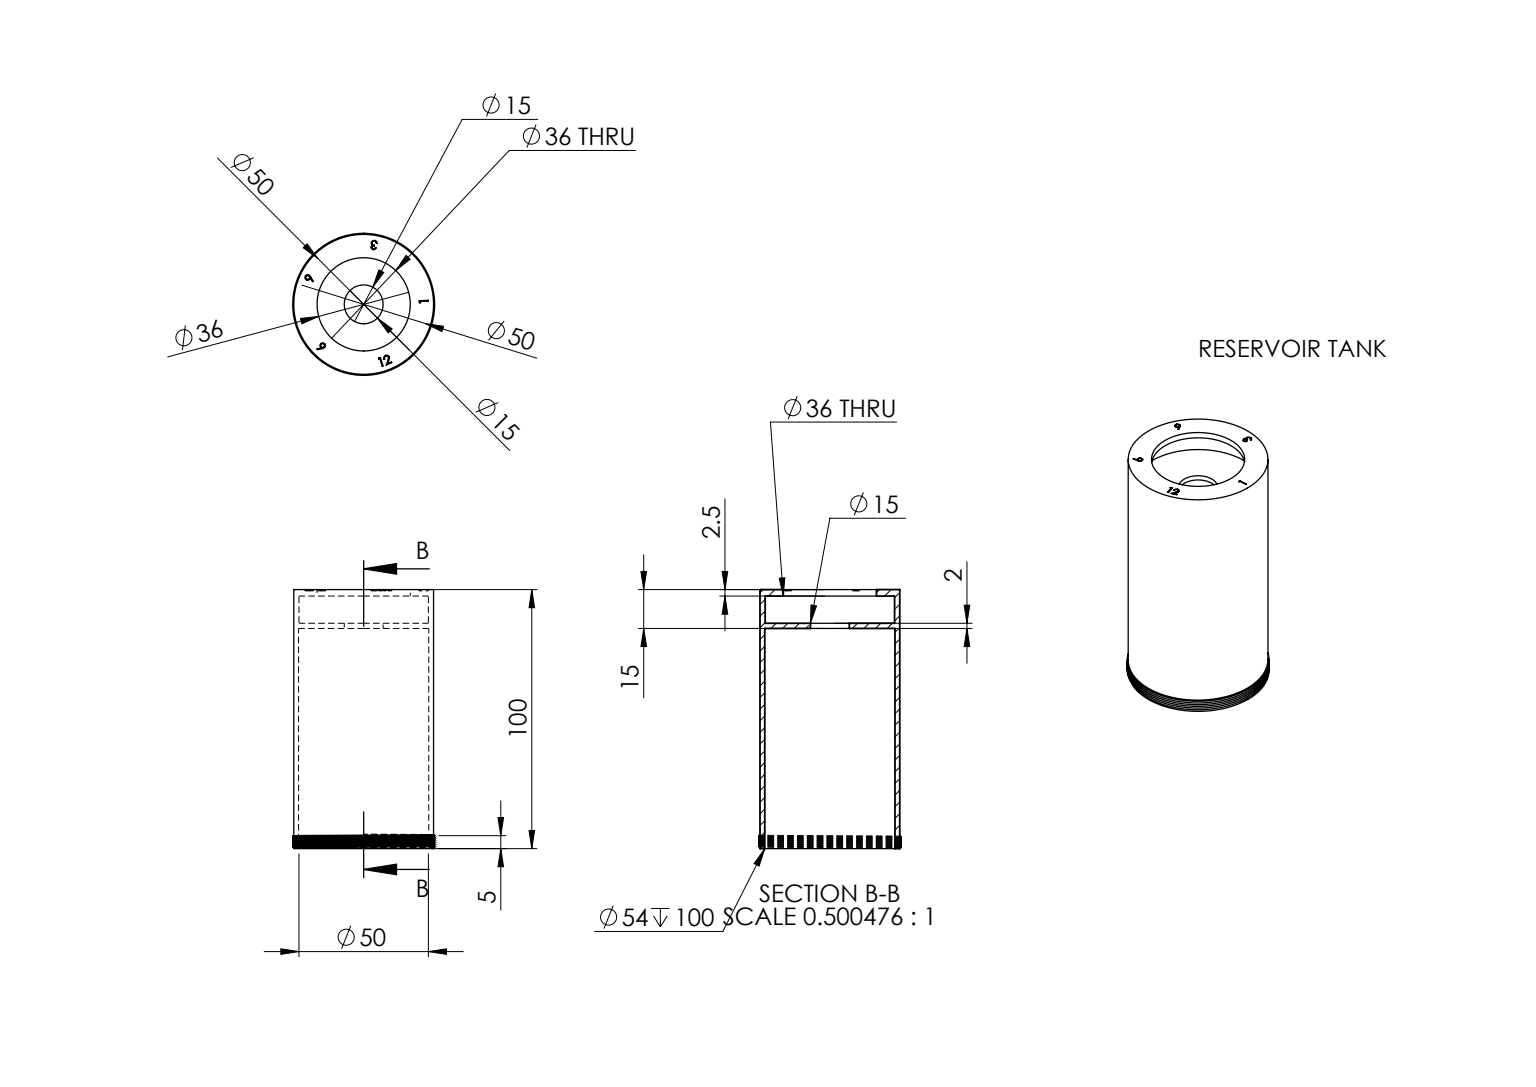
ISO-10303-21;
HEADER;
FILE_DESCRIPTION (('STEP AP214'),
    '1' );
FILE_NAME ('Reservoir Tank.step',
    '2026-10-24T15:06:47',
    ( '' ),
    ( '' ),
    'SwSTEP 2.0',
    'SolidWorks 2026',
    '' );
FILE_SCHEMA (( 'AUTOMOTIVE_DESIGN' ));
ENDSEC;

DATA;
#4=CARTESIAN_POINT ( 'NONE',  ( -22.08823018108446234, 99.50000000000000000, -9.406177930363766038 ) ) ;
#6=EDGE_LOOP ( 'NONE', ( #8139, #8496, #8983, #2392 ) ) ;
#8=CARTESIAN_POINT ( 'NONE',  ( 11.36312591709336850, 1.799999998907525267, 27.43301269999999903 ) ) ;
#9=EDGE_CURVE ( 'NONE', #2280, #2682, #6327, .T. ) ;
#12=ADVANCED_FACE ( 'NONE', ( #17 ), #758, .T. ) ;
#13=CARTESIAN_POINT ( 'NONE',  ( -27.00000000000001421, 4.450000000000000178, 11.18376618407356382 ) ) ;
#14=DIRECTION ( 'NONE',  ( 0.3918949146621865109, 0.000000000000000000, 0.9200099868272720860 ) ) ;
#15=CARTESIAN_POINT ( 'NONE',  ( -21.07742585509981126, 99.49999999999998579, -10.85999754779651383 ) ) ;
#17=FACE_OUTER_BOUND ( 'NONE', #3726, .T. ) ;
#18=CARTESIAN_POINT ( 'NONE',  ( -11.36312591709335962, 2.899999998907525356, -27.43301270000000258 ) ) ;
#19=CARTESIAN_POINT ( 'NONE',  ( 4.295198626299898237, 99.50000000000001421, -24.68029520312135361 ) ) ;
#23=CARTESIAN_POINT ( 'NONE',  ( -22.51767453479306980, 100.0000000000000000, -9.764155749770198511 ) ) ;
#29=CARTESIAN_POINT ( 'NONE',  ( -14.97509118869195888, 99.99999999999998579, 15.26515554624281101 ) ) ;
#35=CARTESIAN_POINT ( 'NONE',  ( -22.31230063665282515, 99.99999999999997158, -10.62159318200525249 ) ) ;
#36=DIRECTION ( 'NONE',  ( 0.000000000000000000, 1.000000000000000000, 0.000000000000000000 ) ) ;
#38=CARTESIAN_POINT ( 'NONE',  ( 27.00000000000000355, 2.999999997815050889, 0.000000000000000000 ) ) ;
#39=CARTESIAN_POINT ( 'NONE',  ( 19.39806930854667399, 3.449999998907525622, 19.39806930854668465 ) ) ;
#41=EDGE_LOOP ( 'NONE', ( #10357, #6514, #2134, #4776 ) ) ;
#43=CARTESIAN_POINT ( 'NONE',  ( 3.739209042966563867, 99.50000000000000000, -21.42288334414699236 ) ) ;
#45=CARTESIAN_POINT ( 'NONE',  ( 3.873456569393397331, 100.0000000000000284, -22.53291374702356364 ) ) ;
#47=CARTESIAN_POINT ( 'NONE',  ( -21.28703419482447146, 99.49999999999997158, -11.01737971290317297 ) ) ;
#48=CARTESIAN_POINT ( 'NONE',  ( 11.36312591709336139, 5.299999998907526155, -27.43301270000000258 ) ) ;
#51=CARTESIAN_POINT ( 'NONE',  ( -15.10382517959271098, 99.49999999999998579, 15.91526905993627317 ) ) ;
#52=DIRECTION ( 'NONE',  ( 0.4750403377899758972, 0.000000000000000000, -0.8799640205556052974 ) ) ;
#56=CARTESIAN_POINT ( 'NONE',  ( 9.910564025336874749, 100.0000000000000142, 20.75459158945058036 ) ) ;
#58=ADVANCED_FACE ( 'NONE', ( #3173 ), #2520, .T. ) ;
#61=CARTESIAN_POINT ( 'NONE',  ( 27.43301270000000258, 1.999999998907524779, -11.36312591709336139 ) ) ;
#63=CARTESIAN_POINT ( 'NONE',  ( 1.679787559701184688E-15, 5.249999998907525445, -27.43301270000000258 ) ) ;
#65=CARTESIAN_POINT ( 'NONE',  ( 11.18376618407356915, 4.950000000000000178, -27.00000000000000355 ) ) ;
#66=FACE_OUTER_BOUND ( 'NONE', #7305, .T. ) ;
#67=CARTESIAN_POINT ( 'NONE',  ( -16.33590634957226229, 99.50000000000000000, 16.80570853669505382 ) ) ;
#68=CARTESIAN_POINT ( 'NONE',  ( -20.91264567078791714, 99.99999999999994316, -10.54226115003387676 ) ) ;
#69=EDGE_CURVE ( 'NONE', #5685, #7937, #6333, .T. ) ;
#70=ORIENTED_EDGE ( 'NONE', *, *, #9652, .T. ) ;
#71=ORIENTED_EDGE ( 'NONE', *, *, #3469, .T. ) ;
#72=CARTESIAN_POINT ( 'NONE',  ( 3.551917533706515417, 100.0000000000000142, -21.11785906961830150 ) ) ;
#73=ORIENTED_EDGE ( 'NONE', *, *, #5083, .F. ) ;
#74=ADVANCED_FACE ( 'NONE', ( #2725 ), #8325, .T. ) ;
#75=CARTESIAN_POINT ( 'NONE',  ( 27.43301269999999548, 4.199999998907525622, 11.36312591709337916 ) ) ;
#76=FACE_OUTER_BOUND ( 'NONE', #1497, .T. ) ;
#81=CARTESIAN_POINT ( 'NONE',  ( -22.63784607493503387, 99.50000000000001421, -10.71517552924587058 ) ) ;
#85=EDGE_CURVE ( 'NONE', #5894, #5272, #1155, .T. ) ;
#86=CARTESIAN_POINT ( 'NONE',  ( 1.653273178848927064E-15, 2.399999997815050357, -27.00000000000000355 ) ) ;
#87=CARTESIAN_POINT ( 'NONE',  ( -20.71654887124055122, 99.50000000000001421, -9.874326132881018125 ) ) ;
#90=B_SPLINE_SURFACE_WITH_KNOTS ( 'NONE', 3, 1, ( 
 ( #3080, #5199 ),
 ( #8397, #1229 ),
 ( #4422, #5539 ),
 ( #1701, #10302 ),
 ( #3282, #3232 ),
 ( #4117, #7200 ),
 ( #3911, #924 ),
 ( #4848, #7097 ),
 ( #4064, #3134 ),
 ( #2291, #2443 ),
 ( #6321, #139 ) ),
 .UNSPECIFIED., .F., .F., .F.,
 ( 4, 1, 1, 1, 1, 1, 1, 1, 4 ),
 ( 2, 2 ),
 ( 0.000000000000000000, 0.09809051273808343241, 0.1997563395654988194, 0.3058527769869914259, 0.4162847437678430240, 0.5377099880548563693, 0.6743560419832976827, 0.8289895874771281425, 1.000000000000000000 ),
 ( 0.000000000000000000, 1.000000000000000000 ),
 .UNSPECIFIED. ) ;
#91=CARTESIAN_POINT ( 'NONE',  ( 3.058419780146050648, 99.50000000000000000, -23.12871267107006545 ) ) ;
#93=AXIS2_PLACEMENT_3D ( 'NONE', #4532, #670, #7729 ) ;
#94=CARTESIAN_POINT ( 'NONE',  ( -15.22320097062094568, 99.50000000000001421, 16.32303119091969634 ) ) ;
#96=CARTESIAN_POINT ( 'NONE',  ( 0.000000000000000000, 100.0000000000000000, 0.000000000000000000 ) ) ;
#97=CARTESIAN_POINT ( 'NONE',  ( 9.245739950628269810, 100.0000000000000284, 20.03726560014620617 ) ) ;
#100=VECTOR ( 'NONE', #6339, 1000.000000000000000 ) ;
#101=CARTESIAN_POINT ( 'NONE',  ( -20.89169796687544789, 100.0000000000000142, -10.40078880447404330 ) ) ;
#105=CARTESIAN_POINT ( 'NONE',  ( 27.43301269999999548, 5.099999998907525978, 11.36312591709337738 ) ) ;
#106=CARTESIAN_POINT ( 'NONE',  ( -15.19031985176477662, 99.49999999999998579, 15.56880617076518547 ) ) ;
#108=CARTESIAN_POINT ( 'NONE',  ( -15.37123125604856710, 99.50000000000001421, 16.48683530611566539 ) ) ;
#111=CARTESIAN_POINT ( 'NONE',  ( 3.970307086022987431, 99.50000000000001421, -24.36314111580913178 ) ) ;
#113=ORIENTED_EDGE ( 'NONE', *, *, #6148, .T. ) ;
#115=CARTESIAN_POINT ( 'NONE',  ( 27.43301270000000258, 1.149999998907525356, 0.000000000000000000 ) ) ;
#118=CARTESIAN_POINT ( 'NONE',  ( -27.43301270000000258, 0.6499999989075253559, -3.359575119402369376E-15 ) ) ;
#120=ORIENTED_EDGE ( 'NONE', *, *, #3091, .T. ) ;
#122=VECTOR ( 'NONE', #1890, 999.9999999999998863 ) ;
#123=CARTESIAN_POINT ( 'NONE',  ( 0.000000000000000000, 99.50000000000000000, 0.000000000000000000 ) ) ;
#124=FACE_OUTER_BOUND ( 'NONE', #10204, .T. ) ;
#128=CARTESIAN_POINT ( 'NONE',  ( 19.39806930854667399, 4.949999998907525622, 19.39806930854668465 ) ) ;
#129=CARTESIAN_POINT ( 'NONE',  ( 3.538198506519217190, 99.99999999999998579, -24.58220198924426114 ) ) ;
#131=CARTESIAN_POINT ( 'NONE',  ( -16.49419651247312046, 99.99999999999998579, 15.57134447358898477 ) ) ;
#132=CARTESIAN_POINT ( 'NONE',  ( -22.69253165798458127, 100.0000000000000142, -10.28928739654909563 ) ) ;
#133=CARTESIAN_POINT ( 'NONE',  ( 4.331079892889020400, 100.0000000000000000, -24.67336562508343079 ) ) ;
#136=ORIENTED_EDGE ( 'NONE', *, *, #3638, .F. ) ;
#137=ORIENTED_EDGE ( 'NONE', *, *, #6348, .F. ) ;
#139=CARTESIAN_POINT ( 'NONE',  ( -16.07368679829020763, 100.0000000000000000, 17.11560437002838952 ) ) ;
#140=CARTESIAN_POINT ( 'NONE',  ( -14.74935495356232984, 100.0000000000000142, 15.91322402822111926 ) ) ;
#142=ADVANCED_FACE ( 'NONE', ( #1039 ), #6680, .T. ) ;
#143=EDGE_CURVE ( 'NONE', #8324, #1908, #2115, .T. ) ;
#148=CARTESIAN_POINT ( 'NONE',  ( -19.09188309203678813, 4.500000000000000888, 19.09188309203678457 ) ) ;
#150=CARTESIAN_POINT ( 'NONE',  ( 3.411785164761435674, 99.50000000000000000, -22.76693382491622231 ) ) ;
#151=CARTESIAN_POINT ( 'NONE',  ( 3.750007936853901658, 99.99999999999998579, -22.95001988029826734 ) ) ;
#152=CARTESIAN_POINT ( 'NONE',  ( 7.856939908706818798, 99.50000000000001421, 20.19612520319305560 ) ) ;
#154=CARTESIAN_POINT ( 'NONE',  ( 27.43301270000000258, 4.349999998907525089, 0.000000000000000000 ) ) ;
#155=CARTESIAN_POINT ( 'NONE',  ( 26.99999999999999645, 3.150000000000000799, 11.18376618407358691 ) ) ;
#156=CARTESIAN_POINT ( 'NONE',  ( -21.24882413972086681, 100.0000000000000284, -9.742484589929601313 ) ) ;
#157=CARTESIAN_POINT ( 'NONE',  ( 3.717146347979291665, 99.50000000000000000, -21.42716062222556417 ) ) ;
#158=CARTESIAN_POINT ( 'NONE',  ( 3.681717055787076642, 99.50000000000000000, -21.09125273517263111 ) ) ;
#162=CARTESIAN_POINT ( 'NONE',  ( -16.01161620991261358, 99.50000000000000000, 17.10240122391520146 ) ) ;
#163=B_SPLINE_CURVE_WITH_KNOTS ( 'NONE', 3,
 ( #932, #5497, #832, #3193, #8885, #3093, #3922, #8786, #6277, #3240, #8737, #729, #9473, #2452, #4752 ),
 .UNSPECIFIED., .F., .F.,
 ( 4, 1, 1, 1, 1, 1, 1, 1, 1, 1, 1, 1, 4 ),
 ( 0.000000000000000000, 0.08490232564366416435, 0.1680779112633816463, 0.2506304657828534177, 0.3338427399641299420, 0.4169763759729993580, 0.4990117930239920674, 0.5811067191809071719, 0.6656374296971073745, 0.7500328835558887075, 0.8331455368193440014, 0.9159638734519762737, 1.000000000000000000 ),
 .UNSPECIFIED. ) ;
#164=CARTESIAN_POINT ( 'NONE',  ( 11.18376618407357626, 3.049999999999999822, 27.00000000000000000 ) ) ;
#165=CARTESIAN_POINT ( 'NONE',  ( 3.373335371007685435, 99.50000000000000000, -22.75111425220066863 ) ) ;
#168=CARTESIAN_POINT ( 'NONE',  ( -21.07742585509981126, 99.99999999999995737, -10.85999754779651383 ) ) ;
#169=ORIENTED_EDGE ( 'NONE', *, *, #6403, .F. ) ;
#174=CARTESIAN_POINT ( 'NONE',  ( 9.404665101723468368, 99.50000000000000000, 20.17141824467128686 ) ) ;
#175=CARTESIAN_POINT ( 'NONE',  ( -16.87593989452418697, 99.49999999999998579, 15.58794934546231126 ) ) ;
#176=CARTESIAN_POINT ( 'NONE',  ( 8.064245308217579122, 99.99999999999998579, 20.64099956338070641 ) ) ;
#179=ORIENTED_EDGE ( 'NONE', *, *, #6506, .T. ) ;
#180=ORIENTED_EDGE ( 'NONE', *, *, #3035, .T. ) ;
#182=CARTESIAN_POINT ( 'NONE',  ( -22.29247428061501779, 99.99999999999997158, -10.66603791136541624 ) ) ;
#183=CARTESIAN_POINT ( 'NONE',  ( 3.611424427577684781, 99.99999999999998579, -21.45475674085064099 ) ) ;
#184=EDGE_CURVE ( 'NONE', #533, #5989, #307, .T. ) ;
#185=CARTESIAN_POINT ( 'NONE',  ( -15.07178375341841381, 100.0000000000000000, 16.66969090848992607 ) ) ;
#187=ORIENTED_EDGE ( 'NONE', *, *, #7681, .T. ) ;
#188=DIRECTION ( 'NONE',  ( 0.000000000000000000, -1.000000000000000000, 0.000000000000000000 ) ) ;
#190=DIRECTION ( 'NONE',  ( -0.05422338932609765960, 0.000000000000000000, -0.9985288298541962204 ) ) ;
#194=ADVANCED_FACE ( 'NONE', ( #1864 ), #9727, .F. ) ;
#195=CARTESIAN_POINT ( 'NONE',  ( 3.302864939465488536, 99.50000000000001421, -22.83905924565489443 ) ) ;
#196=CARTESIAN_POINT ( 'NONE',  ( 3.891852272358404807, 99.99999999999998579, -22.89765557720719968 ) ) ;
#198=EDGE_LOOP ( 'NONE', ( #2371, #2144, #704, #4706 ) ) ;
#199=CARTESIAN_POINT ( 'NONE',  ( 3.207057600658871355, 100.0000000000000284, -22.07913334414698880 ) ) ;
#200=CARTESIAN_POINT ( 'NONE',  ( 27.00000000000000355, 2.999999997815050889, 0.000000000000000000 ) ) ;
#201=CARTESIAN_POINT ( 'NONE',  ( -20.71654887124055122, 100.0000000000000142, -9.874326132881018125 ) ) ;
#202=CARTESIAN_POINT ( 'NONE',  ( -21.66466628782423243, 100.0000000000000142, -9.640935998098070669 ) ) ;
#203=LINE ( 'NONE', #3388, #8398 ) ;
#205=LINE ( 'NONE', #1725, #6091 ) ;
#207=ORIENTED_EDGE ( 'NONE', *, *, #9006, .F. ) ;
#209=FACE_OUTER_BOUND ( 'NONE', #3870, .T. ) ;
#210=CARTESIAN_POINT ( 'NONE',  ( 9.806436918512124734, 99.99999999999998579, 20.18080982695387604 ) ) ;
#212=CARTESIAN_POINT ( 'NONE',  ( -27.43301270000000258, 2.199999998907525622, -11.36312591709336317 ) ) ;
#214=DIRECTION ( 'NONE',  ( -0.000000000000000000, 1.000000000000000000, -0.000000000000000000 ) ) ;
#215=CARTESIAN_POINT ( 'NONE',  ( 8.429066232339796017, 100.0000000000000000, 19.67794530653910101 ) ) ;
#216=CARTESIAN_POINT ( 'NONE',  ( 1.653273178848927064E-15, 2.399999997815050357, -27.00000000000000355 ) ) ;
#217=ORIENTED_EDGE ( 'NONE', *, *, #7917, .F. ) ;
#218=CARTESIAN_POINT ( 'NONE',  ( -20.89052720883767122, 99.50000000000000000, -9.602653601535816819 ) ) ;
#219=CARTESIAN_POINT ( 'NONE',  ( 11.36312591709336139, 5.199999998907525622, -27.43301270000000258 ) ) ;
#220=CARTESIAN_POINT ( 'NONE',  ( -16.18965924272485779, 99.49999999999998579, 15.26525457555968224 ) ) ;
#221=FACE_OUTER_BOUND ( 'NONE', #8631, .T. ) ;
#223=CARTESIAN_POINT ( 'NONE',  ( 26.99999999999999645, 1.550000000000000266, 11.18376618407358691 ) ) ;
#224=VERTEX_POINT ( 'NONE', #1816 ) ;
#225=CARTESIAN_POINT ( 'NONE',  ( 5.240996349771887886, 100.0000000000000142, -23.60769396873743631 ) ) ;
#226=ORIENTED_EDGE ( 'NONE', *, *, #3625, .T. ) ;
#227=EDGE_CURVE ( 'NONE', #6767, #4694, #1090, .T. ) ;
#231=LINE ( 'NONE', #3414, #2289 ) ;
#232=LINE ( 'NONE', #8144, #5785 ) ;
#233=CARTESIAN_POINT ( 'NONE',  ( -22.11394672483139701, 99.50000000000000000, -10.91855052283267646 ) ) ;
#235=CARTESIAN_POINT ( 'NONE',  ( -15.26676860252058887, 99.99999999999998579, 16.38168943497750973 ) ) ;
#236=VECTOR ( 'NONE', #2101, 1000.000000000000000 ) ;
#237=EDGE_CURVE ( 'NONE', #1790, #7639, #6949, .T. ) ;
#240=CARTESIAN_POINT ( 'NONE',  ( 0.000000000000000000, 97.50000000000000000, 18.00000000000000000 ) ) ;
#242=CARTESIAN_POINT ( 'NONE',  ( 3.058419780146050648, 99.50000000000000000, -23.12871267107006545 ) ) ;
#243=LINE ( 'NONE', #5946, #5211 ) ;
#244=CARTESIAN_POINT ( 'NONE',  ( 3.701176614148623756, 99.50000000000000000, -24.64875008328975170 ) ) ;
#245=CARTESIAN_POINT ( 'NONE',  ( 7.734522023158566739, 99.50000000000002842, 20.86022014488863618 ) ) ;
#248=CARTESIAN_POINT ( 'NONE',  ( 1.653273178848927064E-15, 4.799999997815051600, -27.00000000000000355 ) ) ;
#249=CARTESIAN_POINT ( 'NONE',  ( -21.00001322343447541, 99.50000000000001421, -9.990026185521596602 ) ) ;
#250=CARTESIAN_POINT ( 'NONE',  ( 3.635130212803377781, 100.0000000000000000, -23.00575896550913768 ) ) ;
#251=CARTESIAN_POINT ( 'NONE',  ( -21.72555844818415594, 99.50000000000001421, -11.09629251537910655 ) ) ;
#252=CARTESIAN_POINT ( 'NONE',  ( 4.906732565843439531, 100.0000000000000142, -23.57187248890526376 ) ) ;
#255=B_SPLINE_CURVE_WITH_KNOTS ( 'NONE', 3,
 ( #43, #4128, #5748, #6482, #981, #3244, #8984, #8105, #7258, #4950, #7354, #5651, #9812, #9671, #7311 ),
 .UNSPECIFIED., .F., .F.,
 ( 4, 1, 1, 1, 1, 1, 1, 1, 1, 1, 1, 1, 4 ),
 ( 0.000000000000000000, 0.1166921615859537187, 0.2277195327244859735, 0.3361971884410420164, 0.4453256767247914527, 0.5018483577356800396, 0.5617326728321133666, 0.6243107931132723110, 0.6909729641497043273, 0.7615676753376537933, 0.8363829297815326136, 0.9156607463298391814, 0.9999999999999998890 ),
 .UNSPECIFIED. ) ;
#258=CARTESIAN_POINT ( 'NONE',  ( -15.03963071504896121, 100.0000000000000000, 16.63526396357264758 ) ) ;
#261=CARTESIAN_POINT ( 'NONE',  ( 27.43301270000000258, 1.849999998907525534, 0.000000000000000000 ) ) ;
#264=CARTESIAN_POINT ( 'NONE',  ( -20.64578974631102426, 99.99999999999995737, -10.10077944494247504 ) ) ;
#265=DIRECTION ( 'NONE',  ( -0.000000000000000000, 1.000000000000000000, -0.000000000000000000 ) ) ;
#266=CARTESIAN_POINT ( 'NONE',  ( 8.322475189980043098, 100.0000000000000142, 19.72675386960232657 ) ) ;
#267=ORIENTED_EDGE ( 'NONE', *, *, #2370, .F. ) ;
#268=CARTESIAN_POINT ( 'NONE',  ( -21.30033281797529909, 99.50000000000002842, -9.345151174687854834 ) ) ;
#269=CARTESIAN_POINT ( 'NONE',  ( 4.135809822336132591, 99.99999999999998579, -24.70305975188825443 ) ) ;
#271=CARTESIAN_POINT ( 'NONE',  ( 3.775125937424839151, 100.0000000000000000, -21.41825520325024712 ) ) ;
#272=CARTESIAN_POINT ( 'NONE',  ( 8.829292973371666520, 99.49999999999998579, 19.92220432019063736 ) ) ;
#278=ORIENTED_EDGE ( 'NONE', *, *, #3961, .T. ) ;
#279=VECTOR ( 'NONE', #5092, 1000.000000000000000 ) ;
#281=CARTESIAN_POINT ( 'NONE',  ( 6.246869686064662197, 99.50000000000000000, 20.92172973853146090 ) ) ;
#282=CARTESIAN_POINT ( 'NONE',  ( 1.653273178848927064E-15, 4.799999997815051600, -27.00000000000000355 ) ) ;
#285=CARTESIAN_POINT ( 'NONE',  ( 8.081885929396888102, 99.50000000000001421, 20.89785832093561169 ) ) ;
#286=CARTESIAN_POINT ( 'NONE',  ( 2.852289972453743161, 99.50000000000000000, -22.14293542748032451 ) ) ;
#288=CARTESIAN_POINT ( 'NONE',  ( 3.735769352376668184, 99.49999999999998579, -24.30643046864489420 ) ) ;
#292=CARTESIAN_POINT ( 'NONE',  ( -27.43301270000000258, 3.949999998907525178, -3.359575119402369376E-15 ) ) ;
#294=EDGE_CURVE ( 'NONE', #8788, #5320, #3852, .T. ) ;
#296=DIRECTION ( 'NONE',  ( -0.000000000000000000, -1.000000000000000000, -0.000000000000000000 ) ) ;
#297=CARTESIAN_POINT ( 'NONE',  ( 7.771508748547515388, 99.50000000000001421, 20.40818475981234315 ) ) ;
#298=ORIENTED_EDGE ( 'NONE', *, *, #7410, .F. ) ;
#299=CARTESIAN_POINT ( 'NONE',  ( 9.902568905804752575, 99.49999999999998579, 20.48863403721516363 ) ) ;
#300=CARTESIAN_POINT ( 'NONE',  ( -11.18376618407356560, 3.249999997815050001, -27.00000000000000355 ) ) ;
#301=CARTESIAN_POINT ( 'NONE',  ( -21.16695614262292580, 99.50000000000000000, -11.33496398805607441 ) ) ;
#304=CARTESIAN_POINT ( 'NONE',  ( -21.44539290152690114, 100.0000000000000000, -11.08070480119962298 ) ) ;
#306=PLANE ( 'NONE',  #2619 ) ;
#307=LINE ( 'NONE', #5759, #1112 ) ;
#313=CARTESIAN_POINT ( 'NONE',  ( -11.36312591709335962, 2.099999998907525089, -27.43301270000000258 ) ) ;
#314=CARTESIAN_POINT ( 'NONE',  ( -11.18376618407358336, 0.5500000000000000444, 26.99999999999999645 ) ) ;
#315=CARTESIAN_POINT ( 'NONE',  ( 7.826802610544922878, 99.50000000000000000, 21.21129867192371421 ) ) ;
#316=FACE_BOUND ( 'NONE', #7653, .T. ) ;
#318=CARTESIAN_POINT ( 'NONE',  ( 8.133363296361027395, 99.50000000000004263, 19.85287606700953233 ) ) ;
#319=EDGE_CURVE ( 'NONE', #4075, #2239, #1707, .T. ) ;
#320=CARTESIAN_POINT ( 'NONE',  ( 3.538198506519217190, 99.99999999999998579, -24.58220198924426114 ) ) ;
#321=CARTESIAN_POINT ( 'NONE',  ( 27.43301270000000258, 0.2499999989075251949, 0.000000000000000000 ) ) ;
#322=EDGE_CURVE ( 'NONE', #8484, #8640, #4914, .T. ) ;
#324=LINE ( 'NONE', #3511, #9225 ) ;
#325=CARTESIAN_POINT ( 'NONE',  ( 3.341734429721257005, 99.50000000000000000, -22.34498040423979148 ) ) ;
#326=CARTESIAN_POINT ( 'NONE',  ( -21.52330660073277002, 100.0000000000000142, -9.647028226243550719 ) ) ;
#327=ORIENTED_EDGE ( 'NONE', *, *, #2893, .T. ) ;
#328=LINE ( 'NONE', #4461, #9892 ) ;
#330=ORIENTED_EDGE ( 'NONE', *, *, #8122, .T. ) ;
#331=CARTESIAN_POINT ( 'NONE',  ( -22.57971655928959365, 100.0000000000000000, -10.84768434062017839 ) ) ;
#332=CARTESIAN_POINT ( 'NONE',  ( 3.739209042966563867, 99.50000000000000000, -21.42288334414699236 ) ) ;
#333=CARTESIAN_POINT ( 'NONE',  ( 3.635130212803377781, 99.50000000000000000, -23.00575896550913768 ) ) ;
#334=CARTESIAN_POINT ( 'NONE',  ( -15.30066472929571653, 99.99999999999998579, 16.41738810589640707 ) ) ;
#335=ORIENTED_EDGE ( 'NONE', *, *, #10100, .T. ) ;
#336=EDGE_LOOP ( 'NONE', ( #9504, #8678, #3054, #1608, #4599, #7689 ) ) ;
#337=CARTESIAN_POINT ( 'NONE',  ( -16.54770463920453949, 99.99999999999998579, 15.70234036036222847 ) ) ;
#339=CARTESIAN_POINT ( 'NONE',  ( -21.86704275050744073, 100.0000000000000142, -11.06111336656620026 ) ) ;
#340=DIRECTION ( 'NONE',  ( 0.000000000000000000, -0.000000000000000000, 1.000000000000000000 ) ) ;
#341=VERTEX_POINT ( 'NONE', #9434 ) ;
#343=CARTESIAN_POINT ( 'NONE',  ( 11.36312591709336850, 2.599999998907525534, 27.43301269999999903 ) ) ;
#345=CARTESIAN_POINT ( 'NONE',  ( 4.154273145530666511, 99.50000000000000000, -22.82723029927519676 ) ) ;
#346=CARTESIAN_POINT ( 'NONE',  ( 7.783718120363267268, 99.49999999999998579, 21.09473326129887027 ) ) ;
#347=CARTESIAN_POINT ( 'NONE',  ( 3.298672054714395063, 99.50000000000001421, -22.72039518595936869 ) ) ;
#348=CARTESIAN_POINT ( 'NONE',  ( -11.18376618407358336, 5.149999997815050357, 26.99999999999999645 ) ) ;
#349=CARTESIAN_POINT ( 'NONE',  ( 0.000000000000000000, 87.00000000000001421, -7.500000000000000000 ) ) ;
#351=CARTESIAN_POINT ( 'NONE',  ( -21.45221949983897858, 99.50000000000000000, -9.661157428473494235 ) ) ;
#355=CARTESIAN_POINT ( 'NONE',  ( 3.311778287470797721, 100.0000000000000000, -21.22295334266859967 ) ) ;
#356=VECTOR ( 'NONE', #6599, 1000.000000000000000 ) ;
#358=VERTEX_POINT ( 'NONE', #2092 ) ;
#361=CARTESIAN_POINT ( 'NONE',  ( -14.97509118869195888, 99.99999999999997158, 15.26515554624281101 ) ) ;
#362=CARTESIAN_POINT ( 'NONE',  ( 2.940631318607589417, 100.0000000000000000, -23.77584808773673331 ) ) ;
#363=CARTESIAN_POINT ( 'NONE',  ( 19.39806930854668110, 2.749999998907525001, -19.39806930854668110 ) ) ;
#366=FACE_OUTER_BOUND ( 'NONE', #5178, .T. ) ;
#367=LINE ( 'NONE', #3559, #9996 ) ;
#368=EDGE_CURVE ( 'NONE', #3042, #1114, #439, .T. ) ;
#369=VERTEX_POINT ( 'NONE', #584 ) ;
#370=CARTESIAN_POINT ( 'NONE',  ( -20.82968571475833031, 99.50000000000001421, -9.677916414284339908 ) ) ;
#371=CARTESIAN_POINT ( 'NONE',  ( 3.028692941384139026, 100.0000000000000142, -22.52214499033115302 ) ) ;
#373=CARTESIAN_POINT ( 'NONE',  ( 11.36312591709336139, 0.3999999989075252449, -27.43301270000000258 ) ) ;
#374=( NAMED_UNIT ( * ) SI_UNIT ( $, .STERADIAN. ) SOLID_ANGLE_UNIT ( ) );
#375=CARTESIAN_POINT ( 'NONE',  ( 9.431378708427812896, 99.49999999999998579, 21.34379071326255684 ) ) ;
#378=CARTESIAN_POINT ( 'NONE',  ( -16.18394139941567644, 99.50000000000000000, 16.57042731130403723 ) ) ;
#380=VECTOR ( 'NONE', #9183, 1000.000000000000000 ) ;
#383=CARTESIAN_POINT ( 'NONE',  ( -22.17094027205346052, 99.99999999999998579, -9.884352203306939089 ) ) ;
#385=EDGE_CURVE ( 'NONE', #2107, #6279, #9699, .T. ) ;
#388=CARTESIAN_POINT ( 'NONE',  ( 1.653273178848927064E-15, 2.600000000000000533, -27.00000000000000355 ) ) ;
#389=ADVANCED_FACE ( 'NONE', ( #532 ), #7015, .T. ) ;
#390=CARTESIAN_POINT ( 'NONE',  ( 4.743081672682207817, 99.50000000000002842, -21.60795120912350598 ) ) ;
#392=CARTESIAN_POINT ( 'NONE',  ( 3.888553205800344248, 99.49999999999995737, -24.35333287445124739 ) ) ;
#393=VERTEX_POINT ( 'NONE', #3617 ) ;
#394=B_SPLINE_CURVE_WITH_KNOTS ( 'NONE', 3,
 ( #7553, #5714, #8244, #9861, #7500, #8345, #4874, #1176, #4367, #3255, #8064, #8626, #6935, #2911, #8453 ),
 .UNSPECIFIED., .F., .F.,
 ( 4, 1, 1, 1, 1, 1, 1, 1, 1, 1, 1, 1, 4 ),
 ( 0.000000000000000000, 0.1101401978779246588, 0.2116695470404897084, 0.3047824012491699430, 0.3893374185178356539, 0.4648567744508144695, 0.5325800579573772842, 0.5913915682020929321, 0.6424829260185016544, 0.7344861914544180692, 0.8232371011010507500, 0.9113455750355911045, 1.000000000000000000 ),
 .UNSPECIFIED. ) ;
#395=CARTESIAN_POINT ( 'NONE',  ( 2.204364238465235428E-15, 97.50000000000000000, -18.00000000000000000 ) ) ;
#396=CARTESIAN_POINT ( 'NONE',  ( 19.39806930854667399, 2.649999998907525356, 19.39806930854668465 ) ) ;
#398=CARTESIAN_POINT ( 'NONE',  ( 9.838488147574068421, 99.99999999999998579, 20.25735696016189280 ) ) ;
#399=CARTESIAN_POINT ( 'NONE',  ( 4.320351800798612807, 99.99999999999994316, -21.62386382141117736 ) ) ;
#401=CARTESIAN_POINT ( 'NONE',  ( 2.912748042341355870, 99.49999999999998579, -22.34826719014139940 ) ) ;
#402=CARTESIAN_POINT ( 'NONE',  ( 1.653273178848927064E-15, 3.199999997815050623, -27.00000000000000355 ) ) ;
#403=PLANE ( 'NONE',  #1653 ) ;
#405=VERTEX_POINT ( 'NONE', #6179 ) ;
#406=CARTESIAN_POINT ( 'NONE',  ( 4.852629679480013891, 100.0000000000000142, -23.84752007312514621 ) ) ;
#408=CARTESIAN_POINT ( 'NONE',  ( 11.36312591709336850, 1.799999998907525045, 27.43301269999999903 ) ) ;
#412=PLANE ( 'NONE',  #3273 ) ;
#414=CARTESIAN_POINT ( 'NONE',  ( -19.39806930854667755, 2.149999998907525356, -19.39806930854668110 ) ) ;
#415=CARTESIAN_POINT ( 'NONE',  ( -20.42657152723830905, 100.0000000000000000, -10.54129411626120216 ) ) ;
#417=CARTESIAN_POINT ( 'NONE',  ( -15.33577160963320374, 99.99999999999998579, 16.45272793336155814 ) ) ;
#419=DIRECTION ( 'NONE',  ( 0.2499845035238856816, 0.000000000000000000, -0.9682498375925071565 ) ) ;
#420=AXIS2_PLACEMENT_3D ( 'NONE', #8279, #1213, #4351 ) ;
#421=CARTESIAN_POINT ( 'NONE',  ( 3.386276725104728769, 100.0000000000000142, -24.01678749451497907 ) ) ;
#422=CARTESIAN_POINT ( 'NONE',  ( 8.051038018032482313, 99.49999999999998579, 19.92675698219059299 ) ) ;
#423=CARTESIAN_POINT ( 'NONE',  ( 4.820889542125314620, 99.99999999999998579, -21.76289454767624676 ) ) ;
#424=ORIENTED_EDGE ( 'NONE', *, *, #8874, .F. ) ;
#426=CARTESIAN_POINT ( 'NONE',  ( -16.12578516900833137, 99.50000000000001421, 15.23469143358620492 ) ) ;
#427=CARTESIAN_POINT ( 'NONE',  ( -16.38049141020750099, 100.0000000000000000, 14.97568473612765416 ) ) ;
#428=EDGE_CURVE ( 'NONE', #5950, #1908, #2150, .T. ) ;
#429=CARTESIAN_POINT ( 'NONE',  ( 4.061806280070601183, 99.50000000000001421, -22.51960061163626392 ) ) ;
#430=CARTESIAN_POINT ( 'NONE',  ( 27.00000000000000355, 2.400000000000000355, 0.000000000000000000 ) ) ;
#432=CARTESIAN_POINT ( 'NONE',  ( 4.909381318607588973, 100.0000000000000000, -23.54377677363417121 ) ) ;
#434=ORIENTED_EDGE ( 'NONE', *, *, #1477, .F. ) ;
#435=FACE_OUTER_BOUND ( 'NONE', #1717, .T. ) ;
#436=CARTESIAN_POINT ( 'NONE',  ( -20.72805389903318130, 99.50000000000000000, -9.848585782927868237 ) ) ;
#437=CARTESIAN_POINT ( 'NONE',  ( -27.00000000000000355, 4.999999997815050889, -3.306546357697854128E-15 ) ) ;
#438=CARTESIAN_POINT ( 'NONE',  ( 4.503533123526070270, 99.49999999999995737, -24.63026223303895890 ) ) ;
#439=B_SPLINE_CURVE_WITH_KNOTS ( 'NONE', 3,
 ( #8599, #10219, #1422, #6016, #9260, #5228, #8483, #10166, #2941, #2262, #6851, #4611, #3777, #7803, #634, #1312, #2033, #10047, #6122 ),
 .UNSPECIFIED., .F., .F.,
 ( 4, 1, 1, 1, 1, 1, 1, 1, 1, 1, 1, 1, 1, 1, 1, 1, 4 ),
 ( 0.000000000000000000, 0.06485467887857676583, 0.1277145915909605745, 0.1892127134908106190, 0.2497332716026948729, 0.3109554005383074471, 0.3726238983726959941, 0.4350931267523188151, 0.5000867325104639827, 0.5644742510850394579, 0.6276292343746815439, 0.6888483565510189477, 0.7500704854866314664, 0.8105910435985150819, 0.8724026516570742018, 0.9351453211214243444, 1.000000000000000000 ),
 .UNSPECIFIED. ) ;
#441=CARTESIAN_POINT ( 'NONE',  ( 4.433602057339688152, 99.50000000000000000, -21.25644978738549540 ) ) ;
#442=CARTESIAN_POINT ( 'NONE',  ( -16.60513711880302878, 100.0000000000000000, 15.15667007515659570 ) ) ;
#443=CYLINDRICAL_SURFACE ( 'NONE', #7131, 27.00000000000000355 ) ;
#444=ORIENTED_EDGE ( 'NONE', *, *, #143, .F. ) ;
#445=EDGE_CURVE ( 'NONE', #9406, #8902, #446, .T. ) ;
#446=CIRCLE ( 'NONE', #7814, 25.00000000000000000 ) ;
#448=CARTESIAN_POINT ( 'NONE',  ( 27.43301269999999548, 3.499999998907525445, 11.36312591709337738 ) ) ;
#449=CARTESIAN_POINT ( 'NONE',  ( 5.243816414761435674, 99.50000000000000000, -23.48558366465980995 ) ) ;
#454=ORIENTED_EDGE ( 'NONE', *, *, #9048, .F. ) ;
#456=CARTESIAN_POINT ( 'NONE',  ( 9.164845778125666698, 100.0000000000000142, 19.62003801130714820 ) ) ;
#458=CARTESIAN_POINT ( 'NONE',  ( 0.000000000000000000, 100.0000000000000000, 0.000000000000000000 ) ) ;
#460=ORIENTED_EDGE ( 'NONE', *, *, #1580, .F. ) ;
#461=CARTESIAN_POINT ( 'NONE',  ( -16.33590634957226229, 100.0000000000000000, 16.80570853669505382 ) ) ;
#462=CARTESIAN_POINT ( 'NONE',  ( -19.39806930854667755, 0.6499999989075252449, -19.39806930854668110 ) ) ;
#463=VERTEX_POINT ( 'NONE', #796 ) ;
#464=AXIS2_PLACEMENT_3D ( 'NONE', #123, #8026, #3312 ) ;
#467=CARTESIAN_POINT ( 'NONE',  ( 2.955068081869620666, 99.49999999999998579, -21.57801138750623338 ) ) ;
#470=CARTESIAN_POINT ( 'NONE',  ( 11.36312591709336850, 1.799999998907525267, 27.43301269999999903 ) ) ;
#472=CARTESIAN_POINT ( 'NONE',  ( 9.263267005978743640, 99.99999999999998579, 19.65676951151765905 ) ) ;
#473=VECTOR ( 'NONE', #4523, 1000.000000000000000 ) ;
#474=CARTESIAN_POINT ( 'NONE',  ( 4.232798786556307036, 99.50000000000000000, -24.34936571594186105 ) ) ;
#475=CARTESIAN_POINT ( 'NONE',  ( -4.959819536546781389E-15, 4.399999997815050357, 27.00000000000000355 ) ) ;
#476=DIRECTION ( 'NONE',  ( 0.000000000000000000, 1.000000000000000000, 0.000000000000000000 ) ) ;
#479=ORIENTED_EDGE ( 'NONE', *, *, #7743, .T. ) ;
#481=CARTESIAN_POINT ( 'NONE',  ( -11.36312591709335962, 1.299999998907525267, -27.43301270000000258 ) ) ;
#483=LINE ( 'NONE', #1481, #1244 ) ;
#484=CARTESIAN_POINT ( 'NONE',  ( 9.575551604960836016, 99.99999999999994316, 20.57049984249936969 ) ) ;
#485=CARTESIAN_POINT ( 'NONE',  ( 19.09188309203678813, 2.500000000000000000, -19.09188309203678813 ) ) ;
#488=CARTESIAN_POINT ( 'NONE',  ( -16.18394139941567644, 100.0000000000000000, 16.57042731130403723 ) ) ;
#490=ORIENTED_EDGE ( 'NONE', *, *, #6754, .F. ) ;
#491=ADVANCED_FACE ( 'NONE', ( #8851 ), #8702, .T. ) ;
#493=CARTESIAN_POINT ( 'NONE',  ( -4.959819536546781389E-15, 3.799999999999999822, 27.00000000000000355 ) ) ;
#495=B_SPLINE_SURFACE_WITH_KNOTS ( 'NONE', 3, 1, ( 
 ( #5925, #4898 ),
 ( #8143, #182 ),
 ( #1700, #1889 ),
 ( #8094, #5877 ),
 ( #6609, #8234 ),
 ( #9706, #1065 ),
 ( #5084, #6562 ),
 ( #9753, #8284 ),
 ( #5780, #5245 ),
 ( #6869, #8337 ),
 ( #4358, #6086 ),
 ( #5981, #5304 ),
 ( #8443, #2846 ),
 ( #2794, #383 ),
 ( #4518, #9278 ),
 ( #2902, #1273 ),
 ( #3576, #4464 ),
 ( #6031, #9959 ),
 ( #1167, #10065 ) ),
 .UNSPECIFIED., .F., .F., .F.,
 ( 4, 1, 1, 1, 1, 1, 1, 1, 1, 1, 1, 1, 1, 1, 1, 1, 4 ),
 ( 2, 2 ),
 ( 0.000000000000000000, 0.06441145199513656494, 0.1272798026707614161, 0.1891796676955485867, 0.2501048626594916668, 0.3106574229659737063, 0.3727353219478334867, 0.4357106927796215445, 0.5001540812204312569, 0.5646670943021733224, 0.6273118991093056263, 0.6892359343283066542, 0.7500873997029591234, 0.8110709007071082999, 0.8723115105649058565, 0.9354174373376444862, 1.000000000000000000 ),
 ( 0.000000000000000000, 1.000000000000000000 ),
 .UNSPECIFIED. ) ;
#496=CARTESIAN_POINT ( 'NONE',  ( 2.204364238465235428E-15, 97.50000000000000000, -18.00000000000000000 ) ) ;
#497=CARTESIAN_POINT ( 'NONE',  ( 5.142436925601051811, 99.99999999999998579, -24.04117066426968563 ) ) ;
#498=VERTEX_POINT ( 'NONE', #3936 ) ;
#499=CARTESIAN_POINT ( 'NONE',  ( 1.679787559701184688E-15, 5.249999998907525445, -27.43301270000000258 ) ) ;
#501=CARTESIAN_POINT ( 'NONE',  ( -11.18376618407358336, 1.350000000000000089, 26.99999999999999645 ) ) ;
#503=ORIENTED_EDGE ( 'NONE', *, *, #227, .F. ) ;
#505=CARTESIAN_POINT ( 'NONE',  ( -5.039362679103552881E-15, 2.549999998907525267, 27.43301270000000258 ) ) ;
#507=DIRECTION ( 'NONE',  ( 0.2041339490496966447, 0.000000000000000000, 0.9789429660840186509 ) ) ;
#508=ORIENTED_EDGE ( 'NONE', *, *, #6395, .T. ) ;
#509=PLANE ( 'NONE',  #2435 ) ;
#511=CARTESIAN_POINT ( 'NONE',  ( 10.85214315541671759, 99.50000000000000000, 22.51047735782115211 ) ) ;
#514=FACE_BOUND ( 'NONE', #4676, .T. ) ;
#517=CARTESIAN_POINT ( 'NONE',  ( -15.62751930918662069, 99.99999999999998579, 15.20915780906945436 ) ) ;
#518=CARTESIAN_POINT ( 'NONE',  ( 11.36312591709336139, 1.299999998907525267, -27.43301270000000258 ) ) ;
#519=VERTEX_POINT ( 'NONE', #3988 ) ;
#521=EDGE_CURVE ( 'NONE', #9655, #8484, #10339, .T. ) ;
#522=PRODUCT_CONTEXT ( 'NONE', #6203, 'mechanical' ) ;
#523=CARTESIAN_POINT ( 'NONE',  ( -22.08823018108446234, 99.50000000000000000, -9.406177930363766038 ) ) ;
#526=CARTESIAN_POINT ( 'NONE',  ( 4.901590909071964042, 99.50000000000000000, -23.62641080846013608 ) ) ;
#527=CARTESIAN_POINT ( 'NONE',  ( -11.36312591709337383, 2.499999998907525445, 27.43301269999999548 ) ) ;
#528=DIRECTION ( 'NONE',  ( 0.5074415416931677969, 0.000000000000000000, 0.8616861851997287269 ) ) ;
#530=CARTESIAN_POINT ( 'NONE',  ( -16.33590634957226229, 99.50000000000000000, 16.80570853669505382 ) ) ;
#531=EDGE_CURVE ( 'NONE', #4569, #6174, #2823, .T. ) ;
#532=FACE_OUTER_BOUND ( 'NONE', #9383, .T. ) ;
#533=VERTEX_POINT ( 'NONE', #1473 ) ;
#535=CARTESIAN_POINT ( 'NONE',  ( -21.71039561923405969, 99.50000000000004263, -11.44438725057713313 ) ) ;
#537=CARTESIAN_POINT ( 'NONE',  ( 0.000000000000000000, 100.0000000000000000, -27.00000000000000355 ) ) ;
#538=CARTESIAN_POINT ( 'NONE',  ( 27.43301270000000258, 3.449999998907525178, 0.000000000000000000 ) ) ;
#540=CARTESIAN_POINT ( 'NONE',  ( -15.17782247516205274, 99.99999999999994316, 15.06300032623928686 ) ) ;
#541=CARTESIAN_POINT ( 'NONE',  ( 11.18376618407357626, 0.6500000000000001332, 27.00000000000000000 ) ) ;
#542=CARTESIAN_POINT ( 'NONE',  ( 8.973011566395204142, 100.0000000000000000, 19.93291184930431115 ) ) ;
#543=ORIENTED_EDGE ( 'NONE', *, *, #85, .T. ) ;
#544=CARTESIAN_POINT ( 'NONE',  ( 4.773458297025112707, 100.0000000000000142, -24.02094923175124208 ) ) ;
#546=ORIENTED_EDGE ( 'NONE', *, *, #9397, .T. ) ;
#547=VECTOR ( 'NONE', #4546, 1000.000000000000114 ) ;
#548=CARTESIAN_POINT ( 'NONE',  ( 27.43301270000000258, 0.3499999989075252005, 0.000000000000000000 ) ) ;
#549=CARTESIAN_POINT ( 'NONE',  ( -15.15193744131588183, 100.0000000000000142, 16.74589488344418697 ) ) ;
#550=CARTESIAN_POINT ( 'NONE',  ( 8.685676809262872666, 99.50000000000000000, 23.43455588346217766 ) ) ;
#552=CARTESIAN_POINT ( 'NONE',  ( -4.959819536546781389E-15, 3.799999999999999822, 27.00000000000000355 ) ) ;
#557=ORIENTED_EDGE ( 'NONE', *, *, #10190, .F. ) ;
#558=CARTESIAN_POINT ( 'NONE',  ( -22.51488550592518934, 99.99999999999997158, -10.97145172607810615 ) ) ;
#561=CARTESIAN_POINT ( 'NONE',  ( 9.820792995160310568, 100.0000000000000000, 20.21220011423141116 ) ) ;
#563=EDGE_LOOP ( 'NONE', ( #712, #7124, #2211 ) ) ;
#565=CARTESIAN_POINT ( 'NONE',  ( 4.154273145530666511, 99.50000000000000000, -22.82723029927519676 ) ) ;
#566=FACE_OUTER_BOUND ( 'NONE', #1534, .T. ) ;
#567=ORIENTED_EDGE ( 'NONE', *, *, #4419, .F. ) ;
#569=CARTESIAN_POINT ( 'NONE',  ( 27.43301269999999548, 1.899999998907525356, 11.36312591709337916 ) ) ;
#573=CARTESIAN_POINT ( 'NONE',  ( 4.835062408351179286, 99.50000000000000000, -21.79588013901878440 ) ) ;
#574=CARTESIAN_POINT ( 'NONE',  ( 2.864934851235464208, 99.99999999999997158, -21.80148171563692827 ) ) ;
#577=CARTESIAN_POINT ( 'NONE',  ( 1.653273178848927064E-15, 3.199999997815050623, -27.00000000000000355 ) ) ;
#578=CARTESIAN_POINT ( 'NONE',  ( 11.36312591709336850, 3.399999998907525356, 27.43301269999999903 ) ) ;
#579=FACE_OUTER_BOUND ( 'NONE', #8185, .T. ) ;
#583=B_SPLINE_SURFACE_WITH_KNOTS ( 'NONE', 3, 1, ( 
 ( #4695, #1499 ),
 ( #4063, #7149 ),
 ( #2442, #715 ),
 ( #4743, #4640 ),
 ( #9660, #8775 ),
 ( #6419, #3963 ),
 ( #2495, #3910 ),
 ( #7833, #9609 ),
 ( #7883, #5589 ),
 ( #6263, #5689 ),
 ( #5486, #5636 ) ),
 .UNSPECIFIED., .F., .F., .F.,
 ( 4, 1, 1, 1, 1, 1, 1, 1, 4 ),
 ( 2, 2 ),
 ( 0.000000000000000000, 0.1199228846740813259, 0.2396820999030742083, 0.3587608595380448184, 0.4799620281296770319, 0.6043577515038436321, 0.7314057062717854718, 0.8632643124108332344, 1.000000000000000000 ),
 ( 0.000000000000000000, 1.000000000000000000 ),
 .UNSPECIFIED. ) ;
#584=CARTESIAN_POINT ( 'NONE',  ( -22.57971655928959365, 99.50000000000000000, -10.84768434062017839 ) ) ;
#585=ORIENTED_EDGE ( 'NONE', *, *, #7658, .T. ) ;
#587=CARTESIAN_POINT ( 'NONE',  ( 0.000000000000000000, 87.00000000000001421, -25.00000000000000000 ) ) ;
#588=ORIENTED_EDGE ( 'NONE', *, *, #9469, .F. ) ;
#589=DIRECTION ( 'NONE',  ( -0.000000000000000000, 1.000000000000000000, -0.000000000000000000 ) ) ;
#590=CARTESIAN_POINT ( 'NONE',  ( -27.43301270000000969, 3.899999998907524912, 11.36312591709335429 ) ) ;
#593=CARTESIAN_POINT ( 'NONE',  ( -19.09188309203678813, 2.100000000000000089, 19.09188309203678457 ) ) ;
#596=CARTESIAN_POINT ( 'NONE',  ( -19.09188309203678813, 2.900000000000000355, 19.09188309203678457 ) ) ;
#597=CARTESIAN_POINT ( 'NONE',  ( 8.540544597724410991, 100.0000000000000000, 19.98924338346217766 ) ) ;
#598=ORIENTED_EDGE ( 'NONE', *, *, #8582, .F. ) ;
#601=CARTESIAN_POINT ( 'NONE',  ( -27.43301270000000258, 0.6499999989075253559, -3.359575119402369376E-15 ) ) ;
#605=CARTESIAN_POINT ( 'NONE',  ( 3.016803124593948393, 100.0000000000000142, -23.20507807535735978 ) ) ;
#606=CARTESIAN_POINT ( 'NONE',  ( 4.472992770554171216, 99.99999999999995737, -21.83386288566719458 ) ) ;
#608=CARTESIAN_POINT ( 'NONE',  ( 3.302864939465488536, 99.50000000000001421, -22.83905924565489443 ) ) ;
#612=ORIENTED_EDGE ( 'NONE', *, *, #428, .F. ) ;
#616=CARTESIAN_POINT ( 'NONE',  ( 9.263267005978743640, 99.99999999999998579, 19.65676951151765905 ) ) ;
#620=CARTESIAN_POINT ( 'NONE',  ( -15.49723655759404295, 99.99999999999997158, 15.26389171799780264 ) ) ;
#622=CARTESIAN_POINT ( 'NONE',  ( 27.43301270000000258, 1.149999998907525356, 0.000000000000000000 ) ) ;
#623=ORIENTED_EDGE ( 'NONE', *, *, #2893, .F. ) ;
#624=EDGE_CURVE ( 'NONE', #3939, #7023, #5461, .T. ) ;
#626=CARTESIAN_POINT ( 'NONE',  ( 3.638175769014108774, 99.49999999999998579, -21.10017783766535970 ) ) ;
#628=CARTESIAN_POINT ( 'NONE',  ( 19.09188309203678813, 0.6999999978150504010, -19.09188309203678813 ) ) ;
#629=CARTESIAN_POINT ( 'NONE',  ( 19.39806930854667399, 2.649999998907525356, 19.39806930854668465 ) ) ;
#630=CARTESIAN_POINT ( 'NONE',  ( -15.91084591538827198, 100.0000000000000142, 16.65047278764667027 ) ) ;
#631=PRODUCT_DEFINITION_FORMATION_WITH_SPECIFIED_SOURCE ( 'ANY', '', #7269, .NOT_KNOWN. ) ;
#632=CARTESIAN_POINT ( 'NONE',  ( 4.202475441399873723, 99.50000000000000000, -24.35385978717689071 ) ) ;
#633=CARTESIAN_POINT ( 'NONE',  ( 3.254133136943549776, 99.50000000000000000, -21.76036676155726823 ) ) ;
#634=CARTESIAN_POINT ( 'NONE',  ( -16.18965924272485779, 99.99999999999998579, 15.26525457555968224 ) ) ;
#636=CARTESIAN_POINT ( 'NONE',  ( -20.89052720883767122, 99.50000000000000000, -9.602653601535816819 ) ) ;
#637=EDGE_LOOP ( 'NONE', ( #5051, #8667, #546, #8200 ) ) ;
#639=ORIENTED_EDGE ( 'NONE', *, *, #3681, .F. ) ;
#642=CARTESIAN_POINT ( 'NONE',  ( 11.36312591709336139, 1.999999998907525223, -27.43301270000000258 ) ) ;
#643=LINE ( 'NONE', #2269, #10101 ) ;
#644=CARTESIAN_POINT ( 'NONE',  ( 19.09188309203678813, 0.9000000000000001332, -19.09188309203678813 ) ) ;
#646=CARTESIAN_POINT ( 'NONE',  ( 9.502908418173033667, 100.0000000000000284, 20.32929868008965002 ) ) ;
#647=VERTEX_POINT ( 'NONE', #4231 ) ;
#648=ORIENTED_EDGE ( 'NONE', *, *, #8962, .T. ) ;
#649=CARTESIAN_POINT ( 'NONE',  ( -16.57337958714257908, 99.99999999999994316, 15.99273699073067867 ) ) ;
#650=CARTESIAN_POINT ( 'NONE',  ( 8.281567445270807681, 100.0000000000000000, 20.15885744430370252 ) ) ;
#651=EDGE_CURVE ( 'NONE', #7760, #2327, #205, .T. ) ;
#653=VERTEX_POINT ( 'NONE', #3345 ) ;
#655=ADVANCED_FACE ( 'NONE', ( #7411 ), #2659, .F. ) ;
#656=CARTESIAN_POINT ( 'NONE',  ( -15.09818093130665773, 100.0000000000000000, 16.69478731934044191 ) ) ;
#657=CARTESIAN_POINT ( 'NONE',  ( -21.08523985030068459, 99.50000000000000000, -9.874866134143449159 ) ) ;
#659=DIRECTION ( 'NONE',  ( -0.000000000000000000, 1.000000000000000000, 0.000000000000000000 ) ) ;
#662=ORIENTED_EDGE ( 'NONE', *, *, #6983, .T. ) ;
#663=STYLED_ITEM('',(#10387),#6543);
#665=CARTESIAN_POINT ( 'NONE',  ( 8.429066232339796017, 99.50000000000000000, 19.67794530653910101 ) ) ;
#667=B_SPLINE_CURVE_WITH_KNOTS ( 'NONE', 3,
 ( #8704, #1525, #4822, #7964, #636, #7176, #7017, #4718, #7911, #1576, #10326, #6235, #7123, #7070, #4767, #3110, #800, #3991, #4 ),
 .UNSPECIFIED., .F., .F.,
 ( 4, 1, 1, 1, 1, 1, 1, 1, 1, 1, 1, 1, 1, 1, 1, 1, 4 ),
 ( 0.000000000000000000, 0.06358429906668214282, 0.1250797439647324816, 0.1854075229911844314, 0.2454523280917267347, 0.3052969617611028252, 0.3655926515411210831, 0.4275661794825392770, 0.4916205250740160460, 0.5555554127340263104, 0.6185525978810689773, 0.6803322039413655098, 0.7423868736098769849, 0.8044290668430417179, 0.8676072479036442964, 0.9329923078238739897, 1.000000000000000000 ),
 .UNSPECIFIED. ) ;
#669=VERTEX_POINT ( 'NONE', #158 ) ;
#670=DIRECTION ( 'NONE',  ( 0.9415546909775123208, 0.000000000000000000, 0.3368601548094423137 ) ) ;
#671=CARTESIAN_POINT ( 'NONE',  ( 8.751508028230254865, 99.49999999999998579, 19.58480916780017722 ) ) ;
#673=CARTESIAN_POINT ( 'NONE',  ( -22.34867803760930727, 99.49999999999998579, -10.48295844864103721 ) ) ;
#675=DIRECTION ( 'NONE',  ( 0.000000000000000000, 0.000000000000000000, 1.000000000000000000 ) ) ;
#676=CARTESIAN_POINT ( 'NONE',  ( -19.39806930854668465, 4.849999998907525978, 19.39806930854667755 ) ) ;
#679=DIRECTION ( 'NONE',  ( 0.000000000000000000, 1.000000000000000000, 0.000000000000000000 ) ) ;
#681=CARTESIAN_POINT ( 'NONE',  ( -16.91946509138130139, 99.50000000000001421, 15.98858002463268413 ) ) ;
#682=CARTESIAN_POINT ( 'NONE',  ( -19.39806930854667755, 1.449999998907525178, -19.39806930854668110 ) ) ;
#683=ADVANCED_FACE ( 'NONE', ( #2566 ), #4106, .T. ) ;
#684=CARTESIAN_POINT ( 'NONE',  ( -15.30066472929571653, 99.99999999999995737, 16.41738810589640707 ) ) ;
#685=CARTESIAN_POINT ( 'NONE',  ( 21.43339342948717885, 99.50000000000000000, -1.392427884615384803 ) ) ;
#691=EDGE_LOOP ( 'NONE', ( #5924, #5817, #2143, #8431 ) ) ;
#694=CARTESIAN_POINT ( 'NONE',  ( 19.39806930854667399, 1.849999998907525312, 19.39806930854668465 ) ) ;
#695=CARTESIAN_POINT ( 'NONE',  ( 1.679787559701184688E-15, 5.249999998907525445, -27.43301270000000258 ) ) ;
#696=CARTESIAN_POINT ( 'NONE',  ( 27.00000000000000355, 2.449999999999999734, -11.18376618407356737 ) ) ;
#697=CARTESIAN_POINT ( 'NONE',  ( 8.540544597724410991, 99.50000000000000000, 19.98924338346217766 ) ) ;
#698=ORIENTED_EDGE ( 'NONE', *, *, #6395, .F. ) ;
#699=EDGE_CURVE ( 'NONE', #2532, #728, #9823, .T. ) ;
#700=CARTESIAN_POINT ( 'NONE',  ( -15.11611088805441661, 99.50000000000000000, 16.06180012866831319 ) ) ;
#701=CARTESIAN_POINT ( 'NONE',  ( 4.154273145530666511, 100.0000000000000000, -22.82723029927519676 ) ) ;
#704=ORIENTED_EDGE ( 'NONE', *, *, #3027, .T. ) ;
#706=CARTESIAN_POINT ( 'NONE',  ( 11.36312591709336850, 2.499999998907525445, 27.43301269999999903 ) ) ;
#709=CARTESIAN_POINT ( 'NONE',  ( 1.653273178848927064E-15, 3.400000000000000355, -27.00000000000000355 ) ) ;
#712=ORIENTED_EDGE ( 'NONE', *, *, #5166, .F. ) ;
#715=CARTESIAN_POINT ( 'NONE',  ( 4.693123912524271191, 100.0000000000000426, -24.12247278045041554 ) ) ;
#717=VERTEX_POINT ( 'NONE', #4175 ) ;
#723=CARTESIAN_POINT ( 'NONE',  ( -22.06741020400400188, 100.0000000000000426, -9.788922322134999021 ) ) ;
#724=CARTESIAN_POINT ( 'NONE',  ( 9.526349065647009340, 100.0000000000000000, 19.81320455978211470 ) ) ;
#727=VECTOR ( 'NONE', #2964, 1000.000000000000000 ) ;
#728=VERTEX_POINT ( 'NONE', #7314 ) ;
#729=CARTESIAN_POINT ( 'NONE',  ( -14.89910828679519739, 99.49999999999997158, 16.44921749203638939 ) ) ;
#730=AXIS2_PLACEMENT_3D ( 'NONE', #813, #9600, #5627 ) ;
#731=CARTESIAN_POINT ( 'NONE',  ( -27.43301270000000969, 3.999999998907525001, 11.36312591709335784 ) ) ;
#732=ORIENTED_EDGE ( 'NONE', *, *, #8411, .T. ) ;
#734=CARTESIAN_POINT ( 'NONE',  ( 2.843562173796539749, 99.99999999999998579, -21.91597968833000110 ) ) ;
#737=CARTESIAN_POINT ( 'NONE',  ( -27.00000000000001421, 1.849999997815050534, 11.18376618407356382 ) ) ;
#739=CARTESIAN_POINT ( 'NONE',  ( -15.26676860252058887, 99.99999999999995737, 16.38168943497750973 ) ) ;
#740=FACE_OUTER_BOUND ( 'NONE', #5569, .T. ) ;
#744=CARTESIAN_POINT ( 'NONE',  ( 3.207057600658871355, 100.0000000000000000, -22.07913334414698880 ) ) ;
#745=EDGE_LOOP ( 'NONE', ( #5561, #5687, #828, #2897, #6185, #7299 ) ) ;
#746=ADVANCED_FACE ( 'NONE', ( #9763 ), #927, .T. ) ;
#748=CARTESIAN_POINT ( 'NONE',  ( 27.43301270000000258, 4.299999998907525267, -11.36312591709336139 ) ) ;
#750=CARTESIAN_POINT ( 'NONE',  ( -15.98658610793439117, 99.50000000000001421, 14.83943845084690949 ) ) ;
#751=CARTESIAN_POINT ( 'NONE',  ( -19.09188309203678813, 0.5000000000000000000, 19.09188309203678457 ) ) ;
#752=FACE_OUTER_BOUND ( 'NONE', #6503, .T. ) ;
#754=ORIENTED_EDGE ( 'NONE', *, *, #7355, .T. ) ;
#755=LINE ( 'NONE', #9737, #9328 ) ;
#756=CARTESIAN_POINT ( 'NONE',  ( 8.515772100368442565, 99.50000000000000000, 20.00046577258137503 ) ) ;
#758=PLANE ( 'NONE',  #8147 ) ;
#759=CARTESIAN_POINT ( 'NONE',  ( 19.39806930854667399, 3.349999998907525534, 19.39806930854668465 ) ) ;
#760=CARTESIAN_POINT ( 'NONE',  ( -19.09188309203678813, 2.100000000000000089, 19.09188309203678457 ) ) ;
#761=ADVANCED_FACE ( 'NONE', ( #8939 ), #6178, .T. ) ;
#762=B_SPLINE_SURFACE_WITH_KNOTS ( 'NONE', 3, 1, ( 
 ( #3955, #8033 ),
 ( #7139, #866 ),
 ( #3176, #558 ),
 ( #9555, #8085 ),
 ( #4056, #8868 ),
 ( #2383, #7240 ),
 ( #8511, #2487 ),
 ( #3317, #10137 ),
 ( #5579, #1593 ),
 ( #6507, #2536 ),
 ( #1340, #6600 ),
 ( #9063, #5917 ),
 ( #8966, #9790 ),
 ( #3461, #1783 ),
 ( #9113, #4978 ) ),
 .UNSPECIFIED., .F., .F., .F.,
 ( 4, 1, 1, 1, 1, 1, 1, 1, 1, 1, 1, 1, 4 ),
 ( 2, 2 ),
 ( 0.000000000000000000, 0.08450893420292937552, 0.1670077533940913517, 0.2489527561816328172, 0.3323249201989921797, 0.4152786837838207679, 0.4972150204155297848, 0.5791806016509544186, 0.6636863847498374325, 0.7483757861910059761, 0.8320455266939520422, 0.9153409992114193150, 1.000000000000000000 ),
 ( 0.000000000000000000, 1.000000000000000000 ),
 .UNSPECIFIED. ) ;
#763=FACE_OUTER_BOUND ( 'NONE', #9911, .T. ) ;
#767=CARTESIAN_POINT ( 'NONE',  ( -16.65546786808457469, 99.49999999999998579, 16.57295196178722918 ) ) ;
#772=CARTESIAN_POINT ( 'NONE',  ( 0.000000000000000000, 100.0000000000000000, -27.00000000000000355 ) ) ;
#776=VERTEX_POINT ( 'NONE', #1445 ) ;
#777=FACE_BOUND ( 'NONE', #9157, .T. ) ;
#779=CARTESIAN_POINT ( 'NONE',  ( -22.31427554260534052, 99.50000000000002842, -10.13077409178744404 ) ) ;
#780=EDGE_CURVE ( 'NONE', #4040, #6656, #6147, .T. ) ;
#783=ORIENTED_EDGE ( 'NONE', *, *, #1218, .F. ) ;
#786=VECTOR ( 'NONE', #10019, 1000.000000000000114 ) ;
#787=CARTESIAN_POINT ( 'NONE',  ( 3.212364564527730337, 100.0000000000000000, -22.10366694310577884 ) ) ;
#789=CARTESIAN_POINT ( 'NONE',  ( -20.99557965837879081, 99.49999999999997158, -10.74478602187354959 ) ) ;
#790=CARTESIAN_POINT ( 'NONE',  ( -19.39806930854668465, 4.049999998907525267, 19.39806930854667755 ) ) ;
#792=CARTESIAN_POINT ( 'NONE',  ( -20.63666786535793207, 99.49999999999998579, -10.16306733409737717 ) ) ;
#795=CARTESIAN_POINT ( 'NONE',  ( -15.31787750341841559, 99.50000000000001421, 16.43551622900274722 ) ) ;
#796=CARTESIAN_POINT ( 'NONE',  ( 10.85214315541671759, 100.0000000000000000, 22.51047735782115211 ) ) ;
#797=AXIS2_PLACEMENT_3D ( 'NONE', #9860, #6717, #4315 ) ;
#800=CARTESIAN_POINT ( 'NONE',  ( -21.99154324187120579, 99.50000000000001421, -9.362771248264911250 ) ) ;
#802=CARTESIAN_POINT ( 'NONE',  ( -11.36312591709337383, 1.699999998907525178, 27.43301269999999548 ) ) ;
#803=CARTESIAN_POINT ( 'NONE',  ( 1.679787559701184688E-15, 5.316666665574192763, -27.43301270000000258 ) ) ;
#804=CARTESIAN_POINT ( 'NONE',  ( 19.09188309203678813, 3.299999999999999822, -19.09188309203678813 ) ) ;
#805=CARTESIAN_POINT ( 'NONE',  ( 2.964854786877021642, 100.0000000000000000, -22.43901021186594846 ) ) ;
#807=CARTESIAN_POINT ( 'NONE',  ( 8.187169943530866689, 99.49999999999998579, 20.27434297626003712 ) ) ;
#810=ORIENTED_EDGE ( 'NONE', *, *, #9, .F. ) ;
#811=CARTESIAN_POINT ( 'NONE',  ( 11.36312591709336139, 3.599999998907525089, -27.43301270000000258 ) ) ;
#812=CARTESIAN_POINT ( 'NONE',  ( 3.977571997893210032, 100.0000000000000000, -24.70179182097838932 ) ) ;
#813=CARTESIAN_POINT ( 'NONE',  ( 9.248677610544923766, 99.50000000000000000, 22.83089001807756446 ) ) ;
#817=CARTESIAN_POINT ( 'NONE',  ( -4.959819536546781389E-15, 1.399999999999999911, 27.00000000000000355 ) ) ;
#818=CARTESIAN_POINT ( 'NONE',  ( 11.18376618407357626, 5.249999997815050889, 27.00000000000000000 ) ) ;
#819=ORIENTED_EDGE ( 'NONE', *, *, #5028, .T. ) ;
#820=EDGE_CURVE ( 'NONE', #224, #4694, #7051, .T. ) ;
#823=FACE_OUTER_BOUND ( 'NONE', #7757, .T. ) ;
#825=CARTESIAN_POINT ( 'NONE',  ( -21.30928386698190025, 99.50000000000000000, -11.02857376369709996 ) ) ;
#827=VERTEX_POINT ( 'NONE', #4374 ) ;
#828=ORIENTED_EDGE ( 'NONE', *, *, #7593, .T. ) ;
#831=CARTESIAN_POINT ( 'NONE',  ( -22.35642768247353729, 99.49999999999995737, -10.34293228154892752 ) ) ;
#832=CARTESIAN_POINT ( 'NONE',  ( -14.97509118869195888, 99.49999999999998579, 15.26515554624281101 ) ) ;
#833=CARTESIAN_POINT ( 'NONE',  ( -5.039362679103552881E-15, 4.149999998907524912, 27.43301270000000258 ) ) ;
#834=VERTEX_POINT ( 'NONE', #9345 ) ;
#837=CARTESIAN_POINT ( 'NONE',  ( -20.96129225301843135, 100.0000000000000142, -10.68089388303413934 ) ) ;
#840=CARTESIAN_POINT ( 'NONE',  ( -21.13504512532655610, 99.50000000000000000, -11.31853095674525100 ) ) ;
#841=CARTESIAN_POINT ( 'NONE',  ( -11.36312591709337383, 4.099999998907525089, 27.43301269999999548 ) ) ;
#842=CARTESIAN_POINT ( 'NONE',  ( -15.26676860252058887, 99.49999999999998579, 16.38168943497750973 ) ) ;
#844=CARTESIAN_POINT ( 'NONE',  ( 0.000000000000000000, 0.000000000000000000, 0.000000000000000000 ) ) ;
#845=CARTESIAN_POINT ( 'NONE',  ( 3.231466532446834350, 99.99999999999997158, -21.81145066552309686 ) ) ;
#849=CARTESIAN_POINT ( 'NONE',  ( 9.820792995160308791, 100.0000000000000000, 20.21220011423140761 ) ) ;
#853=CARTESIAN_POINT ( 'NONE',  ( -11.36312591709335962, 4.499999998907525445, -27.43301270000000258 ) ) ;
#854=DIRECTION ( 'NONE',  ( -0.1697592580069431922, 0.000000000000000000, 0.9854855627156250408 ) ) ;
#855=CARTESIAN_POINT ( 'NONE',  ( -5.039362679103552881E-15, 0.8499999989075253115, 27.43301270000000258 ) ) ;
#860=CARTESIAN_POINT ( 'NONE',  ( 8.132491713109025966, 99.50000000000000000, 21.08089001807756091 ) ) ;
#861=CARTESIAN_POINT ( 'NONE',  ( 4.909381318607588973, 99.50000000000000000, -23.54377677363417121 ) ) ;
#863=CARTESIAN_POINT ( 'NONE',  ( -11.36312591709337561, 3.999999998907525889, 27.43301269999999548 ) ) ;
#866=CARTESIAN_POINT ( 'NONE',  ( -22.55793349878803156, 100.0000000000000000, -10.88926985104519929 ) ) ;
#868=CARTESIAN_POINT ( 'NONE',  ( -16.54770463920453949, 100.0000000000000284, 15.70234036036222847 ) ) ;
#869=CARTESIAN_POINT ( 'NONE',  ( -16.84090648038580085, 99.99999999999998579, 15.49469789757679727 ) ) ;
#870=CARTESIAN_POINT ( 'NONE',  ( 5.142436925601051811, 99.99999999999995737, -24.04117066426968563 ) ) ;
#872=VERTEX_POINT ( 'NONE', #5374 ) ;
#873=CARTESIAN_POINT ( 'NONE',  ( 8.685676809262872666, 99.50000000000000000, 23.43455588346217766 ) ) ;
#874=EDGE_CURVE ( 'NONE', #3238, #9838, #4617, .T. ) ;
#875=CARTESIAN_POINT ( 'NONE',  ( -14.83571502646304197, 100.0000000000000426, 16.32397075880403392 ) ) ;
#877=AXIS2_PLACEMENT_3D ( 'NONE', #9689, #1582, #14 ) ;
#878=ORIENTED_EDGE ( 'NONE', *, *, #6262, .F. ) ;
#879=DIRECTION ( 'NONE',  ( 0.3368601548094422582, 0.000000000000000000, -0.9415546909775122097 ) ) ;
#881=CARTESIAN_POINT ( 'NONE',  ( -22.28738277804067636, 99.49999999999997158, -10.06255608345902886 ) ) ;
#882=DIRECTION ( 'NONE',  ( -0.000000000000000000, -1.000000000000000000, -0.000000000000000000 ) ) ;
#884=CARTESIAN_POINT ( 'NONE',  ( 9.482997300390421103, 100.0000000000000000, 20.28643943712827991 ) ) ;
#885=AXIS2_PLACEMENT_3D ( 'NONE', #1301, #7484, #4250 ) ;
#886=FACE_OUTER_BOUND ( 'NONE', #8707, .T. ) ;
#888=CARTESIAN_POINT ( 'NONE',  ( 3.269123371500344710, 99.99999999999998579, -23.64665713169964434 ) ) ;
#890=CARTESIAN_POINT ( 'NONE',  ( -21.24310748994415832, 99.49999999999998579, -10.99527971241054658 ) ) ;
#891=CARTESIAN_POINT ( 'NONE',  ( -5.039362679103552881E-15, 4.949999998907525622, 27.43301270000000258 ) ) ;
#892=CARTESIAN_POINT ( 'NONE',  ( -15.15623813234777018, 99.50000000000000000, 16.19783826294960249 ) ) ;
#893=AXIS2_PLACEMENT_3D ( 'NONE', #8051, #4077, #5944 ) ;
#894=CARTESIAN_POINT ( 'NONE',  ( -21.94169572595625795, 100.0000000000000000, -9.715372641902229489 ) ) ;
#895=CARTESIAN_POINT ( 'NONE',  ( -15.55395551812965671, 99.50000000000002842, 16.59868653893595791 ) ) ;
#896=CARTESIAN_POINT ( 'NONE',  ( -22.51767453479306980, 100.0000000000000000, -9.764155749770198511 ) ) ;
#898=PLANE ( 'NONE',  #9130 ) ;
#900=CARTESIAN_POINT ( 'NONE',  ( 11.36312591709336139, 4.399999998907525800, -27.43301270000000258 ) ) ;
#902=CARTESIAN_POINT ( 'NONE',  ( -16.07368679829020763, 99.50000000000000000, 17.11560437002838952 ) ) ;
#904=CARTESIAN_POINT ( 'NONE',  ( -4.959819536546781389E-15, 4.599999999999999645, 27.00000000000000355 ) ) ;
#905=CARTESIAN_POINT ( 'NONE',  ( -20.79740905086423552, 100.0000000000000142, -11.06234285579171051 ) ) ;
#907=CARTESIAN_POINT ( 'NONE',  ( -16.35834224700816009, 99.50000000000000000, 16.43761959438736397 ) ) ;
#908=DIRECTION ( 'NONE',  ( -0.000000000000000000, -1.000000000000000000, -0.000000000000000000 ) ) ;
#909=ORIENTED_EDGE ( 'NONE', *, *, #1596, .F. ) ;
#910=CARTESIAN_POINT ( 'NONE',  ( -20.77412980915959650, 99.49999999999997158, -9.759484723497815040 ) ) ;
#911=EDGE_CURVE ( 'NONE', #9838, #3238, #8959, .T. ) ;
#912=DIRECTION ( 'NONE',  ( -0.9415543565890244215, 0.000000000000000000, -0.3368610894541372303 ) ) ;
#913=CARTESIAN_POINT ( 'NONE',  ( 3.409892249890944527, 100.0000000000000000, -24.50637943905448779 ) ) ;
#915=CARTESIAN_POINT ( 'NONE',  ( -19.09188309203678457, 0.8999999978150503566, -19.09188309203678813 ) ) ;
#917=CARTESIAN_POINT ( 'NONE',  ( -16.37547766376588854, 100.0000000000000000, 16.41943072543956816 ) ) ;
#918=CARTESIAN_POINT ( 'NONE',  ( -22.13144646319157260, 100.0000000000000142, -9.428651666388001118 ) ) ;
#919=CARTESIAN_POINT ( 'NONE',  ( 8.081885929396888102, 100.0000000000000142, 20.89785832093561169 ) ) ;
#922=ORIENTED_EDGE ( 'NONE', *, *, #4166, .T. ) ;
#924=CARTESIAN_POINT ( 'NONE',  ( -15.58193289918752278, 100.0000000000000000, 16.98546238400348329 ) ) ;
#925=CARTESIAN_POINT ( 'NONE',  ( 9.184850993605147944E-16, 87.00000000000001421, 7.500000000000000000 ) ) ;
#927=B_SPLINE_SURFACE_WITH_KNOTS ( 'NONE', 3, 1, ( 
 ( #8251, #3487 ),
 ( #5795, #3339 ),
 ( #346, #8300 ),
 ( #5100, #9089 ),
 ( #245, #8987 ),
 ( #2559, #6671 ),
 ( #3429, #9867 ),
 ( #2652, #1807 ),
 ( #297, #5154 ),
 ( #1078, #6726 ),
 ( #152, #7456 ),
 ( #3537, #7507 ),
 ( #6623, #1959 ),
 ( #5893, #6530 ),
 ( #1906, #9922 ),
 ( #5948, #4223 ),
 ( #4130, #4274 ),
 ( #7403, #3380 ),
 ( #6575, #2604 ) ),
 .UNSPECIFIED., .F., .F., .F.,
 ( 4, 1, 1, 1, 1, 1, 1, 1, 1, 1, 1, 1, 1, 1, 1, 1, 4 ),
 ( 2, 2 ),
 ( 0.000000000000000000, 0.06839333837245492598, 0.1346519561570838353, 0.1985335841112251809, 0.2613354512981445610, 0.3228799447584090876, 0.3842093944964607433, 0.4462111754260434937, 0.5089246482083435996, 0.5715029624870164859, 0.6324491702983550123, 0.6923675070709934820, 0.7521785462597534444, 0.8119602890481165680, 0.8728645645504365946, 0.9355733815441056311, 1.000000000000000000 ),
 ( 0.000000000000000000, 1.000000000000000000 ),
 .UNSPECIFIED. ) ;
#928=ORIENTED_EDGE ( 'NONE', *, *, #3384, .F. ) ;
#930=CARTESIAN_POINT ( 'NONE',  ( -20.63200021313574695, 99.50000000000000000, -10.19493994959453431 ) ) ;
#931=LINE ( 'NONE', #8151, #4479 ) ;
#932=CARTESIAN_POINT ( 'NONE',  ( -15.07178375341841559, 99.50000000000001421, 15.16157792772069968 ) ) ;
#933=CARTESIAN_POINT ( 'NONE',  ( -27.00000000000001421, 4.450000000000000178, 11.18376618407356560 ) ) ;
#936=CARTESIAN_POINT ( 'NONE',  ( 4.061806280070601183, 100.0000000000000142, -22.51960061163626392 ) ) ;
#937=CARTESIAN_POINT ( 'NONE',  ( 4.232447118646125439, 99.49999999999998579, -21.54138831197867887 ) ) ;
#938=CARTESIAN_POINT ( 'NONE',  ( -20.91264567078791714, 99.49999999999997158, -10.54226115003387676 ) ) ;
#939=CARTESIAN_POINT ( 'NONE',  ( -27.43301270000000969, 3.999999998907525001, 11.36312591709335429 ) ) ;
#941=CARTESIAN_POINT ( 'NONE',  ( -4.959819536546781389E-15, 3.000000000000000000, 27.00000000000000355 ) ) ;
#942=CARTESIAN_POINT ( 'NONE',  ( 11.18376618407357093, 3.949999997815050179, -27.00000000000000355 ) ) ;
#943=CARTESIAN_POINT ( 'NONE',  ( -15.83671465916681242, 99.50000000000000000, 16.65403364262263608 ) ) ;
#945=CARTESIAN_POINT ( 'NONE',  ( -21.37606745505193473, 99.50000000000002842, -11.05925878703054011 ) ) ;
#950=CARTESIAN_POINT ( 'NONE',  ( 27.43301269999999548, 0.9999999989075254447, 11.36312591709337738 ) ) ;
#951=B_SPLINE_CURVE_WITH_KNOTS ( 'NONE', 3,
 ( #8897, #7961, #5660, #4036, #2412, #6536, #7173, #3986, #9723, #943, #10366, #4137, #3344, #895, #7319, #5607, #108, #3251, #795 ),
 .UNSPECIFIED., .F., .F.,
 ( 4, 1, 1, 1, 1, 1, 1, 1, 1, 1, 1, 1, 1, 1, 1, 1, 4 ),
 ( 0.000000000000000000, 0.06473117683888822416, 0.1283191082976379849, 0.1900130092022370987, 0.2509653124206144836, 0.3118694605430146760, 0.3735603890354366463, 0.4359106579620777855, 0.5007804971236301528, 0.5656503362851855732, 0.6280858374182423098, 0.6899222460797727052, 0.7510277903999277305, 0.8114330998898260372, 0.8726106248506092511, 0.9357151229638154266, 1.000000000000000000 ),
 .UNSPECIFIED. ) ;
#956=EDGE_CURVE ( 'NONE', #4002, #7760, #7549, .T. ) ;
#958=AXIS2_PLACEMENT_3D ( 'NONE', #6633, #9875, #3391 ) ;
#961=SURFACE_STYLE_FILL_AREA ( #5129 ) ;
#963=LINE ( 'NONE', #3178, #4889 ) ;
#964=CARTESIAN_POINT ( 'NONE',  ( -16.90689012439429462, 99.49999999999998579, 16.08742389234230785 ) ) ;
#965=CARTESIAN_POINT ( 'NONE',  ( 5.207032889226773875, 100.0000000000000000, -23.83708953234284778 ) ) ;
#966=EDGE_CURVE ( 'NONE', #2239, #2880, #5183, .T. ) ;
#967=EDGE_CURVE ( 'NONE', #7282, #872, #8454, .T. ) ;
#969=VERTEX_POINT ( 'NONE', #8920 ) ;
#972=FACE_OUTER_BOUND ( 'NONE', #7578, .T. ) ;
#973=CARTESIAN_POINT ( 'NONE',  ( -21.37606745505193473, 99.50000000000002842, -11.05925878703054011 ) ) ;
#976=CIRCLE ( 'NONE', #7648, 27.00000000000000355 ) ;
#977=ORIENTED_EDGE ( 'NONE', *, *, #8288, .F. ) ;
#978=LINE ( 'NONE', #1708, #6313 ) ;
#980=CARTESIAN_POINT ( 'NONE',  ( -27.00000000000001421, 2.649999997815050357, 11.18376618407356560 ) ) ;
#981=CARTESIAN_POINT ( 'NONE',  ( 4.049441352997683374, 99.50000000000000000, -21.43849541167161732 ) ) ;
#982=CARTESIAN_POINT ( 'NONE',  ( 3.434779879277784609, 99.99999999999998579, -23.17575050830969374 ) ) ;
#983=CARTESIAN_POINT ( 'NONE',  ( 4.277141017070624329, 100.0000000000000000, -21.57940364907851816 ) ) ;
#984=CARTESIAN_POINT ( 'NONE',  ( 3.222930479149370253, 99.49999999999995737, -22.15251218086615381 ) ) ;
#985=CARTESIAN_POINT ( 'NONE',  ( 27.00000000000000355, 3.049999997815050268, -11.18376618407356737 ) ) ;
#988=CARTESIAN_POINT ( 'NONE',  ( 3.552835461024879127, 100.0000000000000000, -21.47801279722421697 ) ) ;
#989=DIRECTION ( 'NONE',  ( -0.9851965920526258857, 0.000000000000000000, -0.1714283378204774222 ) ) ;
#996=CARTESIAN_POINT ( 'NONE',  ( 19.39806930854667399, 0.9499999989075252893, 19.39806930854668465 ) ) ;
#997=CARTESIAN_POINT ( 'NONE',  ( 3.105863891863242632, 99.50000000000001421, -22.59672720503480292 ) ) ;
#998=DIRECTION ( 'NONE',  ( -0.000000000000000000, 1.000000000000000000, -0.000000000000000000 ) ) ;
#999=CARTESIAN_POINT ( 'NONE',  ( -19.46743691185369585, 99.50000000000000000, -8.912588186774021537 ) ) ;
#1000=CARTESIAN_POINT ( 'NONE',  ( -21.28703419482447146, 99.49999999999997158, -11.01737971290317297 ) ) ;
#1001=ORIENTED_EDGE ( 'NONE', *, *, #2037, .T. ) ;
#1002=CARTESIAN_POINT ( 'NONE',  ( -20.82968571475833031, 99.99999999999994316, -9.677916414284339908 ) ) ;
#1003=CARTESIAN_POINT ( 'NONE',  ( 3.171774962637509798, 100.0000000000000000, -24.28498992023182268 ) ) ;
#1004=CARTESIAN_POINT ( 'NONE',  ( 9.576498344683301411, 99.49999999999998579, 20.78592410672095880 ) ) ;
#1005=( LENGTH_UNIT ( ) NAMED_UNIT ( * ) SI_UNIT ( .MILLI., .METRE. ) );
#1007=CARTESIAN_POINT ( 'NONE',  ( -22.58826642033182353, 99.49999999999998579, -9.883148377786627137 ) ) ;
#1008=EDGE_CURVE ( 'NONE', #7448, #9173, #9916, .T. ) ;
#1009=EDGE_CURVE ( 'NONE', #2960, #2104, #4408, .T. ) ;
#1010=CARTESIAN_POINT ( 'NONE',  ( -16.91659681606879317, 100.0000000000000000, 15.78485274883190392 ) ) ;
#1011=CARTESIAN_POINT ( 'NONE',  ( 5.226890989224467710, 100.0000000000000000, -23.72545275563321354 ) ) ;
#1014=ORIENTED_EDGE ( 'NONE', *, *, #445, .T. ) ;
#1015=CARTESIAN_POINT ( 'NONE',  ( -21.29537297865864431, 100.0000000000000000, -11.39144590536739976 ) ) ;
#1016=CARTESIAN_POINT ( 'NONE',  ( 3.214822648120007731, 99.50000000000000000, -21.86319392453323829 ) ) ;
#1017=CARTESIAN_POINT ( 'NONE',  ( -14.83363727892122519, 100.0000000000000142, 15.50654517199034466 ) ) ;
#1019=CARTESIAN_POINT ( 'NONE',  ( 8.117007248954752896, 99.50000000000001421, 20.40979824468519155 ) ) ;
#1020=CARTESIAN_POINT ( 'NONE',  ( 4.100286767325537873, 99.50000000000000000, -22.51382885696750336 ) ) ;
#1023=ORIENTED_EDGE ( 'NONE', *, *, #7917, .T. ) ;
#1024=B_SPLINE_CURVE_WITH_KNOTS ( 'NONE', 3,
 ( #10301, #5538, #4014, #1656, #3133, #3079, #8878, #3856, #9513, #4847, #8040, #7043, #2338, #10248, #9462, #4207, #5830, #7301, #9076 ),
 .UNSPECIFIED., .F., .F.,
 ( 4, 1, 1, 1, 1, 1, 1, 1, 1, 1, 1, 1, 1, 1, 1, 1, 4 ),
 ( 0.000000000000000000, 0.07315862907712983310, 0.1430989967074559055, 0.2105333571262071879, 0.2759142635903734653, 0.3397077151413689933, 0.4013946392018796772, 0.4627937533375801049, 0.5237250720276656057, 0.5836284080752294212, 0.6425725562371763511, 0.7010486867616194662, 0.7591976973140022178, 0.8177727706511607186, 0.8769111530050104353, 0.9375229829315941954, 1.000000000000000000 ),
 .UNSPECIFIED. ) ;
#1025=DIRECTION ( 'NONE',  ( 0.000000000000000000, 0.000000000000000000, -1.000000000000000000 ) ) ;
#1027=CIRCLE ( 'NONE', #1540, 25.15000000000000213 ) ;
#1028=EDGE_CURVE ( 'NONE', #6302, #10278, #5133, .T. ) ;
#1030=CARTESIAN_POINT ( 'NONE',  ( 3.845216150098881513, 99.99999999999997158, -21.40922359334548020 ) ) ;
#1031=CARTESIAN_POINT ( 'NONE',  ( 3.291601991079349698, 99.49999999999997158, -22.28586332678438353 ) ) ;
#1032=CARTESIAN_POINT ( 'NONE',  ( -19.09188309203678813, 2.699999997815051067, 19.09188309203678457 ) ) ;
#1033=CARTESIAN_POINT ( 'NONE',  ( -20.88772068548257366, 99.50000000000001421, -11.14739719174079546 ) ) ;
#1034=CARTESIAN_POINT ( 'NONE',  ( -21.38163724633288965, 100.0000000000000568, -9.681902434707239991 ) ) ;
#1038=FACE_OUTER_BOUND ( 'NONE', #2724, .T. ) ;
#1039=FACE_OUTER_BOUND ( 'NONE', #9827, .T. ) ;
#1040=EDGE_LOOP ( 'NONE', ( #6213, #6520, #7596, #4974 ) ) ;
#1043=CARTESIAN_POINT ( 'NONE',  ( -14.78677372028383097, 99.99999999999997158, 15.63810349997947569 ) ) ;
#1046=CARTESIAN_POINT ( 'NONE',  ( -27.43301270000000969, 2.299999998907525267, 11.36312591709335429 ) ) ;
#1048=B_SPLINE_CURVE_WITH_KNOTS ( 'NONE', 3,
 ( #695, #7704, #1429, #3115 ),
 .UNSPECIFIED., .F., .F.,
 ( 4, 4 ),
 ( 0.000000000000000000, 1.000000000000000000 ),
 .UNSPECIFIED. ) ;
#1049=CARTESIAN_POINT ( 'NONE',  ( -16.35834224700816009, 100.0000000000000142, 16.43761959438736397 ) ) ;
#1050=CARTESIAN_POINT ( 'NONE',  ( 4.739008722453744049, 100.0000000000000142, -24.06821587619827696 ) ) ;
#1051=CARTESIAN_POINT ( 'NONE',  ( -20.89145576992255116, 99.99999999999994316, -10.33073932272468198 ) ) ;
#1053=CARTESIAN_POINT ( 'NONE',  ( 7.856939908706818798, 99.50000000000001421, 20.19612520319305560 ) ) ;
#1054=CARTESIAN_POINT ( 'NONE',  ( 27.43301269999999548, 4.999999998907525445, 11.36312591709337916 ) ) ;
#1055=CARTESIAN_POINT ( 'NONE',  ( 7.486453019397995234, 100.0000000000000000, 23.81666162955709964 ) ) ;
#1056=FILL_AREA_STYLE_COLOUR ( '', #6062 ) ;
#1057=CARTESIAN_POINT ( 'NONE',  ( -22.08823018108446234, 99.50000000000000000, -9.406177930363766038 ) ) ;
#1058=CARTESIAN_POINT ( 'NONE',  ( 9.304660012616079001, 99.50000000000000000, 20.07619068507570859 ) ) ;
#1059=CARTESIAN_POINT ( 'NONE',  ( 9.513000527211589841, 99.50000000000000000, 20.35102222961602436 ) ) ;
#1060=CARTESIAN_POINT ( 'NONE',  ( -21.87421819196487505, 100.0000000000000000, -9.684578881761979119 ) ) ;
#1064=EDGE_CURVE ( 'NONE', #3729, #7819, #7433, .T. ) ;
#1065=CARTESIAN_POINT ( 'NONE',  ( -22.35673484330673944, 99.99999999999998579, -10.41320610523044721 ) ) ;
#1066=CARTESIAN_POINT ( 'NONE',  ( 3.611424427577684781, 99.50000000000001421, -21.45475674085064099 ) ) ;
#1067=LINE ( 'NONE', #1892, #5390 ) ;
#1068=VECTOR ( 'NONE', #10226, 1000.000000000000000 ) ;
#1069=FACE_BOUND ( 'NONE', #4305, .T. ) ;
#1071=CARTESIAN_POINT ( 'NONE',  ( -22.16320288552370243, 100.0000000000000142, -10.86869938533413915 ) ) ;
#1072=CARTESIAN_POINT ( 'NONE',  ( 3.296462644833695776, 99.50000000000001421, -23.81854410834942115 ) ) ;
#1073=VERTEX_POINT ( 'NONE', #5078 ) ;
#1074=CARTESIAN_POINT ( 'NONE',  ( 4.100286767325537873, 99.50000000000000000, -22.51382885696750336 ) ) ;
#1075=CARTESIAN_POINT ( 'NONE',  ( -27.43301270000000969, 3.199999998907525178, 11.36312591709335429 ) ) ;
#1077=LINE ( 'NONE', #7455, #9617 ) ;
#1078=CARTESIAN_POINT ( 'NONE',  ( 7.809833820264425519, 99.49999999999995737, 20.29999375863051370 ) ) ;
#1080=ORIENTED_EDGE ( 'NONE', *, *, #319, .T. ) ;
#1081=DIRECTION ( 'NONE',  ( -0.000000000000000000, -1.000000000000000000, -0.000000000000000000 ) ) ;
#1082=CARTESIAN_POINT ( 'NONE',  ( 11.18376618407357626, 3.649999997815050357, 27.00000000000000000 ) ) ;
#1083=ADVANCED_FACE ( 'NONE', ( #6026 ), #1268, .F. ) ;
#1084=CARTESIAN_POINT ( 'NONE',  ( -20.69312081029678296, 99.99999999999997158, -9.926742041671966277 ) ) ;
#1088=CARTESIAN_POINT ( 'NONE',  ( -21.65488089977124275, 99.99999999999997158, -11.10326233039539723 ) ) ;
#1089=CARTESIAN_POINT ( 'NONE',  ( 3.203979444200292015, 100.0000000000000000, -21.29640115293693725 ) ) ;
#1090=LINE ( 'NONE', #9045, #7449 ) ;
#1091=AXIS2_PLACEMENT_3D ( 'NONE', #7906, #2309, #6437 ) ;
#1095=CARTESIAN_POINT ( 'NONE',  ( 27.43301269999999548, 4.199999998907525622, 11.36312591709337738 ) ) ;
#1096=CARTESIAN_POINT ( 'NONE',  ( -19.09188309203678457, 0.3000000000000000444, -19.09188309203678813 ) ) ;
#1098=CARTESIAN_POINT ( 'NONE',  ( 4.584380863705032283, 100.0000000000000142, -24.21384527865288305 ) ) ;
#1100=ORIENTED_EDGE ( 'NONE', *, *, #2793, .F. ) ;
#1101=CARTESIAN_POINT ( 'NONE',  ( -20.95972469638759250, 99.50000000000000000, -9.536167108072199028 ) ) ;
#1102=CARTESIAN_POINT ( 'NONE',  ( -21.16695614262292580, 100.0000000000000000, -11.33496398805607441 ) ) ;
#1104=( NAMED_UNIT ( * ) PLANE_ANGLE_UNIT ( ) SI_UNIT ( $, .RADIAN. ) );
#1105=CARTESIAN_POINT ( 'NONE',  ( 21.79306891025641235, 99.50000000000000000, -1.065004006410256387 ) ) ;
#1106=CYLINDRICAL_SURFACE ( 'NONE', #885, 27.00000000000000355 ) ;
#1107=CARTESIAN_POINT ( 'NONE',  ( -16.60513711880302878, 99.50000000000000000, 15.15667007515659570 ) ) ;
#1108=AXIS2_PLACEMENT_3D ( 'NONE', #6420, #5590, #8776 ) ;
#1109=CARTESIAN_POINT ( 'NONE',  ( -21.24882413972086681, 100.0000000000000284, -9.742484589929601313 ) ) ;
#1111=CARTESIAN_POINT ( 'NONE',  ( -15.91084591538827198, 100.0000000000000142, 16.65047278764667027 ) ) ;
#1112=VECTOR ( 'NONE', #3494, 1000.000000000000000 ) ;
#1114=VERTEX_POINT ( 'NONE', #1214 ) ;
#1116=AXIS2_PLACEMENT_3D ( 'NONE', #4023, #36, #2597 ) ;
#1117=CARTESIAN_POINT ( 'NONE',  ( -21.84904385032055174, 99.99999999999998579, -11.42736543092427404 ) ) ;
#1118=CARTESIAN_POINT ( 'NONE',  ( 3.254133136943549776, 99.99999999999997158, -21.76036676155726823 ) ) ;
#1120=CARTESIAN_POINT ( 'NONE',  ( -11.18376618407356737, 3.249999997815050001, -27.00000000000000355 ) ) ;
#1123=FACE_OUTER_BOUND ( 'NONE', #3482, .T. ) ;
#1124=CARTESIAN_POINT ( 'NONE',  ( 9.692323321704657602, 100.0000000000000142, 21.58969587442354410 ) ) ;
#1127=CARTESIAN_POINT ( 'NONE',  ( -27.43301270000000258, 2.299999998907525267, -11.36312591709336317 ) ) ;
#1129=AXIS2_PLACEMENT_3D ( 'NONE', #5815, #8321, #4395 ) ;
#1130=CARTESIAN_POINT ( 'NONE',  ( 3.350143586568126164, 99.50000000000001421, -24.46212657588250394 ) ) ;
#1131=CARTESIAN_POINT ( 'NONE',  ( 4.128176300878408256, 99.50000000000001421, -21.47174600747824869 ) ) ;
#1132=CARTESIAN_POINT ( 'NONE',  ( 3.291601991079349698, 100.0000000000000000, -22.28586332678438353 ) ) ;
#1133=CARTESIAN_POINT ( 'NONE',  ( -11.18376618407356560, 2.449999997815050179, -27.00000000000000355 ) ) ;
#1135=DIRECTION ( 'NONE',  ( 0.000000000000000000, 0.000000000000000000, -1.000000000000000000 ) ) ;
#1136=CARTESIAN_POINT ( 'NONE',  ( 3.374624233514611937, 100.0000000000000284, -23.25900349070959550 ) ) ;
#1137=CARTESIAN_POINT ( 'NONE',  ( -21.86704275050744073, 99.50000000000001421, -11.06111336656620026 ) ) ;
#1139=CARTESIAN_POINT ( 'NONE',  ( 2.837666006185522782, 100.0000000000000000, -22.03040394835428373 ) ) ;
#1144=ADVANCED_FACE ( 'NONE', ( #3679 ), #6862, .T. ) ;
#1145=CARTESIAN_POINT ( 'NONE',  ( -15.07178375341841559, 99.50000000000001421, 15.16157792772069968 ) ) ;
#1146=CARTESIAN_POINT ( 'NONE',  ( 3.058419780146050648, 99.50000000000000000, -23.12871267107006545 ) ) ;
#1147=CARTESIAN_POINT ( 'NONE',  ( 27.43301269999999548, 3.399999998907525356, 11.36312591709337738 ) ) ;
#1148=ADVANCED_FACE ( 'NONE', ( #5825 ), #1834, .T. ) ;
#1149=CARTESIAN_POINT ( 'NONE',  ( -27.43301270000000258, 0.7499999989075251117, -3.359575119402369376E-15 ) ) ;
#1152=CARTESIAN_POINT ( 'NONE',  ( 7.913184448816831029, 100.0000000000000000, 20.09878816755126252 ) ) ;
#1154=ORIENTED_EDGE ( 'NONE', *, *, #69, .T. ) ;
#1155=LINE ( 'NONE', #6800, #9495 ) ;
#1158=CARTESIAN_POINT ( 'NONE',  ( -16.05932294508833280, 99.50000000000000000, 15.21084698918278555 ) ) ;
#1160=EDGE_CURVE ( 'NONE', #3123, #405, #8323, .T. ) ;
#1161=CARTESIAN_POINT ( 'NONE',  ( 9.526533506306627430, 99.99999999999994316, 21.03094362668609207 ) ) ;
#1164=FACE_OUTER_BOUND ( 'NONE', #1230, .T. ) ;
#1166=ORIENTED_EDGE ( 'NONE', *, *, #5394, .T. ) ;
#1167=CARTESIAN_POINT ( 'NONE',  ( -21.94169572595625795, 99.50000000000000000, -9.715372641902229489 ) ) ;
#1168=CARTESIAN_POINT ( 'NONE',  ( 24.93339342948717885, 99.50000000000000000, -1.235376602564102644 ) ) ;
#1169=CARTESIAN_POINT ( 'NONE',  ( 3.573144549190039321, 99.49999999999998579, -23.04580706645134214 ) ) ;
#1171=CARTESIAN_POINT ( 'NONE',  ( -11.18376618407356737, 2.649999999999999467, -27.00000000000000355 ) ) ;
#1173=DIRECTION ( 'NONE',  ( -0.000000000000000000, 1.000000000000000000, -0.000000000000000000 ) ) ;
#1174=ORIENTED_EDGE ( 'NONE', *, *, #1949, .F. ) ;
#1175=CARTESIAN_POINT ( 'NONE',  ( -22.11394672483139701, 100.0000000000000000, -10.91855052283267646 ) ) ;
#1176=CARTESIAN_POINT ( 'NONE',  ( 9.547662139763570366, 99.99999999999997158, 20.94662037603165672 ) ) ;
#1178=B_SPLINE_CURVE_WITH_KNOTS ( 'NONE', 3,
 ( #825, #3417, #973, #8145, #4164, #4901, #7348, #9611, #4118, #7250, #4794, #1747, #6611, #233, #5738, #8189, #7993, #1603, #8927 ),
 .UNSPECIFIED., .F., .F.,
 ( 4, 1, 1, 1, 1, 1, 1, 1, 1, 1, 1, 1, 1, 1, 1, 1, 4 ),
 ( 0.000000000000000000, 0.06463354665699841406, 0.1274839167070160040, 0.1893660780973640267, 0.2502738481868047038, 0.3108090901939400408, 0.3728692346228669741, 0.4358265942208103261, 0.5002515515682643965, 0.5647461136436963125, 0.6273730017603231790, 0.6892793264321037672, 0.7497280364991398827, 0.8111249352628771003, 0.8723480300361200479, 0.9354359082354426480, 1.000000000000000000 ),
 .UNSPECIFIED. ) ;
#1180=CARTESIAN_POINT ( 'NONE',  ( 27.43301270000000258, 5.149999998907525800, 0.000000000000000000 ) ) ;
#1182=CARTESIAN_POINT ( 'NONE',  ( 9.915951879163557692, 99.50000000000002842, 20.63215000232408158 ) ) ;
#1183=CARTESIAN_POINT ( 'NONE',  ( 26.99999999999999645, 4.549999997815051600, 11.18376618407358691 ) ) ;
#1184=VERTEX_POINT ( 'NONE', #9270 ) ;
#1185=CARTESIAN_POINT ( 'NONE',  ( 3.252389375388976323, 99.50000000000004263, -22.22144413113850447 ) ) ;
#1186=CARTESIAN_POINT ( 'NONE',  ( 19.09188309203678813, 3.099999997815050090, -19.09188309203678813 ) ) ;
#1187=LINE ( 'NONE', #2071, #2352 ) ;
#1189=CARTESIAN_POINT ( 'NONE',  ( 3.973150561375555334, 100.0000000000000000, -22.87236500961342855 ) ) ;
#1190=ORIENTED_EDGE ( 'NONE', *, *, #2658, .F. ) ;
#1191=CARTESIAN_POINT ( 'NONE',  ( -4.959819536546781389E-15, 2.799999997815050268, 27.00000000000000355 ) ) ;
#1193=ORIENTED_EDGE ( 'NONE', *, *, #9, .T. ) ;
#1197=CARTESIAN_POINT ( 'NONE',  ( -14.89508182811745662, 99.99999999999995737, 15.38112983991209326 ) ) ;
#1198=CARTESIAN_POINT ( 'NONE',  ( 9.820792995160308791, 100.0000000000000000, 20.21220011423140761 ) ) ;
#1199=CARTESIAN_POINT ( 'NONE',  ( -11.36312591709337383, 3.999999998907525889, 27.43301269999999548 ) ) ;
#1200=ORIENTED_EDGE ( 'NONE', *, *, #2801, .T. ) ;
#1201=VECTOR ( 'NONE', #8870, 1000.000000000000000 ) ;
#1202=CARTESIAN_POINT ( 'NONE',  ( -15.98323291606820362, 99.99999999999998579, 16.64087298452848884 ) ) ;
#1203=CARTESIAN_POINT ( 'NONE',  ( 21.47055288461538325, 100.0000000000000000, -0.7081330128205128860 ) ) ;
#1204=CARTESIAN_POINT ( 'NONE',  ( 3.478562133589548910, 99.99999999999997158, -24.13114810667639532 ) ) ;
#1205=CARTESIAN_POINT ( 'NONE',  ( 8.322475189980043098, 99.50000000000001421, 19.72675386960232657 ) ) ;
#1209=CARTESIAN_POINT ( 'NONE',  ( -27.43301270000000258, 0.6499999989075252449, -3.359575119402369376E-15 ) ) ;
#1210=CIRCLE ( 'NONE', #9577, 25.00000000000000000 ) ;
#1212=CARTESIAN_POINT ( 'NONE',  ( 4.363164797760430424, 100.0000000000000284, -21.67376679147534446 ) ) ;
#1213=DIRECTION ( 'NONE',  ( 0.000000000000000000, 1.000000000000000000, 0.000000000000000000 ) ) ;
#1214=CARTESIAN_POINT ( 'NONE',  ( -16.36254897777739004, 100.0000000000000142, 15.39785597259249350 ) ) ;
#1215=ORIENTED_EDGE ( 'NONE', *, *, #3912, .F. ) ;
#1216=CARTESIAN_POINT ( 'NONE',  ( -16.05266356869597644, 100.0000000000000000, 16.62382211633880047 ) ) ;
#1217=AXIS2_PLACEMENT_3D ( 'NONE', #5160, #5801, #5005 ) ;
#1218=EDGE_CURVE ( 'NONE', #1184, #6802, #8495, .T. ) ;
#1221=ADVANCED_FACE ( 'NONE', ( #752 ), #1677, .T. ) ;
#1222=CARTESIAN_POINT ( 'NONE',  ( 4.640952353770416927, 99.50000000000000000, -24.17064508475253604 ) ) ;
#1223=LINE ( 'NONE', #6032, #5287 ) ;
#1224=CARTESIAN_POINT ( 'NONE',  ( 3.293841816516395848, 99.49999999999998579, -23.44781013845121009 ) ) ;
#1225=CARTESIAN_POINT ( 'NONE',  ( -11.18376618407358336, 3.549999997815050268, 26.99999999999999645 ) ) ;
#1227=LINE ( 'NONE', #8451, #473 ) ;
#1229=CARTESIAN_POINT ( 'NONE',  ( -15.09818093130665773, 100.0000000000000000, 16.69478731934044191 ) ) ;
#1230=EDGE_LOOP ( 'NONE', ( #5144, #5256, #1827, #169, #4560, #2743 ) ) ;
#1232=CARTESIAN_POINT ( 'NONE',  ( -11.36312591709337383, 3.299999998907525267, 27.43301269999999548 ) ) ;
#1234=CARTESIAN_POINT ( 'NONE',  ( -16.88522588321459494, 99.50000000000002842, 16.18266969485829421 ) ) ;
#1235=ORIENTED_EDGE ( 'NONE', *, *, #9720, .F. ) ;
#1236=CARTESIAN_POINT ( 'NONE',  ( 1.679787559701184688E-15, 5.349999998907525089, -27.43301270000000258 ) ) ;
#1237=CARTESIAN_POINT ( 'NONE',  ( 8.536201443755420115, 99.50000000000002842, 19.63502355897212581 ) ) ;
#1238=( BOUNDED_CURVE ( )  B_SPLINE_CURVE ( 2, ( #3288, #3974, #9669, #7206, #38, #9620, #8837, #4858, #8688 ),
 .UNSPECIFIED., .F., .F. ) 
 B_SPLINE_CURVE_WITH_KNOTS ( ( 3, 2, 2, 2, 3 ),
 ( 0.3928571428571428492, 0.4107142857142856984, 0.4285714285714285476, 0.4464285714285714524, 0.4642857142857143016 ),
 .UNSPECIFIED. ) 
 CURVE ( )  GEOMETRIC_REPRESENTATION_ITEM ( )  RATIONAL_B_SPLINE_CURVE ( ( 1.000000000000000000, 0.9238795325112867385, 1.000000000000000000, 0.9238795325112867385, 1.000000000000000000, 0.9238795325112867385, 1.000000000000000000, 0.9238795325112867385, 1.000000000000000000 ) ) 
 REPRESENTATION_ITEM ( '' )  );
#1241=CARTESIAN_POINT ( 'NONE',  ( 3.275092494823534928, 100.0000000000000000, -23.54688978826290580 ) ) ;
#1243=DIRECTION ( 'NONE',  ( 0.000000000000000000, 1.000000000000000000, 0.000000000000000000 ) ) ;
#1244=VECTOR ( 'NONE', #1372, 1000.000000000000000 ) ;
#1245=CARTESIAN_POINT ( 'NONE',  ( 27.43301270000000258, 2.749999998907525445, 0.000000000000000000 ) ) ;
#1249=CARTESIAN_POINT ( 'NONE',  ( 3.311778287470797721, 99.99999999999997158, -21.22295334266859967 ) ) ;
#1251=CARTESIAN_POINT ( 'NONE',  ( 19.39806930854667399, 4.149999998907525800, 19.39806930854668465 ) ) ;
#1252=CARTESIAN_POINT ( 'NONE',  ( -11.36312591709337383, 3.299999998907525267, 27.43301269999999548 ) ) ;
#1254=CARTESIAN_POINT ( 'NONE',  ( 9.820792995160308791, 100.0000000000000000, 20.21220011423140761 ) ) ;
#1255=DIRECTION ( 'NONE',  ( -0.8799640205556051864, 0.000000000000000000, -0.4750403377899757862 ) ) ;
#1256=CARTESIAN_POINT ( 'NONE',  ( 0.000000000000000000, 87.00000000000001421, 0.000000000000000000 ) ) ;
#1258=CARTESIAN_POINT ( 'NONE',  ( 3.428794695218988053, 100.0000000000000142, -24.07607503615978572 ) ) ;
#1259=ADVANCED_BREP_SHAPE_REPRESENTATION ( '', ( #6543, #5055 ), #8584 ) ;
#1265=CARTESIAN_POINT ( 'NONE',  ( -5.039362679103552881E-15, 0.8499999989075252005, 27.43301270000000258 ) ) ;
#1266=CARTESIAN_POINT ( 'NONE',  ( -15.84712739808237103, 99.99999999999994316, 14.83079670662049310 ) ) ;
#1267=CARTESIAN_POINT ( 'NONE',  ( 9.500395184910136237, 99.99999999999994316, 21.12540332933289733 ) ) ;
#1268=CYLINDRICAL_SURFACE ( 'NONE', #3424, 25.00000000000000000 ) ;
#1270=CYLINDRICAL_SURFACE ( 'NONE', #2390, 27.00000000000000355 ) ;
#1273=CARTESIAN_POINT ( 'NONE',  ( -22.06741020400400188, 100.0000000000000142, -9.788922322134999021 ) ) ;
#1276=VECTOR ( 'NONE', #1944, 1000.000000000000000 ) ;
#1277=DIRECTION ( 'NONE',  ( 0.000000000000000000, 1.000000000000000000, 0.000000000000000000 ) ) ;
#1278=CARTESIAN_POINT ( 'NONE',  ( 3.207968951880266761, 99.99999999999998579, -22.92616835434091627 ) ) ;
#1279=ADVANCED_FACE ( 'NONE', ( #3789 ), #4725, .T. ) ;
#1280=VECTOR ( 'NONE', #8827, 1000.000000000000114 ) ;
#1281=CARTESIAN_POINT ( 'NONE',  ( 3.712044765110731337, 99.49999999999998579, -21.08683700305641651 ) ) ;
#1282=CARTESIAN_POINT ( 'NONE',  ( -19.09188309203678457, 1.100000000000000089, -19.09188309203678813 ) ) ;
#1283=DIRECTION ( 'NONE',  ( -0.9804671828129908340, 0.000000000000000000, 0.1966827481675937905 ) ) ;
#1284=ORIENTED_EDGE ( 'NONE', *, *, #911, .F. ) ;
#1286=CARTESIAN_POINT ( 'NONE',  ( -11.36312591709337383, 2.499999998907525445, 27.43301269999999548 ) ) ;
#1288=DIRECTION ( 'NONE',  ( 0.05376826219280737146, 0.000000000000000000, 0.9985534407235125975 ) ) ;
#1290=CARTESIAN_POINT ( 'NONE',  ( -20.89052720883767122, 100.0000000000000000, -9.602653601535816819 ) ) ;
#1291=CARTESIAN_POINT ( 'NONE',  ( 5.240996349771887886, 99.50000000000001421, -23.60769396873743631 ) ) ;
#1293=CARTESIAN_POINT ( 'NONE',  ( -16.54770463920453949, 99.50000000000002842, 15.70234036036222847 ) ) ;
#1295=CARTESIAN_POINT ( 'NONE',  ( -16.63177974700816009, 100.0000000000000000, 16.59747536361813403 ) ) ;
#1296=CARTESIAN_POINT ( 'NONE',  ( 1.679787559701184688E-15, 2.949999998907525178, -27.43301270000000258 ) ) ;
#1301=CARTESIAN_POINT ( 'NONE',  ( 0.000000000000000000, 100.0000000000000000, 0.000000000000000000 ) ) ;
#1302=CARTESIAN_POINT ( 'NONE',  ( 0.000000000000000000, 100.0000000000000000, 0.000000000000000000 ) ) ;
#1303=( BOUNDED_CURVE ( )  B_SPLINE_CURVE ( 2, ( #5578, #3220, #8766, #7238, #4783, #7928, #760, #8866, #4054 ),
 .UNSPECIFIED., .F., .T. ) 
 B_SPLINE_CURVE_WITH_KNOTS ( ( 3, 2, 2, 2, 3 ),
 ( 0.3214285714285714524, 0.3392857142857143016, 0.3571428571428571508, 0.3750000000000000000, 0.3928571428571428492 ),
 .UNSPECIFIED. ) 
 CURVE ( )  GEOMETRIC_REPRESENTATION_ITEM ( )  RATIONAL_B_SPLINE_CURVE ( ( 1.000000000000000000, 0.9238795325112867385, 1.000000000000000000, 0.9238795325112867385, 1.000000000000000000, 0.9238795325112867385, 1.000000000000000000, 0.9238795325112867385, 1.000000000000000000 ) ) 
 REPRESENTATION_ITEM ( '' )  );
#1305=CARTESIAN_POINT ( 'NONE',  ( -16.90689012439429462, 99.49999999999998579, 16.08742389234230785 ) ) ;
#1306=CARTESIAN_POINT ( 'NONE',  ( -27.43301270000000258, 1.499999998907525223, -11.36312591709336317 ) ) ;
#1307=ORIENTED_EDGE ( 'NONE', *, *, #6517, .T. ) ;
#1309=CARTESIAN_POINT ( 'NONE',  ( -15.84712739808237103, 99.99999999999997158, 14.83079670662049310 ) ) ;
#1312=CARTESIAN_POINT ( 'NONE',  ( -16.25072943800822500, 100.0000000000000568, 15.30228603765648820 ) ) ;
#1313=VERTEX_POINT ( 'NONE', #3944 ) ;
#1315=CARTESIAN_POINT ( 'NONE',  ( 2.859712287474666770, 100.0000000000000000, -22.17872625191749236 ) ) ;
#1316=ORIENTED_EDGE ( 'NONE', *, *, #8630, .F. ) ;
#1318=CARTESIAN_POINT ( 'NONE',  ( -27.43301270000000969, 3.099999998907525089, 11.36312591709335429 ) ) ;
#1319=ADVANCED_FACE ( 'NONE', ( #10059 ), #6360, .T. ) ;
#1320=CARTESIAN_POINT ( 'NONE',  ( -15.98658610793439117, 99.50000000000001421, 14.83943845084690949 ) ) ;
#1321=B_SPLINE_CURVE_WITH_KNOTS ( 'NONE', 3,
 ( #4880, #9642, #2476, #5672, #8076, #905, #3311, #7372, #4339, #8370, #7473 ),
 .UNSPECIFIED., .F., .F.,
 ( 4, 1, 1, 1, 1, 1, 1, 1, 4 ),
 ( 0.000000000000000000, 0.09767211715481777246, 0.1989896052561311024, 0.3043518128873296535, 0.4150874769980872347, 0.5363819683935961979, 0.6738601886791220075, 0.8283091006677448798, 1.000000000000000000 ),
 .UNSPECIFIED. ) ;
#1322=CARTESIAN_POINT ( 'NONE',  ( -19.09188309203678457, 1.899999999999999911, -19.09188309203678813 ) ) ;
#1323=CARTESIAN_POINT ( 'NONE',  ( 8.973011566395204142, 99.49999999999997158, 19.93291184930431115 ) ) ;
#1324=EDGE_LOOP ( 'NONE', ( #4697, #1014 ) ) ;
#1327=ORIENTED_EDGE ( 'NONE', *, *, #521, .T. ) ;
#1328=B_SPLINE_CURVE_WITH_KNOTS ( 'NONE', 3,
 ( #1049, #3722, #7800, #5346, #10044, #7580, #7750, #1202, #630, #4445, #4394, #8535, #3614, #6230, #3773, #3669, #8479, #417, #6960 ),
 .UNSPECIFIED., .F., .F.,
 ( 4, 1, 1, 1, 1, 1, 1, 1, 1, 1, 1, 1, 1, 1, 1, 1, 4 ),
 ( 0.000000000000000000, 0.06473117683888822416, 0.1283191082976379849, 0.1900130092022370987, 0.2509653124206144836, 0.3118694605430146760, 0.3735603890354366463, 0.4359106579620777855, 0.5007804971236301528, 0.5656503362851855732, 0.6280858374182423098, 0.6899222460797727052, 0.7510277903999277305, 0.8114330998898260372, 0.8726106248506092511, 0.9357151229638154266, 1.000000000000000000 ),
 .UNSPECIFIED. ) ;
#1329=CYLINDRICAL_SURFACE ( 'NONE', #2785, 25.00000000000000000 ) ;
#1330=CARTESIAN_POINT ( 'NONE',  ( -15.89341924297059094, 100.0000000000000142, 17.07725933521297890 ) ) ;
#1331=DIRECTION ( 'NONE',  ( -0.1697592580069431922, 0.000000000000000000, 0.9854855627156250408 ) ) ;
#1335=CARTESIAN_POINT ( 'NONE',  ( -11.18376618407356737, 3.450000000000000178, -27.00000000000000355 ) ) ;
#1336=CARTESIAN_POINT ( 'NONE',  ( 3.771794781161601939, 99.49999999999998579, -21.07813736596861176 ) ) ;
#1338=CARTESIAN_POINT ( 'NONE',  ( 19.09188309203678813, 0.9000000000000001332, -19.09188309203678813 ) ) ;
#1340=CARTESIAN_POINT ( 'NONE',  ( -21.56977948371741505, 99.49999999999995737, -11.44450812306045329 ) ) ;
#1343=CARTESIAN_POINT ( 'NONE',  ( 9.881472129446523311, 99.50000000000002842, 20.94326683228310060 ) ) ;
#1345=LINE ( 'NONE', #511, #8390 ) ;
#1347=FACE_BOUND ( 'NONE', #8726, .T. ) ;
#1348=ORIENTED_EDGE ( 'NONE', *, *, #8427, .T. ) ;
#1349=CARTESIAN_POINT ( 'NONE',  ( 0.000000000000000000, 97.50000000000000000, 0.000000000000000000 ) ) ;
#1350=CARTESIAN_POINT ( 'NONE',  ( -19.39806930854667755, 3.049999998907525711, -19.39806930854668110 ) ) ;
#1351=ORIENTED_EDGE ( 'NONE', *, *, #4166, .F. ) ;
#1354=CARTESIAN_POINT ( 'NONE',  ( 27.00000000000000355, 0.000000000000000000, 0.000000000000000000 ) ) ;
#1355=FACE_OUTER_BOUND ( 'NONE', #8614, .T. ) ;
#1357=CARTESIAN_POINT ( 'NONE',  ( -16.60513711880302878, 99.50000000000000000, 15.15667007515659570 ) ) ;
#1358=CARTESIAN_POINT ( 'NONE',  ( -27.43301270000000258, 3.149999998907524912, -3.359575119402369376E-15 ) ) ;
#1359=ORIENTED_EDGE ( 'NONE', *, *, #8169, .F. ) ;
#1360=CARTESIAN_POINT ( 'NONE',  ( 9.445361748092775400, 100.0000000000000142, 19.75398588445988324 ) ) ;
#1362=CARTESIAN_POINT ( 'NONE',  ( 7.486453019397995234, 100.0000000000000000, 23.81666162955709964 ) ) ;
#1366=VERTEX_POINT ( 'NONE', #4775 ) ;
#1369=CARTESIAN_POINT ( 'NONE',  ( -27.43301270000000258, 3.849999998907525534, -3.359575119402369376E-15 ) ) ;
#1371=VERTEX_POINT ( 'NONE', #6400 ) ;
#1372=DIRECTION ( 'NONE',  ( -0.000000000000000000, -1.000000000000000000, -0.000000000000000000 ) ) ;
#1373=VECTOR ( 'NONE', #9662, 999.9999999999998863 ) ;
#1374=CARTESIAN_POINT ( 'NONE',  ( 19.09188309203678813, 1.700000000000000178, -19.09188309203678813 ) ) ;
#1377=ORIENTED_EDGE ( 'NONE', *, *, #9704, .F. ) ;
#1378=CARTESIAN_POINT ( 'NONE',  ( -16.37951318544778445, 99.99999999999994316, 15.41600550949200077 ) ) ;
#1379=CARTESIAN_POINT ( 'NONE',  ( -15.33577160963320374, 99.49999999999998579, 16.45272793336155814 ) ) ;
#1382=ORIENTED_EDGE ( 'NONE', *, *, #8246, .F. ) ;
#1384=DIRECTION ( 'NONE',  ( -0.000000000000000000, 1.000000000000000000, -0.000000000000000000 ) ) ;
#1387=CARTESIAN_POINT ( 'NONE',  ( 5.179363668139080445, 100.0000000000000995, -23.94265746362379943 ) ) ;
#1388=CARTESIAN_POINT ( 'NONE',  ( 4.446585460023182890, 100.0000000000000000, -21.79057454014859019 ) ) ;
#1389=ADVANCED_FACE ( 'NONE', ( #66 ), #9591, .T. ) ;
#1391=CARTESIAN_POINT ( 'NONE',  ( 4.691018317478480526, 99.49999999999995737, -21.52316599815148024 ) ) ;
#1392=VERTEX_POINT ( 'NONE', #7281 ) ;
#1393=CARTESIAN_POINT ( 'NONE',  ( 3.375079225685456041, 99.50000000000000000, -22.79123997459842954 ) ) ;
#1399=ORIENTED_EDGE ( 'NONE', *, *, #9313, .F. ) ;
#1401=CARTESIAN_POINT ( 'NONE',  ( 9.063633472794011325, 99.49999999999998579, 19.59517414759687526 ) ) ;
#1404=FACE_BOUND ( 'NONE', #10064, .T. ) ;
#1406=CARTESIAN_POINT ( 'NONE',  ( -16.42071764973191250, 99.50000000000001421, 16.76105279315999042 ) ) ;
#1408=ORIENTED_EDGE ( 'NONE', *, *, #8045, .T. ) ;
#1412=ADVANCED_FACE ( 'NONE', ( #2422 ), #8859, .T. ) ;
#1413=CARTESIAN_POINT ( 'NONE',  ( -20.96643530928959365, 99.50000000000000000, -10.05541671241504886 ) ) ;
#1414=CARTESIAN_POINT ( 'NONE',  ( -5.039362679103552881E-15, 1.749999998907525223, 27.43301270000000258 ) ) ;
#1415=ORIENTED_EDGE ( 'NONE', *, *, #6754, .T. ) ;
#1418=CARTESIAN_POINT ( 'NONE',  ( 9.164845778125666698, 100.0000000000000142, 19.62003801130714820 ) ) ;
#1420=CARTESIAN_POINT ( 'NONE',  ( 3.198738776810544415, 99.50000000000001421, -22.02447230026614022 ) ) ;
#1422=CARTESIAN_POINT ( 'NONE',  ( -15.37731512048643268, 100.0000000000000000, 15.34394520743122214 ) ) ;
#1423=ORIENTED_EDGE ( 'NONE', *, *, #2005, .T. ) ;
#1425=CARTESIAN_POINT ( 'NONE',  ( 4.570993444255353921, 99.99999999999998579, -21.37574484917381668 ) ) ;
#1426=ORIENTED_EDGE ( 'NONE', *, *, #10127, .F. ) ;
#1428=CARTESIAN_POINT ( 'NONE',  ( 27.43301270000000258, 2.649999998907525356, 0.000000000000000000 ) ) ;
#1429=CARTESIAN_POINT ( 'NONE',  ( 1.662111305799679408E-15, 5.083333332969175444, -27.14433756666667108 ) ) ;
#1430=CARTESIAN_POINT ( 'NONE',  ( -11.18376618407356560, 0.2500000000000000000, -27.00000000000000355 ) ) ;
#1431=CARTESIAN_POINT ( 'NONE',  ( 6.477538756577482459, 99.50000000000000000, 20.49684993083915430 ) ) ;
#1432=ORIENTED_EDGE ( 'NONE', *, *, #294, .F. ) ;
#1433=VECTOR ( 'NONE', #8642, 1000.000000000000000 ) ;
#1434=CARTESIAN_POINT ( 'NONE',  ( 24.91446314102564230, 99.50000000000000000, -1.581029647435897578 ) ) ;
#1435=CARTESIAN_POINT ( 'NONE',  ( 8.063732359723156051, 100.0000000000000142, 20.72384750152746236 ) ) ;
#1436=( BOUNDED_CURVE ( )  B_SPLINE_CURVE ( 2, ( #817, #3322, #8871, #223, #2539, #3408, #4841, #5732, #7985 ),
 .UNSPECIFIED., .F., .T. ) 
 B_SPLINE_CURVE_WITH_KNOTS ( ( 3, 2, 2, 2, 3 ),
 ( 0.2500000000000000000, 0.2678571428571428492, 0.2857142857142856984, 0.3035714285714285476, 0.3214285714285714524 ),
 .UNSPECIFIED. ) 
 CURVE ( )  GEOMETRIC_REPRESENTATION_ITEM ( )  RATIONAL_B_SPLINE_CURVE ( ( 1.000000000000000000, 0.9238795325112867385, 1.000000000000000000, 0.9238795325112867385, 1.000000000000000000, 0.9238795325112867385, 1.000000000000000000, 0.9238795325112867385, 1.000000000000000000 ) ) 
 REPRESENTATION_ITEM ( '' )  );
#1438=VERTEX_POINT ( 'NONE', #8167 ) ;
#1440=CARTESIAN_POINT ( 'NONE',  ( -15.72775836928289017, 100.0000000000000000, 17.03252426573849476 ) ) ;
#1441=CARTESIAN_POINT ( 'NONE',  ( -21.00001322343447541, 99.50000000000001421, -9.990026185521596602 ) ) ;
#1443=CARTESIAN_POINT ( 'NONE',  ( -27.00000000000000355, 3.549999999999999822, -11.18376618407357270 ) ) ;
#1445=CARTESIAN_POINT ( 'NONE',  ( 3.681717055787076642, 100.0000000000000000, -21.09125273517263111 ) ) ;
#1447=CARTESIAN_POINT ( 'NONE',  ( 3.058419780146050648, 99.50000000000000000, -23.12871267107006545 ) ) ;
#1449=ORIENTED_EDGE ( 'NONE', *, *, #6403, .T. ) ;
#1453=EDGE_CURVE ( 'NONE', #9675, #4732, #1321, .T. ) ;
#1454=VERTEX_POINT ( 'NONE', #7421 ) ;
#1455=PLANE ( 'NONE',  #93 ) ;
#1456=AXIS2_PLACEMENT_3D ( 'NONE', #7770, #2109, #8615 ) ;
#1463=CARTESIAN_POINT ( 'NONE',  ( 9.182805720491336032, 100.0000000000000000, 20.00174565872165289 ) ) ;
#1468=CARTESIAN_POINT ( 'NONE',  ( 4.803433990161294354, 99.50000000000001421, -23.96838578116891583 ) ) ;
#1469=CARTESIAN_POINT ( 'NONE',  ( -19.39806930854668465, 1.649999998907525356, 19.39806930854667755 ) ) ;
#1470=VERTEX_POINT ( 'NONE', #4240 ) ;
#1473=CARTESIAN_POINT ( 'NONE',  ( 2.940631318607589417, 99.50000000000000000, -23.77584808773673331 ) ) ;
#1475=CARTESIAN_POINT ( 'NONE',  ( 3.948639947730041566, 99.49999999999998579, -21.07692942975820927 ) ) ;
#1476=ORIENTED_EDGE ( 'NONE', *, *, #2750, .F. ) ;
#1477=EDGE_CURVE ( 'NONE', #7818, #1371, #1027, .T. ) ;
#1479=CARTESIAN_POINT ( 'NONE',  ( 11.36312591709336850, 3.299999998907525711, 27.43301269999999903 ) ) ;
#1481=CARTESIAN_POINT ( 'NONE',  ( 3.061616997868383043E-15, 100.0000000000000000, 25.00000000000000000 ) ) ;
#1482=CARTESIAN_POINT ( 'NONE',  ( -4.959819536546781389E-15, 1.399999999999999911, 27.00000000000000355 ) ) ;
#1484=CARTESIAN_POINT ( 'NONE',  ( 8.612131858919537919, 99.49999999999998579, 19.96100069886393413 ) ) ;
#1485=VERTEX_POINT ( 'NONE', #9202 ) ;
#1486=CARTESIAN_POINT ( 'NONE',  ( -16.40919047799676989, 99.50000000000000000, 16.38364531277195013 ) ) ;
#1487=CARTESIAN_POINT ( 'NONE',  ( 8.064245308217579122, 99.99999999999998579, 20.64099956338070641 ) ) ;
#1490=VERTEX_POINT ( 'NONE', #3450 ) ;
#1491=CARTESIAN_POINT ( 'NONE',  ( 27.43301270000000258, 1.849999998907525534, 0.000000000000000000 ) ) ;
#1493=EDGE_CURVE ( 'NONE', #4732, #7023, #9993, .T. ) ;
#1495=CARTESIAN_POINT ( 'NONE',  ( 5.226890989224467710, 99.50000000000000000, -23.72545275563321354 ) ) ;
#1496=DIRECTION ( 'NONE',  ( 0.000000000000000000, 1.000000000000000000, 0.000000000000000000 ) ) ;
#1497=EDGE_LOOP ( 'NONE', ( #1377, #2001, #3588, #479 ) ) ;
#1499=CARTESIAN_POINT ( 'NONE',  ( 4.739008722453743161, 100.0000000000000142, -24.06821587619827341 ) ) ;
#1504=B_SPLINE_SURFACE_WITH_KNOTS ( 'NONE', 3, 1, ( 
 ( #10232, #7133 ),
 ( #2425, #4972 ),
 ( #8811, #2576 ),
 ( #9691, #5769 ),
 ( #8909, #1689 ),
 ( #6548, #1051 ),
 ( #7333, #2621 ),
 ( #6402, #3356 ),
 ( #5816, #68 ),
 ( #2531, #5724 ),
 ( #4193, #1640 ),
 ( #8172, #6594 ),
 ( #4885, #9784 ),
 ( #15, #168 ),
 ( #6455, #9005 ),
 ( #2479, #9644 ),
 ( #3313, #3217 ),
 ( #1000, #9738 ),
 ( #8125, #1826 ) ),
 .UNSPECIFIED., .F., .F., .F.,
 ( 4, 1, 1, 1, 1, 1, 1, 1, 1, 1, 1, 1, 1, 1, 1, 1, 4 ),
 ( 2, 2 ),
 ( 0.000000000000000000, 0.06455295689170470474, 0.1273249605695649933, 0.1891299628201091876, 0.2499617887110622549, 0.3104215510145779122, 0.3717966107350694216, 0.4346754705585744727, 0.4991966429079077727, 0.5636107885140392293, 0.6264421791528413941, 0.6882713145562978641, 0.7491215306807221808, 0.8100115732567139126, 0.8716292230916812267, 0.9349778748807419104, 1.000000000000000000 ),
 ( 0.000000000000000000, 1.000000000000000000 ),
 .UNSPECIFIED. ) ;
#1505=CARTESIAN_POINT ( 'NONE',  ( 8.685676809262872666, 100.0000000000000000, 23.43455588346217766 ) ) ;
#1506=CARTESIAN_POINT ( 'NONE',  ( 9.806436918512124734, 99.49999999999998579, 20.18080982695387604 ) ) ;
#1510=CARTESIAN_POINT ( 'NONE',  ( -19.09188309203678457, 2.499999997815050445, -19.09188309203678813 ) ) ;
#1511=CARTESIAN_POINT ( 'NONE',  ( 1.679787559701184688E-15, 5.349999998907525089, -27.43301270000000258 ) ) ;
#1512=ORIENTED_EDGE ( 'NONE', *, *, #4929, .T. ) ;
#1515=CARTESIAN_POINT ( 'NONE',  ( 3.275092494823534928, 99.99999999999997158, -23.54688978826290580 ) ) ;
#1517=CARTESIAN_POINT ( 'NONE',  ( 3.764204346677844093, 99.50000000000001421, -22.52576385118515745 ) ) ;
#1518=CARTESIAN_POINT ( 'NONE',  ( 11.18376618407356915, 1.549999997815050490, -27.00000000000000355 ) ) ;
#1519=CARTESIAN_POINT ( 'NONE',  ( -15.31787750341841559, 99.99999999999997158, 16.43551622900274722 ) ) ;
#1521=CARTESIAN_POINT ( 'NONE',  ( 3.198592217420132666, 99.50000000000000000, -21.96964977087737836 ) ) ;
#1523=CARTESIAN_POINT ( 'NONE',  ( -22.67341330918043951, 100.0000000000000000, -10.57563951594260665 ) ) ;
#1525=CARTESIAN_POINT ( 'NONE',  ( -20.74358258379034936, 99.49999999999998579, -9.818556592845180120 ) ) ;
#1526=ORIENTED_EDGE ( 'NONE', *, *, #2961, .T. ) ;
#1528=CARTESIAN_POINT ( 'NONE',  ( 1.679787559701184688E-15, 1.349999998907525312, -27.43301270000000258 ) ) ;
#1529=CARTESIAN_POINT ( 'NONE',  ( -16.56926954694585774, 99.50000000000001421, 15.12296757606276643 ) ) ;
#1530=LINE ( 'NONE', #6916, #2591 ) ;
#1533=CARTESIAN_POINT ( 'NONE',  ( 8.231219904624582639, 100.0000000000000000, 20.21381436664452735 ) ) ;
#1534=EDGE_LOOP ( 'NONE', ( #5350, #1415, #3867, #444 ) ) ;
#1537=CARTESIAN_POINT ( 'NONE',  ( -19.39806930854668465, 1.549999998907525489, 19.39806930854667755 ) ) ;
#1538=AXIS2_PLACEMENT_3D ( 'NONE', #3330, #9755, #7201 ) ;
#1539=CARTESIAN_POINT ( 'NONE',  ( 3.977571997893210032, 99.50000000000000000, -24.70179182097838932 ) ) ;
#1540=AXIS2_PLACEMENT_3D ( 'NONE', #7523, #2829, #6010 ) ;
#1544=CARTESIAN_POINT ( 'NONE',  ( 9.834295043520187463, 100.0000000000000142, 21.14079655679390513 ) ) ;
#1548=VECTOR ( 'NONE', #7489, 1000.000000000000000 ) ;
#1554=CARTESIAN_POINT ( 'NONE',  ( 8.465276868207817884, 99.50000000000001421, 19.66343818277063704 ) ) ;
#1556=VECTOR ( 'NONE', #6322, 1000.000000000000000 ) ;
#1557=ORIENTED_EDGE ( 'NONE', *, *, #9087, .T. ) ;
#1558=CARTESIAN_POINT ( 'NONE',  ( 3.016803124593948393, 99.50000000000001421, -23.20507807535735978 ) ) ;
#1559=FACE_OUTER_BOUND ( 'NONE', #5044, .T. ) ;
#1560=CARTESIAN_POINT ( 'NONE',  ( -22.35673484330673944, 99.50000000000001421, -10.41320610523044721 ) ) ;
#1561=DIRECTION ( 'NONE',  ( -0.05417351272771728926, 0.000000000000000000, -0.9985315370676781654 ) ) ;
#1562=CARTESIAN_POINT ( 'NONE',  ( 19.39806930854667399, 5.049999998907525267, 19.39806930854668465 ) ) ;
#1563=ORIENTED_EDGE ( 'NONE', *, *, #8450, .T. ) ;
#1566=CARTESIAN_POINT ( 'NONE',  ( 3.477525819554967423, 100.0000000000000000, -22.44236894434852658 ) ) ;
#1568=CARTESIAN_POINT ( 'NONE',  ( -20.42657152723830905, 99.50000000000000000, -10.54129411626120216 ) ) ;
#1569=CARTESIAN_POINT ( 'NONE',  ( -19.09188309203678457, 0.8999999978150503566, -19.09188309203678813 ) ) ;
#1571=LINE ( 'NONE', #3202, #100 ) ;
#1573=CARTESIAN_POINT ( 'NONE',  ( 3.283294465904739390, 100.0000000000000284, -21.71066637097430885 ) ) ;
#1574=CARTESIAN_POINT ( 'NONE',  ( 1.653273178848927064E-15, 4.200000000000000178, -27.00000000000000355 ) ) ;
#1576=CARTESIAN_POINT ( 'NONE',  ( -21.30033281797529909, 99.50000000000002842, -9.345151174687854834 ) ) ;
#1578=CARTESIAN_POINT ( 'NONE',  ( -19.39806930854667755, 1.449999998907525178, -19.39806930854668110 ) ) ;
#1579=CARTESIAN_POINT ( 'NONE',  ( -15.58193289918752278, 99.50000000000000000, 16.98546238400348329 ) ) ;
#1580=EDGE_CURVE ( 'NONE', #2567, #5889, #5964, .T. ) ;
#1581=CARTESIAN_POINT ( 'NONE',  ( -11.36312591709335962, 0.4999999989075252227, -27.43301270000000258 ) ) ;
#1582=DIRECTION ( 'NONE',  ( -0.9200099868272721970, 0.000000000000000000, 0.3918949146621865665 ) ) ;
#1586=CARTESIAN_POINT ( 'NONE',  ( 8.515772100368442565, 100.0000000000000000, 20.00046577258137503 ) ) ;
#1589=ORIENTED_EDGE ( 'NONE', *, *, #5244, .F. ) ;
#1590=CARTESIAN_POINT ( 'NONE',  ( 27.43301270000000258, 2.699999998907525178, -11.36312591709336139 ) ) ;
#1593=CARTESIAN_POINT ( 'NONE',  ( -21.84904385032055174, 99.99999999999998579, -11.42736543092427404 ) ) ;
#1595=CARTESIAN_POINT ( 'NONE',  ( 10.72103337977569204, 99.50000000000000000, 22.20268488987243316 ) ) ;
#1596=EDGE_CURVE ( 'NONE', #2682, #3764, #6034, .T. ) ;
#1597=CARTESIAN_POINT ( 'NONE',  ( -16.92301558088953328, 99.50000000000001421, 15.88693424423437683 ) ) ;
#1598=CARTESIAN_POINT ( 'NONE',  ( 8.399337394135656609, 99.99999999999998579, 20.06291166101774692 ) ) ;
#1599=ADVANCED_FACE ( 'NONE', ( #3501 ), #6702, .F. ) ;
#1603=CARTESIAN_POINT ( 'NONE',  ( -22.27115127098604574, 99.50000000000000000, -10.71048520281369676 ) ) ;
#1604=VECTOR ( 'NONE', #8608, 1000.000000000000000 ) ;
#1606=EDGE_CURVE ( 'NONE', #10071, #1699, #2548, .T. ) ;
#1607=CARTESIAN_POINT ( 'NONE',  ( 2.940631318607589417, 99.50000000000000000, -23.77584808773673331 ) ) ;
#1608=ORIENTED_EDGE ( 'NONE', *, *, #2676, .T. ) ;
#1609=EDGE_CURVE ( 'NONE', #5515, #10090, #5990, .T. ) ;
#1611=CYLINDRICAL_SURFACE ( 'NONE', #6134, 27.00000000000000355 ) ;
#1612=CARTESIAN_POINT ( 'NONE',  ( 19.39806930854668110, 3.649999998907525356, -19.39806930854668110 ) ) ;
#1615=EDGE_CURVE ( 'NONE', #8551, #463, #1345, .T. ) ;
#1616=VECTOR ( 'NONE', #3577, 999.9999999999998863 ) ;
#1617=CARTESIAN_POINT ( 'NONE',  ( 3.328702480760086235, 99.99999999999994316, -23.35145716610488975 ) ) ;
#1619=FACE_OUTER_BOUND ( 'NONE', #10298, .T. ) ;
#1620=CARTESIAN_POINT ( 'NONE',  ( 1.653273178848927064E-15, 0.7999999978150503788, -27.00000000000000355 ) ) ;
#1621=CARTESIAN_POINT ( 'NONE',  ( -20.64578974631102426, 99.99999999999995737, -10.10077944494247504 ) ) ;
#1624=CARTESIAN_POINT ( 'NONE',  ( 3.478562133589548910, 99.49999999999997158, -24.13114810667639532 ) ) ;
#1625=CARTESIAN_POINT ( 'NONE',  ( 3.399971579580567393, 100.0000000000000000, -21.57509867787664248 ) ) ;
#1626=CARTESIAN_POINT ( 'NONE',  ( 11.18376618407357093, 4.150000000000000355, -27.00000000000000355 ) ) ;
#1627=AXIS2_PLACEMENT_3D ( 'NONE', #8028, #9044, #4280 ) ;
#1629=DIRECTION ( 'NONE',  ( -0.000000000000000000, 1.000000000000000000, -0.000000000000000000 ) ) ;
#1633=CARTESIAN_POINT ( 'NONE',  ( 11.36312591709336139, 5.199999998907525622, -27.43301270000000258 ) ) ;
#1634=LINE ( 'NONE', #3212, #6445 ) ;
#1635=CARTESIAN_POINT ( 'NONE',  ( 11.36312591709336850, 0.8999999989075253559, 27.43301269999999903 ) ) ;
#1636=CARTESIAN_POINT ( 'NONE',  ( 3.028692941384139026, 99.50000000000001421, -22.52214499033115302 ) ) ;
#1638=EDGE_LOOP ( 'NONE', ( #10223, #2329, #1348, #5031 ) ) ;
#1640=CARTESIAN_POINT ( 'NONE',  ( -20.96129225301843135, 99.99999999999998579, -10.68089388303413934 ) ) ;
#1641=EDGE_CURVE ( 'NONE', #827, #2600, #3703, .T. ) ;
#1642=FACE_OUTER_BOUND ( 'NONE', #3861, .T. ) ;
#1643=ORIENTED_EDGE ( 'NONE', *, *, #8965, .F. ) ;
#1644=CARTESIAN_POINT ( 'NONE',  ( -19.39806930854668465, 3.149999998907525356, 19.39806930854667755 ) ) ;
#1645=CARTESIAN_POINT ( 'NONE',  ( 2.940631318607589417, 100.0000000000000000, -23.77584808773673331 ) ) ;
#1646=FACE_OUTER_BOUND ( 'NONE', #2819, .T. ) ;
#1647=( GEOMETRIC_REPRESENTATION_CONTEXT ( 3 ) GLOBAL_UNCERTAINTY_ASSIGNED_CONTEXT ( ( #7169 ) ) GLOBAL_UNIT_ASSIGNED_CONTEXT ( ( #1688, #4831, #7184 ) ) REPRESENTATION_CONTEXT ( 'NONE', 'WORKASPACE' ) );
#1650=CARTESIAN_POINT ( 'NONE',  ( -16.90147242988460263, 99.99999999999998579, 15.68472263728856753 ) ) ;
#1653=AXIS2_PLACEMENT_3D ( 'NONE', #458, #3760, #4535 ) ;
#1656=CARTESIAN_POINT ( 'NONE',  ( 4.743081672682207817, 100.0000000000000284, -21.60795120912350598 ) ) ;
#1658=CARTESIAN_POINT ( 'NONE',  ( 9.526349065647009340, 99.50000000000000000, 19.81320455978211470 ) ) ;
#1660=EDGE_LOOP ( 'NONE', ( #8586, #567, #5060, #187 ) ) ;
#1664=CARTESIAN_POINT ( 'NONE',  ( 24.93339342948717885, 99.50000000000000000, -1.235376602564102644 ) ) ;
#1665=CARTESIAN_POINT ( 'NONE',  ( 8.973011566395204142, 99.99999999999997158, 19.93291184930431115 ) ) ;
#1666=ORIENTED_EDGE ( 'NONE', *, *, #5442, .F. ) ;
#1667=B_SPLINE_CURVE_WITH_KNOTS ( 'NONE', 3,
 ( #331, #7438, #3522, #8187, #8975, #4257, #5034, #5736, #1117, #9022, #3326, #6659, #1015, #2638, #6707 ),
 .UNSPECIFIED., .F., .F.,
 ( 4, 1, 1, 1, 1, 1, 1, 1, 1, 1, 1, 1, 4 ),
 ( 0.000000000000000000, 0.08450893420292937552, 0.1670077533940913517, 0.2489527561816328172, 0.3323249201989921797, 0.4152786837838207679, 0.4972150204155297848, 0.5791806016509544186, 0.6636863847498374325, 0.7483757861910059761, 0.8320455266939520422, 0.9153409992114193150, 1.000000000000000000 ),
 .UNSPECIFIED. ) ;
#1668=CARTESIAN_POINT ( 'NONE',  ( 3.080354370726382296, 99.50000000000004263, -23.09295995363041598 ) ) ;
#1669=FACE_OUTER_BOUND ( 'NONE', #10289, .T. ) ;
#1671=CARTESIAN_POINT ( 'NONE',  ( -20.89169796687544789, 99.50000000000001421, -10.40078880447404330 ) ) ;
#1672=CARTESIAN_POINT ( 'NONE',  ( -19.09188309203678457, 1.699999997815050401, -19.09188309203678813 ) ) ;
#1674=CARTESIAN_POINT ( 'NONE',  ( -15.32348647777738826, 99.50000000000000000, 15.39505148541300450 ) ) ;
#1676=CARTESIAN_POINT ( 'NONE',  ( 3.202955020264580899, 100.0000000000000000, -21.91595956354277064 ) ) ;
#1677=B_SPLINE_SURFACE_WITH_KNOTS ( 'NONE', 3, 1, ( 
 ( #7079, #7867 ),
 ( #7919, #646 ),
 ( #7817, #7706 ),
 ( #2160, #6135 ),
 ( #9498, #3841 ),
 ( #2272, #9386 ),
 ( #5521, #9329 ),
 ( #10284, #2895 ),
 ( #7763, #3061 ),
 ( #4625, #6244 ),
 ( #7026, #5470 ),
 ( #1323, #542 ),
 ( #10229, #5361 ),
 ( #6300, #2322 ),
 ( #9444, #2103 ),
 ( #8550, #3735 ),
 ( #1484, #2215 ),
 ( #4678, #6917 ),
 ( #697, #5418 ) ),
 .UNSPECIFIED., .F., .F., .F.,
 ( 4, 1, 1, 1, 1, 1, 1, 1, 1, 1, 1, 1, 1, 1, 1, 1, 4 ),
 ( 2, 2 ),
 ( 0.000000000000000000, 0.06222907146265880401, 0.1227741760084055250, 0.1821991178386986321, 0.2415152369242211383, 0.3014228132391471027, 0.3622599083280184651, 0.4248173832850619669, 0.4890434280230284148, 0.5537961591902206271, 0.6173286602167864512, 0.6798064121185800612, 0.7417947397634444551, 0.8039614856828293243, 0.8674939867093949264, 0.9325113003366737319, 1.000000000000000000 ),
 ( 0.000000000000000000, 1.000000000000000000 ),
 .UNSPECIFIED. ) ;
#1678=ADVANCED_FACE ( 'NONE', ( #2009 ), #7944, .T. ) ;
#1679=CARTESIAN_POINT ( 'NONE',  ( -22.57971655928959365, 100.0000000000000000, -10.84768434062017839 ) ) ;
#1682=ORIENTED_EDGE ( 'NONE', *, *, #8100, .T. ) ;
#1684=CARTESIAN_POINT ( 'NONE',  ( -27.43301270000000969, 4.699999998907524734, 11.36312591709335429 ) ) ;
#1686=CARTESIAN_POINT ( 'NONE',  ( 27.00000000000000355, 3.250000000000000444, -11.18376618407356737 ) ) ;
#1688=( LENGTH_UNIT ( ) NAMED_UNIT ( * ) SI_UNIT ( .MILLI., .METRE. ) );
#1689=CARTESIAN_POINT ( 'NONE',  ( -20.89948324804827706, 99.99999999999998579, -10.26098411820691858 ) ) ;
#1690=CARTESIAN_POINT ( 'NONE',  ( -20.74358258379034936, 99.49999999999998579, -9.818556592845180120 ) ) ;
#1691=CARTESIAN_POINT ( 'NONE',  ( 19.39806930854668110, 2.749999998907525001, -19.39806930854668110 ) ) ;
#1692=CARTESIAN_POINT ( 'NONE',  ( 3.293272160652527258, 99.99999999999997158, -24.41359064397622802 ) ) ;
#1695=CARTESIAN_POINT ( 'NONE',  ( -16.45391695211397831, 100.0000000000000426, 16.32580124622701589 ) ) ;
#1696=CARTESIAN_POINT ( 'NONE',  ( -16.91946509138130139, 100.0000000000000142, 15.98858002463268413 ) ) ;
#1697=CARTESIAN_POINT ( 'NONE',  ( 5.242860087038358152, 100.0000000000000284, -23.52699316036146371 ) ) ;
#1699=VERTEX_POINT ( 'NONE', #8165 ) ;
#1700=CARTESIAN_POINT ( 'NONE',  ( -22.31230063665282515, 99.49999999999997158, -10.62159318200525249 ) ) ;
#1701=CARTESIAN_POINT ( 'NONE',  ( -15.24337324910153946, 99.49999999999997158, 16.81353386054630761 ) ) ;
#1707=B_SPLINE_CURVE_WITH_KNOTS ( 'NONE', 3,
 ( #8049, #3975, #884, #7159, #9670, #2453, #4074, #97, #1463, #5649, #8838, #1665, #4859, #3289, #3869, #9714, #7309, #6525, #2555 ),
 .UNSPECIFIED., .F., .F.,
 ( 4, 1, 1, 1, 1, 1, 1, 1, 1, 1, 1, 1, 1, 1, 1, 1, 4 ),
 ( 0.000000000000000000, 0.06222907146265880401, 0.1227741760084055250, 0.1821991178386986321, 0.2415152369242211383, 0.3014228132391471027, 0.3622599083280184651, 0.4248173832850619669, 0.4890434280230284148, 0.5537961591902206271, 0.6173286602167864512, 0.6798064121185800612, 0.7417947397634444551, 0.8039614856828293243, 0.8674939867093949264, 0.9325113003366737319, 1.000000000000000000 ),
 .UNSPECIFIED. ) ;
#1708=CARTESIAN_POINT ( 'NONE',  ( 27.00000000000000355, 0.2999999989075251561, 0.000000000000000000 ) ) ;
#1710=LINE ( 'NONE', #10308, #9489 ) ;
#1711=CARTESIAN_POINT ( 'NONE',  ( 1.653273178848927064E-15, 4.200000000000000178, -27.00000000000000355 ) ) ;
#1714=CARTESIAN_POINT ( 'NONE',  ( -21.18296228862668329, 100.0000000000000284, -10.95406920104765724 ) ) ;
#1716=EDGE_CURVE ( 'NONE', #4040, #10122, #5117, .T. ) ;
#1717=EDGE_LOOP ( 'NONE', ( #8594, #6345, #1476, #878 ) ) ;
#1718=CARTESIAN_POINT ( 'NONE',  ( 3.986298408513477387, 99.50000000000002842, -22.53092616755505162 ) ) ;
#1719=CARTESIAN_POINT ( 'NONE',  ( -11.18376618407356560, 0.8499999978150503122, -27.00000000000000355 ) ) ;
#1721=DIRECTION ( 'NONE',  ( -0.5137073458062109133, 0.000000000000000000, -0.8579654788304353907 ) ) ;
#1722=AXIS2_PLACEMENT_3D ( 'NONE', #10052, #6803, #8544 ) ;
#1723=CARTESIAN_POINT ( 'NONE',  ( -4.959819536546781389E-15, 3.599999997815050534, 27.00000000000000355 ) ) ;
#1724=CARTESIAN_POINT ( 'NONE',  ( 3.717146347979291665, 100.0000000000000000, -21.42716062222556417 ) ) ;
#1725=CARTESIAN_POINT ( 'NONE',  ( 5.243816414761435674, 100.0000000000000000, -23.48558366465980995 ) ) ;
#1729=ADVANCED_FACE ( 'NONE', ( #1972 ), #5608, .T. ) ;
#1730=CARTESIAN_POINT ( 'NONE',  ( -15.70584307919286893, 99.50000000000000000, 14.84247401567675162 ) ) ;
#1731=EDGE_CURVE ( 'NONE', #7666, #2013, #1770, .T. ) ;
#1732=CARTESIAN_POINT ( 'NONE',  ( -19.39806930854667755, 0.5499999989075252671, -19.39806930854668110 ) ) ;
#1733=CARTESIAN_POINT ( 'NONE',  ( 2.912748042341355870, 99.99999999999998579, -22.34826719014139940 ) ) ;
#1734=CARTESIAN_POINT ( 'NONE',  ( 27.00000000000000355, 2.199999997815050623, 0.000000000000000000 ) ) ;
#1735=ORIENTED_EDGE ( 'NONE', *, *, #5028, .F. ) ;
#1736=CARTESIAN_POINT ( 'NONE',  ( 4.241330131419338123, 99.99999999999998579, -24.68798891778770965 ) ) ;
#1739=CARTESIAN_POINT ( 'NONE',  ( 4.232798786556307036, 100.0000000000000000, -24.34936571594186105 ) ) ;
#1740=CARTESIAN_POINT ( 'NONE',  ( -22.08823018108446234, 100.0000000000000000, -9.406177930363766038 ) ) ;
#1741=CARTESIAN_POINT ( 'NONE',  ( 8.067960508813904141, 100.0000000000000000, 20.80952186068213905 ) ) ;
#1744=ORIENTED_EDGE ( 'NONE', *, *, #6056, .T. ) ;
#1746=CARTESIAN_POINT ( 'NONE',  ( 3.283294465904739390, 99.50000000000002842, -21.71066637097430885 ) ) ;
#1747=CARTESIAN_POINT ( 'NONE',  ( -21.99951964646687941, 99.50000000000001421, -11.00094659099690553 ) ) ;
#1750=DIRECTION ( 'NONE',  ( -1.000000000000000000, 1.320207234900709352E-11, 0.000000000000000000 ) ) ;
#1752=EDGE_CURVE ( 'NONE', #5272, #4302, #8212, .T. ) ;
#1756=CARTESIAN_POINT ( 'NONE',  ( 3.374624233514611937, 100.0000000000000000, -23.25900349070959550 ) ) ;
#1757=CARTESIAN_POINT ( 'NONE',  ( 3.739209042966564311, 99.50000000000001421, -21.42288334414699591 ) ) ;
#1758=CARTESIAN_POINT ( 'NONE',  ( 3.195700652717397894, 99.49999999999997158, -22.66286045753255962 ) ) ;
#1759=CARTESIAN_POINT ( 'NONE',  ( 19.09188309203678102, 5.299999997815050712, 19.09188309203678813 ) ) ;
#1760=CARTESIAN_POINT ( 'NONE',  ( -20.72805389903318130, 99.50000000000000000, -9.848585782927868237 ) ) ;
#1762=CARTESIAN_POINT ( 'NONE',  ( 3.497829868842083023, 100.0000000000000000, -21.50512556757917793 ) ) ;
#1763=CARTESIAN_POINT ( 'NONE',  ( -22.27115127098604574, 100.0000000000000000, -10.71048520281369676 ) ) ;
#1764=DIRECTION ( 'NONE',  ( -0.000000000000000000, -1.000000000000000000, -0.000000000000000000 ) ) ;
#1769=PLANE ( 'NONE',  #7599 ) ;
#1770=LINE ( 'NONE', #9050, #5729 ) ;
#1771=CARTESIAN_POINT ( 'NONE',  ( -19.09188309203678457, 4.299999999999999822, -19.09188309203678813 ) ) ;
#1773=CARTESIAN_POINT ( 'NONE',  ( -20.69312081029678296, 99.99999999999997158, -9.926742041671966277 ) ) ;
#1775=FACE_OUTER_BOUND ( 'NONE', #6727, .T. ) ;
#1776=CARTESIAN_POINT ( 'NONE',  ( 21.43339342948717885, 100.0000000000000000, -1.392427884615384803 ) ) ;
#1777=VERTEX_POINT ( 'NONE', #5037 ) ;
#1778=ORIENTED_EDGE ( 'NONE', *, *, #7012, .F. ) ;
#1779=CARTESIAN_POINT ( 'NONE',  ( 8.223467485077383898, 99.49999999999997158, 19.78581333328655134 ) ) ;
#1781=DIRECTION ( 'NONE',  ( 0.3918949146621865109, 0.000000000000000000, 0.9200099868272720860 ) ) ;
#1782=CARTESIAN_POINT ( 'NONE',  ( -21.94169572595625795, 99.50000000000000000, -9.715372641902229489 ) ) ;
#1783=CARTESIAN_POINT ( 'NONE',  ( -21.20999280589743918, 100.0000000000000284, -11.35389291771566000 ) ) ;
#1786=CARTESIAN_POINT ( 'NONE',  ( -22.33111803333905243, 99.49999999999997158, -9.558150950182401573 ) ) ;
#1790=VERTEX_POINT ( 'NONE', #9805 ) ;
#1791=ORIENTED_EDGE ( 'NONE', *, *, #2551, .T. ) ;
#1792=EDGE_CURVE ( 'NONE', #5243, #3042, #5518, .T. ) ;
#1793=AXIS2_PLACEMENT_3D ( 'NONE', #8217, #9836, #2575 ) ;
#1794=DIRECTION ( 'NONE',  ( 0.000000000000000000, 1.000000000000000000, 0.000000000000000000 ) ) ;
#1795=CARTESIAN_POINT ( 'NONE',  ( 3.198592217420132666, 99.99999999999997158, -21.96964977087737836 ) ) ;
#1796=CARTESIAN_POINT ( 'NONE',  ( -14.89508182811745662, 99.99999999999997158, 15.38112983991209326 ) ) ;
#1797=CARTESIAN_POINT ( 'NONE',  ( 4.688812652749139609, 100.0000000000000426, -24.54863390154074310 ) ) ;
#1800=DIRECTION ( 'NONE',  ( -0.000000000000000000, 1.000000000000000000, -0.000000000000000000 ) ) ;
#1802=FACE_OUTER_BOUND ( 'NONE', #2622, .T. ) ;
#1803=ORIENTED_EDGE ( 'NONE', *, *, #651, .T. ) ;
#1804=B_SPLINE_CURVE_WITH_KNOTS ( 'NONE', 3,
 ( #8597, #8700, #1420, #1521, #4609, #3158, #7802, #633, #3831, #8649, #6232, #9433, #4715, #7908, #6341, #9535, #4500, #157, #9631 ),
 .UNSPECIFIED., .F., .F.,
 ( 4, 1, 1, 1, 1, 1, 1, 1, 1, 1, 1, 1, 1, 1, 1, 1, 4 ),
 ( 0.000000000000000000, 0.05935611633690887623, 0.1167563879513689451, 0.1743885027374874330, 0.2308223543163396840, 0.2888100779544915953, 0.3475404098195560842, 0.4086537266250744316, 0.4723446836969566465, 0.5362968130936018873, 0.6000923674009760456, 0.6637702377379335328, 0.7274568328636339398, 0.7924602533659969028, 0.8590386936388050287, 0.9283644560612371865, 1.000000000000000000 ),
 .UNSPECIFIED. ) ;
#1805=CYLINDRICAL_SURFACE ( 'NONE', #3738, 27.00000000000000355 ) ;
#1806=CARTESIAN_POINT ( 'NONE',  ( 3.409892249890944527, 99.50000000000000000, -24.50637943905448779 ) ) ;
#1807=CARTESIAN_POINT ( 'NONE',  ( 7.746148141271532950, 99.99999999999997158, 20.51930889200067298 ) ) ;
#1809=CARTESIAN_POINT ( 'NONE',  ( 3.477525819554967423, 99.50000000000000000, -22.44236894434852658 ) ) ;
#1810=CARTESIAN_POINT ( 'NONE',  ( 19.09188309203678813, 3.899999997815050357, -19.09188309203678813 ) ) ;
#1811=CARTESIAN_POINT ( 'NONE',  ( -20.72805389903318130, 100.0000000000000000, -9.848585782927868237 ) ) ;
#1812=CARTESIAN_POINT ( 'NONE',  ( -21.80427673524616239, 100.0000000000000000, -9.663674634844889866 ) ) ;
#1814=CARTESIAN_POINT ( 'NONE',  ( -21.51485068221570174, 99.50000000000000000, -11.09552232883975087 ) ) ;
#1816=CARTESIAN_POINT ( 'NONE',  ( -4.959819536546781389E-15, 4.399999997815050357, 27.00000000000000355 ) ) ;
#1819=CARTESIAN_POINT ( 'NONE',  ( -14.97509118869195888, 99.49999999999998579, 15.26515554624281101 ) ) ;
#1820=DIRECTION ( 'NONE',  ( -0.000000000000000000, 1.000000000000000000, -0.000000000000000000 ) ) ;
#1821=CARTESIAN_POINT ( 'NONE',  ( 19.39806930854667399, 1.749999998907525223, 19.39806930854668465 ) ) ;
#1822=DIRECTION ( 'NONE',  ( 0.5074415416931677969, 0.000000000000000000, 0.8616861851997287269 ) ) ;
#1825=CARTESIAN_POINT ( 'NONE',  ( 0.000000000000000000, 100.0000000000000000, -27.00000000000000355 ) ) ;
#1826=CARTESIAN_POINT ( 'NONE',  ( -21.30928386698190025, 99.99999999999997158, -11.02857376369709996 ) ) ;
#1827=ORIENTED_EDGE ( 'NONE', *, *, #9346, .T. ) ;
#1828=CARTESIAN_POINT ( 'NONE',  ( -22.08823018108446234, 99.99999999999994316, -9.406177930363766038 ) ) ;
#1829=CARTESIAN_POINT ( 'NONE',  ( 3.024867170474271116, 99.99999999999995737, -24.05477125543085748 ) ) ;
#1830=CARTESIAN_POINT ( 'NONE',  ( -16.36254897777739004, 99.50000000000001421, 15.39785597259249350 ) ) ;
#1831=SHAPE_REPRESENTATION_RELATIONSHIP ( 'NONE' , 'NONE' ,  #4065, #1259 ) ;
#1832=CARTESIAN_POINT ( 'NONE',  ( 8.540544597724410991, 100.0000000000000000, 19.98924338346217766 ) ) ;
#1833=CARTESIAN_POINT ( 'NONE',  ( 9.583828860305853681, 99.49999999999998579, 20.68614437522342797 ) ) ;
#1834=PLANE ( 'NONE',  #4779 ) ;
#1835=ORIENTED_EDGE ( 'NONE', *, *, #8450, .F. ) ;
#1839=CARTESIAN_POINT ( 'NONE',  ( 0.000000000000000000, 0.000000000000000000, -27.00000000000000355 ) ) ;
#1840=CARTESIAN_POINT ( 'NONE',  ( 3.399971579580567393, 99.50000000000000000, -21.57509867787664248 ) ) ;
#1841=CARTESIAN_POINT ( 'NONE',  ( 3.689266881520847807, 99.50000000000000000, -22.97735580002706968 ) ) ;
#1843=EDGE_CURVE ( 'NONE', #5137, #7619, #7379, .T. ) ;
#1845=CARTESIAN_POINT ( 'NONE',  ( 8.132491713109025966, 99.50000000000000000, 21.08089001807756091 ) ) ;
#1846=CARTESIAN_POINT ( 'NONE',  ( 3.306546357697854128E-15, 100.0000000000000000, 27.00000000000000355 ) ) ;
#1847=LINE ( 'NONE', #8152, #4801 ) ;
#1849=CYLINDRICAL_SURFACE ( 'NONE', #893, 18.00000000000000000 ) ;
#1850=CARTESIAN_POINT ( 'NONE',  ( -27.43301270000000258, 0.7499999989075251117, -3.359575119402369376E-15 ) ) ;
#1851=CARTESIAN_POINT ( 'NONE',  ( 0.000000000000000000, 97.50000000000000000, -25.00000000000000000 ) ) ;
#1852=VECTOR ( 'NONE', #5066, 1000.000000000000227 ) ;
#1853=CARTESIAN_POINT ( 'NONE',  ( 3.097283534322414766, 99.50000000000002842, -24.18405864774921454 ) ) ;
#1854=CARTESIAN_POINT ( 'NONE',  ( 4.128176300878408256, 99.99999999999998579, -21.47174600747824869 ) ) ;
#1855=ORIENTED_EDGE ( 'NONE', *, *, #9459, .F. ) ;
#1856=CARTESIAN_POINT ( 'NONE',  ( 3.373335371007685435, 99.50000000000000000, -22.75111425220066863 ) ) ;
#1857=CARTESIAN_POINT ( 'NONE',  ( 26.99999999999999645, 5.349999997815049646, 11.18376618407358691 ) ) ;
#1858=CARTESIAN_POINT ( 'NONE',  ( -20.52076770522338833, 99.50000000000000000, -10.69798695537560462 ) ) ;
#1859=CARTESIAN_POINT ( 'NONE',  ( -20.97771390646102319, 99.50000000000002842, -10.03345247102482674 ) ) ;
#1860=CARTESIAN_POINT ( 'NONE',  ( 3.750007936853901658, 100.0000000000000142, -22.95001988029826734 ) ) ;
#1861=VECTOR ( 'NONE', #6954, 1000.000000000000000 ) ;
#1862=CARTESIAN_POINT ( 'NONE',  ( 6.246869686064662197, 100.0000000000000000, 20.92172973853146090 ) ) ;
#1864=FACE_OUTER_BOUND ( 'NONE', #9659, .T. ) ;
#1868=CARTESIAN_POINT ( 'NONE',  ( -14.97579057656165169, 99.50000000000001421, 16.56690896377573452 ) ) ;
#1869=DIRECTION ( 'NONE',  ( -0.000000000000000000, 1.000000000000000000, -0.000000000000000000 ) ) ;
#1871=B_SPLINE_CURVE_WITH_KNOTS ( 'NONE', 3,
 ( #3407, #5076, #4299, #5775, #10092, #6602, #8225 ),
 .UNSPECIFIED., .F., .F.,
 ( 4, 1, 1, 1, 4 ),
 ( 0.000000000000000000, 0.2687002788711734813, 0.5225003893189538173, 0.7676814173175746658, 1.000000000000000000 ),
 .UNSPECIFIED. ) ;
#1872=CARTESIAN_POINT ( 'NONE',  ( 11.36312591709336139, 2.799999998907525267, -27.43301270000000258 ) ) ;
#1874=CARTESIAN_POINT ( 'NONE',  ( 9.342627931057743140, 99.50000000000000000, 21.59831790269294771 ) ) ;
#1875=DIRECTION ( 'NONE',  ( -0.05422338932609765960, 0.000000000000000000, -0.9985288298541962204 ) ) ;
#1876=CARTESIAN_POINT ( 'NONE',  ( 8.223467485077383898, 99.99999999999997158, 19.78581333328655134 ) ) ;
#1878=CARTESIAN_POINT ( 'NONE',  ( -21.49703851962343037, 99.99999999999991473, -9.300281078773625865 ) ) ;
#1879=CARTESIAN_POINT ( 'NONE',  ( 9.500395184910136237, 99.50000000000000000, 21.12540332933289733 ) ) ;
#1883=CARTESIAN_POINT ( 'NONE',  ( 9.431378708427812896, 99.99999999999992895, 21.34379071326255684 ) ) ;
#1884=CARTESIAN_POINT ( 'NONE',  ( -21.13452028402337035, 100.0000000000000000, -9.824917503107416294 ) ) ;
#1886=CARTESIAN_POINT ( 'NONE',  ( -16.34021191015031249, 100.0000000000000000, 16.45483272884350967 ) ) ;
#1889=CARTESIAN_POINT ( 'NONE',  ( -22.31230063665282515, 99.99999999999994316, -10.62159318200525249 ) ) ;
#1890=DIRECTION ( 'NONE',  ( -0.9567206510497618943, 0.000000000000000000, 0.2910078965507976179 ) ) ;
#1892=CARTESIAN_POINT ( 'NONE',  ( 4.154273145530666511, 100.0000000000000000, -22.82723029927519676 ) ) ;
#1893=CARTESIAN_POINT ( 'NONE',  ( -4.959819536546781389E-15, 3.599999997815050534, 27.00000000000000355 ) ) ;
#1894=CARTESIAN_POINT ( 'NONE',  ( -20.66628160326443364, 99.50000000000001421, -10.01789642611028874 ) ) ;
#1896=LINE ( 'NONE', #8343, #2492 ) ;
#1899=CARTESIAN_POINT ( 'NONE',  ( 3.664124300404482337, 99.50000000000002842, -24.27219056640880623 ) ) ;
#1901=ADVANCED_FACE ( 'NONE', ( #6612 ), #3755, .T. ) ;
#1903=CARTESIAN_POINT ( 'NONE',  ( -27.43301270000000258, 3.149999998907524912, -3.359575119402369376E-15 ) ) ;
#1906=CARTESIAN_POINT ( 'NONE',  ( 8.133363296361027395, 99.50000000000004263, 19.85287606700953233 ) ) ;
#1907=EDGE_CURVE ( 'NONE', #1313, #10278, #6130, .T. ) ;
#1908=VERTEX_POINT ( 'NONE', #3803 ) ;
#1909=CARTESIAN_POINT ( 'NONE',  ( 3.563396934924631942, 99.50000000000001421, -22.47881610735839431 ) ) ;
#1910=CARTESIAN_POINT ( 'NONE',  ( 1.653273178848927064E-15, 3.999999997815050889, -27.00000000000000355 ) ) ;
#1914=CARTESIAN_POINT ( 'NONE',  ( -21.99951964646687941, 100.0000000000000142, -11.00094659099690553 ) ) ;
#1917=VECTOR ( 'NONE', #7118, 1000.000000000000000 ) ;
#1921=DIRECTION ( 'NONE',  ( 0.000000000000000000, 1.000000000000000000, 0.000000000000000000 ) ) ;
#1923=CARTESIAN_POINT ( 'NONE',  ( 27.43301270000000258, 4.249999998907525445, 0.000000000000000000 ) ) ;
#1924=CARTESIAN_POINT ( 'NONE',  ( -11.18376618407356737, 0.2500000000000000000, -27.00000000000000355 ) ) ;
#1926=CARTESIAN_POINT ( 'NONE',  ( 4.311343222282856047, 100.0000000000000000, -24.33387958695581688 ) ) ;
#1927=CARTESIAN_POINT ( 'NONE',  ( 7.856939908706818798, 100.0000000000000142, 20.19612520319305560 ) ) ;
#1928=ORIENTED_EDGE ( 'NONE', *, *, #4088, .T. ) ;
#1929=CARTESIAN_POINT ( 'NONE',  ( -21.89277277937676303, 99.49999999999998579, -9.329958722595300458 ) ) ;
#1931=CARTESIAN_POINT ( 'NONE',  ( 3.350143586568126164, 100.0000000000000142, -24.46212657588250394 ) ) ;
#1932=CARTESIAN_POINT ( 'NONE',  ( 9.513000527211589841, 99.50000000000000000, 20.35102222961602436 ) ) ;
#1933=( LENGTH_UNIT ( ) NAMED_UNIT ( * ) SI_UNIT ( .MILLI., .METRE. ) );
#1934=CARTESIAN_POINT ( 'NONE',  ( 0.000000000000000000, 5.000000000000004441, -27.00000000000000355 ) ) ;
#1935=CARTESIAN_POINT ( 'NONE',  ( 9.500395184910136237, 99.50000000000000000, 21.12540332933289733 ) ) ;
#1937=DIRECTION ( 'NONE',  ( -0.000000000000000000, 1.000000000000000000, -0.000000000000000000 ) ) ;
#1938=EDGE_LOOP ( 'NONE', ( #1426, #6837, #5410, #6885 ) ) ;
#1939=CARTESIAN_POINT ( 'NONE',  ( 8.132491713109025966, 99.50000000000000000, 21.08089001807756091 ) ) ;
#1940=AXIS2_PLACEMENT_3D ( 'NONE', #5406, #3725, #2205 ) ;
#1942=ORIENTED_EDGE ( 'NONE', *, *, #6701, .T. ) ;
#1943=CARTESIAN_POINT ( 'NONE',  ( -22.43115009631934953, 99.50000000000001421, -11.08196351649073819 ) ) ;
#1944=DIRECTION ( 'NONE',  ( -0.000000000000000000, 1.000000000000000000, -0.000000000000000000 ) ) ;
#1945=CARTESIAN_POINT ( 'NONE',  ( 3.374624233514611937, 99.50000000000002842, -23.25900349070959550 ) ) ;
#1946=CARTESIAN_POINT ( 'NONE',  ( 4.599186066243659887, 100.0000000000000568, -24.59301055568561623 ) ) ;
#1949=EDGE_CURVE ( 'NONE', #6063, #9655, #8128, .T. ) ;
#1950=CARTESIAN_POINT ( 'NONE',  ( -15.15623813234777018, 99.50000000000000000, 16.19783826294960249 ) ) ;
#1952=DIRECTION ( 'NONE',  ( 6.123233995736763571E-17, 0.000000000000000000, -1.000000000000000000 ) ) ;
#1953=CARTESIAN_POINT ( 'NONE',  ( 9.861577898019769250, 99.99999999999995737, 21.03794551367759169 ) ) ;
#1955=DIRECTION ( 'NONE',  ( -0.2149789550291109352, 0.000000000000000000, -0.9766186814179788067 ) ) ;
#1956=CARTESIAN_POINT ( 'NONE',  ( 27.43301270000000258, 5.199999998907525622, -11.36312591709336139 ) ) ;
#1958=CARTESIAN_POINT ( 'NONE',  ( 3.606694021351891877, 99.50000000000000000, -24.61315535935035115 ) ) ;
#1959=CARTESIAN_POINT ( 'NONE',  ( 7.978247738654171251, 99.99999999999994316, 20.00924965157036794 ) ) ;
#1960=CARTESIAN_POINT ( 'NONE',  ( 9.802580223201115217, 99.49999999999997158, 21.25247094773282086 ) ) ;
#1961=CARTESIAN_POINT ( 'NONE',  ( 1.653273178848927064E-15, 2.399999997815050357, -27.00000000000000355 ) ) ;
#1965=ORIENTED_EDGE ( 'NONE', *, *, #227, .T. ) ;
#1966=CARTESIAN_POINT ( 'NONE',  ( 4.852629679480013891, 99.50000000000001421, -23.84752007312514621 ) ) ;
#1972=FACE_OUTER_BOUND ( 'NONE', #7310, .T. ) ;
#1973=EDGE_CURVE ( 'NONE', #10278, #5989, #2527, .T. ) ;
#1974=CARTESIAN_POINT ( 'NONE',  ( -27.43301270000000258, 1.399999998907525134, -11.36312591709336317 ) ) ;
#1975=CARTESIAN_POINT ( 'NONE',  ( -27.00000000000001421, 0.4500000000000000666, 11.18376618407356560 ) ) ;
#1977=EDGE_CURVE ( 'NONE', #6767, #872, #6929, .T. ) ;
#1979=CARTESIAN_POINT ( 'NONE',  ( 0.000000000000000000, 0.000000000000000000, 0.000000000000000000 ) ) ;
#1981=CARTESIAN_POINT ( 'NONE',  ( 7.783718120363267268, 99.49999999999998579, 21.09473326129887027 ) ) ;
#1985=CARTESIAN_POINT ( 'NONE',  ( 9.389534246205572643, 99.50000000000001421, 21.46805835725047729 ) ) ;
#1986=CARTESIAN_POINT ( 'NONE',  ( -16.56926954694585774, 99.99999999999997158, 15.12296757606276643 ) ) ;
#1987=CARTESIAN_POINT ( 'NONE',  ( 9.547662139763570366, 99.49999999999997158, 20.94662037603165672 ) ) ;
#1988=CARTESIAN_POINT ( 'NONE',  ( 27.00000000000000355, 2.449999999999999734, -11.18376618407356915 ) ) ;
#1990=CARTESIAN_POINT ( 'NONE',  ( -16.35834224700816009, 100.0000000000000000, 16.43761959438736397 ) ) ;
#1992=VERTEX_POINT ( 'NONE', #3850 ) ;
#1993=CARTESIAN_POINT ( 'NONE',  ( 4.739008722453744049, 99.50000000000001421, -24.06821587619827696 ) ) ;
#1996=CARTESIAN_POINT ( 'NONE',  ( -15.22320097062094568, 100.0000000000000142, 16.32303119091969634 ) ) ;
#1999=CARTESIAN_POINT ( 'NONE',  ( -16.84090648038580085, 99.99999999999998579, 15.49469789757679727 ) ) ;
#2000=CARTESIAN_POINT ( 'NONE',  ( 3.535161742238301041, 99.50000000000001421, -24.18247714022527006 ) ) ;
#2001=ORIENTED_EDGE ( 'NONE', *, *, #184, .F. ) ;
#2002=FACE_OUTER_BOUND ( 'NONE', #3692, .T. ) ;
#2003=CARTESIAN_POINT ( 'NONE',  ( 27.43301269999999548, 2.699999998907525178, 11.36312591709337738 ) ) ;
#2005=EDGE_CURVE ( 'NONE', #3644, #8551, #5372, .T. ) ;
#2006=CARTESIAN_POINT ( 'NONE',  ( -16.70213339477928471, 99.99999999999998579, 16.52464093453885852 ) ) ;
#2008=CARTESIAN_POINT ( 'NONE',  ( -21.89277277937676303, 99.99999999999998579, -9.329958722595300458 ) ) ;
#2009=FACE_OUTER_BOUND ( 'NONE', #9388, .T. ) ;
#2010=LINE ( 'NONE', #6781, #10027 ) ;
#2012=CARTESIAN_POINT ( 'NONE',  ( 3.689266881520847807, 100.0000000000000000, -22.97735580002706968 ) ) ;
#2013=VERTEX_POINT ( 'NONE', #3272 ) ;
#2014=B_SPLINE_CURVE_WITH_KNOTS ( 'NONE', 3,
 ( #8567, #1393, #608, #6990, #5435, #8625, #1447 ),
 .UNSPECIFIED., .F., .F.,
 ( 4, 1, 1, 1, 4 ),
 ( 0.000000000000000000, 0.2581490702850675056, 0.5078756004687992043, 0.7540928115589713432, 1.000000000000000000 ),
 .UNSPECIFIED. ) ;
#2015=CARTESIAN_POINT ( 'NONE',  ( -15.98972951825121669, 99.99999999999997158, 15.19400804711857411 ) ) ;
#2017=CARTESIAN_POINT ( 'NONE',  ( 11.36312591709336850, 2.599999998907525534, 27.43301269999999903 ) ) ;
#2019=ORIENTED_EDGE ( 'NONE', *, *, #4043, .T. ) ;
#2026=CARTESIAN_POINT ( 'NONE',  ( -5.039362679103552881E-15, 4.049999998907525267, 27.43301270000000258 ) ) ;
#2029=AXIS2_PLACEMENT_3D ( 'NONE', #10176, #10116, #6975 ) ;
#2030=CARTESIAN_POINT ( 'NONE',  ( -15.29853103387017121, 100.0000000000000142, 14.98378122532347057 ) ) ;
#2031=EDGE_CURVE ( 'NONE', #2682, #8581, #963, .T. ) ;
#2032=DIRECTION ( 'NONE',  ( 0.000000000000000000, 1.430867686834485556E-12, -1.000000000000000000 ) ) ;
#2033=CARTESIAN_POINT ( 'NONE',  ( -16.30857500771091040, 99.99999999999994316, 15.34700649443169063 ) ) ;
#2037=EDGE_CURVE ( 'NONE', #7672, #7769, #9181, .T. ) ;
#2039=CARTESIAN_POINT ( 'NONE',  ( -19.39806930854667755, 1.349999998907525312, -19.39806930854668110 ) ) ;
#2043=CARTESIAN_POINT ( 'NONE',  ( 11.18376618407357093, 4.950000000000000178, -27.00000000000000355 ) ) ;
#2044=DIRECTION ( 'NONE',  ( -0.000000000000000000, 1.000000000000000000, -0.000000000000000000 ) ) ;
#2046=ORIENTED_EDGE ( 'NONE', *, *, #5317, .T. ) ;
#2047=ORIENTED_EDGE ( 'NONE', *, *, #7593, .F. ) ;
#2048=DIRECTION ( 'NONE',  ( -0.000000000000000000, -1.000000000000000000, -0.000000000000000000 ) ) ;
#2049=MECHANICAL_DESIGN_GEOMETRIC_PRESENTATION_REPRESENTATION('',(#2563),#9589);
#2052=CARTESIAN_POINT ( 'NONE',  ( 4.311343222282856047, 99.50000000000000000, -24.33387958695581688 ) ) ;
#2055=CARTESIAN_POINT ( 'NONE',  ( -19.09188309203678813, 5.099999997815051422, 19.09188309203678457 ) ) ;
#2056=CARTESIAN_POINT ( 'NONE',  ( 5.179363668139080445, 99.50000000000007105, -23.94265746362379943 ) ) ;
#2060=CARTESIAN_POINT ( 'NONE',  ( -16.90147242988460263, 99.99999999999998579, 15.68472263728856753 ) ) ;
#2062=ORIENTED_EDGE ( 'NONE', *, *, #3389, .F. ) ;
#2063=CARTESIAN_POINT ( 'NONE',  ( 27.00000000000000355, 1.399999997815050579, 0.000000000000000000 ) ) ;
#2064=CARTESIAN_POINT ( 'NONE',  ( 19.39806930854667399, 5.049999998907525267, 19.39806930854668465 ) ) ;
#2066=CARTESIAN_POINT ( 'NONE',  ( 9.692323321704657602, 99.50000000000001421, 21.58969587442354410 ) ) ;
#2070=CARTESIAN_POINT ( 'NONE',  ( 8.465276868207817884, 99.50000000000001421, 19.66343818277063704 ) ) ;
#2071=CARTESIAN_POINT ( 'NONE',  ( 6.477538756577482459, 100.0000000000000000, 20.49684993083915430 ) ) ;
#2072=CARTESIAN_POINT ( 'NONE',  ( -16.56313167360273297, 99.50000000000002842, 16.06491815633068398 ) ) ;
#2074=EDGE_CURVE ( 'NONE', #1371, #2426, #8723, .T. ) ;
#2076=CARTESIAN_POINT ( 'NONE',  ( -15.56095293356939813, 100.0000000000000142, 15.23332223661997453 ) ) ;
#2077=CARTESIAN_POINT ( 'NONE',  ( 27.43301270000000258, 2.799999998907524823, -11.36312591709336139 ) ) ;
#2078=ORIENTED_EDGE ( 'NONE', *, *, #1453, .T. ) ;
#2084=CARTESIAN_POINT ( 'NONE',  ( 27.43301269999999548, 4.999999998907525445, 11.36312591709337738 ) ) ;
#2085=CARTESIAN_POINT ( 'NONE',  ( 11.36312591709336850, 2.599999998907525534, 27.43301269999999903 ) ) ;
#2087=CARTESIAN_POINT ( 'NONE',  ( -15.70584307919286893, 100.0000000000000000, 14.84247401567675162 ) ) ;
#2088=CARTESIAN_POINT ( 'NONE',  ( 10.72103337977569204, 100.0000000000000000, 22.20268488987243316 ) ) ;
#2089=CARTESIAN_POINT ( 'NONE',  ( 7.734522023158566739, 100.0000000000000284, 20.86022014488863618 ) ) ;
#2091=ADVANCED_FACE ( 'NONE', ( #5581 ), #4840, .T. ) ;
#2092=CARTESIAN_POINT ( 'NONE',  ( 1.653273178848927064E-15, 0.7999999978150503788, -27.00000000000000355 ) ) ;
#2095=CARTESIAN_POINT ( 'NONE',  ( 2.874264611687397331, 100.0000000000000142, -22.24889838548798693 ) ) ;
#2096=ORIENTED_EDGE ( 'NONE', *, *, #294, .T. ) ;
#2097=DIRECTION ( 'NONE',  ( -0.000000000000000000, -1.000000000000000000, -0.000000000000000000 ) ) ;
#2099=CARTESIAN_POINT ( 'NONE',  ( 27.43301269999999548, 2.599999998907525089, 11.36312591709337738 ) ) ;
#2101=DIRECTION ( 'NONE',  ( -0.000000000000000000, 1.000000000000000000, -0.000000000000000000 ) ) ;
#2102=CARTESIAN_POINT ( 'NONE',  ( 1.653273178848927064E-15, 1.000000000000000000, -27.00000000000000355 ) ) ;
#2103=CARTESIAN_POINT ( 'NONE',  ( 8.757234875838378230, 100.0000000000000284, 19.92790116963689329 ) ) ;
#2104=VERTEX_POINT ( 'NONE', #2538 ) ;
#2105=LINE ( 'NONE', #1939, #6229 ) ;
#2107=VERTEX_POINT ( 'NONE', #1739 ) ;
#2108=CARTESIAN_POINT ( 'NONE',  ( 4.584380863705032283, 99.50000000000001421, -24.21384527865288305 ) ) ;
#2109=DIRECTION ( 'NONE',  ( 0.000000000000000000, 1.000000000000000000, 0.000000000000000000 ) ) ;
#2113=CARTESIAN_POINT ( 'NONE',  ( 5.240996349771887886, 100.0000000000000426, -23.60769396873743631 ) ) ;
#2114=B_SPLINE_CURVE_WITH_KNOTS ( 'NONE', 3,
 ( #8736, #6328, #3090, #8047, #673, #1560, #831, #2400, #4751, #779, #881, #3973, #7158, #5595, #3866, #5647, #7254, #9619, #4072 ),
 .UNSPECIFIED., .F., .F.,
 ( 4, 1, 1, 1, 1, 1, 1, 1, 1, 1, 1, 1, 1, 1, 1, 1, 4 ),
 ( 0.000000000000000000, 0.06441145199513656494, 0.1272798026707614161, 0.1891796676955485867, 0.2501048626594916668, 0.3106574229659737063, 0.3727353219478334867, 0.4357106927796215445, 0.5001540812204312569, 0.5646670943021733224, 0.6273118991093056263, 0.6892359343283066542, 0.7500873997029591234, 0.8110709007071082999, 0.8723115105649058565, 0.9354174373376444862, 1.000000000000000000 ),
 .UNSPECIFIED. ) ;
#2115=CIRCLE ( 'NONE', #3631, 7.500000000000000000 ) ;
#2118=CARTESIAN_POINT ( 'NONE',  ( 3.681717055787076642, 99.50000000000000000, -21.09125273517263111 ) ) ;
#2119=CARTESIAN_POINT ( 'NONE',  ( -4.959819536546781389E-15, 1.399999999999999911, 27.00000000000000355 ) ) ;
#2122=CARTESIAN_POINT ( 'NONE',  ( -17.94007301623892658, 99.50000000000000000, 17.49000340848992607 ) ) ;
#2123=CARTESIAN_POINT ( 'NONE',  ( -19.39806930854668465, 4.049999998907525267, 19.39806930854667755 ) ) ;
#2125=CARTESIAN_POINT ( 'NONE',  ( 9.873655262861264603, 99.50000000000000000, 20.34710108723753308 ) ) ;
#2126=CARTESIAN_POINT ( 'NONE',  ( -15.15871127190382417, 99.50000000000000000, 15.63231653451427761 ) ) ;
#2128=CARTESIAN_POINT ( 'NONE',  ( 5.226890989224467710, 99.50000000000000000, -23.72545275563321354 ) ) ;
#2129=CARTESIAN_POINT ( 'NONE',  ( 1.653273178848927064E-15, 3.400000000000000355, -27.00000000000000355 ) ) ;
#2130=FACE_BOUND ( 'NONE', #2901, .T. ) ;
#2133=CARTESIAN_POINT ( 'NONE',  ( 11.36312591709336139, 0.4999999989075251672, -27.43301270000000258 ) ) ;
#2134=ORIENTED_EDGE ( 'NONE', *, *, #2246, .T. ) ;
#2135=VECTOR ( 'NONE', #10163, 1000.000000000000227 ) ;
#2138=CARTESIAN_POINT ( 'NONE',  ( -22.51767453479306980, 99.50000000000000000, -9.764155749770198511 ) ) ;
#2139=CARTESIAN_POINT ( 'NONE',  ( 2.901827748664965068, 99.99999999999995737, -21.68759887446373469 ) ) ;
#2141=CARTESIAN_POINT ( 'NONE',  ( -16.79604063091391097, 99.50000000000000000, 15.40463673182947701 ) ) ;
#2142=CARTESIAN_POINT ( 'NONE',  ( -11.36312591709337383, 1.699999998907525178, 27.43301269999999548 ) ) ;
#2143=ORIENTED_EDGE ( 'NONE', *, *, #2423, .T. ) ;
#2144=ORIENTED_EDGE ( 'NONE', *, *, #3187, .F. ) ;
#2150=LINE ( 'NONE', #7636, #2463 ) ;
#2151=ORIENTED_EDGE ( 'NONE', *, *, #2573, .F. ) ;
#2153=CARTESIAN_POINT ( 'NONE',  ( -21.43094455402013310, 99.50000000000000000, -11.42705968398779426 ) ) ;
#2155=CARTESIAN_POINT ( 'NONE',  ( -19.39806930854667755, 3.749999998907525445, -19.39806930854668110 ) ) ;
#2159=CARTESIAN_POINT ( 'NONE',  ( 27.00000000000000355, 0.8500000000000001998, -11.18376618407356737 ) ) ;
#2160=CARTESIAN_POINT ( 'NONE',  ( 9.446088657802272692, 99.50000000000004263, 20.22669104216016578 ) ) ;
#2162=CARTESIAN_POINT ( 'NONE',  ( 8.540544597724410991, 99.50000000000000000, 19.98924338346217766 ) ) ;
#2163=CARTESIAN_POINT ( 'NONE',  ( 8.102924533678123709, 100.0000000000000000, 20.98904009517733726 ) ) ;
#2166=ORIENTED_EDGE ( 'NONE', *, *, #7977, .F. ) ;
#2168=B_SPLINE_CURVE_WITH_KNOTS ( 'NONE', 3,
 ( #3512, #429, #9214, #7535, #7432, #9845, #2679, #3627, #5869, #325, #2733, #2784, #6807, #10005, #9385 ),
 .UNSPECIFIED., .F., .F.,
 ( 4, 1, 1, 1, 1, 1, 1, 1, 1, 1, 1, 1, 4 ),
 ( 0.000000000000000000, 0.1055296353700490852, 0.2070742529895955586, 0.3056622059958778448, 0.4023599870273183998, 0.4943057198019382148, 0.5778637904027289496, 0.6550095244395398586, 0.7278863574113029200, 0.7976678238154090161, 0.8645871040366396310, 0.9319858836656568224, 1.000000000000000000 ),
 .UNSPECIFIED. ) ;
#2169=CARTESIAN_POINT ( 'NONE',  ( -22.55793349878803156, 99.50000000000000000, -10.88926985104519929 ) ) ;
#2170=CARTESIAN_POINT ( 'NONE',  ( -11.36312591709337561, 0.7999999989075252671, 27.43301269999999548 ) ) ;
#2171=CARTESIAN_POINT ( 'NONE',  ( -21.04016555629948826, 99.50000000000001421, -9.929603401003973318 ) ) ;
#2174=EDGE_CURVE ( 'NONE', #2880, #4986, #4009, .T. ) ;
#2175=CARTESIAN_POINT ( 'NONE',  ( 21.79306891025641235, 99.50000000000000000, -1.065004006410256387 ) ) ;
#2176=CARTESIAN_POINT ( 'NONE',  ( 4.793167276645844410, 99.49999999999998579, -21.69837440717521204 ) ) ;
#2177=CARTESIAN_POINT ( 'NONE',  ( 1.653273178848927064E-15, 1.000000000000000000, -27.00000000000000355 ) ) ;
#2178=CARTESIAN_POINT ( 'NONE',  ( -16.60513711880302878, 100.0000000000000000, 15.15667007515659570 ) ) ;
#2179=EDGE_CURVE ( 'NONE', #1114, #8029, #9517, .T. ) ;
#2180=CARTESIAN_POINT ( 'NONE',  ( 3.058419780146050648, 100.0000000000000000, -23.12871267107006545 ) ) ;
#2185=CARTESIAN_POINT ( 'NONE',  ( -21.39817337045129619, 100.0000000000000142, -9.317726141196148504 ) ) ;
#2187=CARTESIAN_POINT ( 'NONE',  ( 5.207032889226773875, 99.50000000000000000, -23.83708953234284778 ) ) ;
#2191=B_SPLINE_CURVE_WITH_KNOTS ( 'NONE', 3,
 ( #5025, #9165, #5820, #2580, #9891, #4977, #7588, #5128, #8222, #9841, #5773, #8328, #1158, #426, #220, #8964, #7382, #2674, #1830 ),
 .UNSPECIFIED., .F., .F.,
 ( 4, 1, 1, 1, 1, 1, 1, 1, 1, 1, 1, 1, 1, 1, 1, 1, 4 ),
 ( 0.000000000000000000, 0.06485467887857676583, 0.1277145915909605745, 0.1892127134908106190, 0.2497332716026948729, 0.3109554005383074471, 0.3726238983726959941, 0.4350931267523188151, 0.5000867325104639827, 0.5644742510850394579, 0.6276292343746815439, 0.6888483565510189477, 0.7500704854866314664, 0.8105910435985150819, 0.8724026516570742018, 0.9351453211214243444, 1.000000000000000000 ),
 .UNSPECIFIED. ) ;
#2197=CARTESIAN_POINT ( 'NONE',  ( 3.428579745388047328, 99.49999999999998579, -21.16399209792802694 ) ) ;
#2199=CARTESIAN_POINT ( 'NONE',  ( 4.887668416326221177, 99.50000000000001421, -23.70513093767710089 ) ) ;
#2200=CARTESIAN_POINT ( 'NONE',  ( 1.679787559701184688E-15, 2.949999998907525178, -27.43301270000000258 ) ) ;
#2201=CARTESIAN_POINT ( 'NONE',  ( -16.49882833452567965, 100.0000000000000000, 15.05677840364783115 ) ) ;
#2202=AXIS2_PLACEMENT_3D ( 'NONE', #5308, #9280, #1331 ) ;
#2204=CARTESIAN_POINT ( 'NONE',  ( -16.61132721736409934, 99.50000000000001421, 16.61681399495993716 ) ) ;
#2205=DIRECTION ( 'NONE',  ( -0.9851965920526258857, 0.000000000000000000, -0.1714283378204774222 ) ) ;
#2207=CARTESIAN_POINT ( 'NONE',  ( 4.118246196500586542, 99.99999999999998579, -21.10643963665684453 ) ) ;
#2208=ORIENTED_EDGE ( 'NONE', *, *, #6691, .T. ) ;
#2209=DIRECTION ( 'NONE',  ( 0.000000000000000000, 1.000000000000000000, 0.000000000000000000 ) ) ;
#2210=CARTESIAN_POINT ( 'NONE',  ( 19.39806930854667399, 0.9499999989075252893, 19.39806930854668465 ) ) ;
#2211=ORIENTED_EDGE ( 'NONE', *, *, #7162, .F. ) ;
#2213=VECTOR ( 'NONE', #3036, 1000.000000000000000 ) ;
#2214=CARTESIAN_POINT ( 'NONE',  ( 27.00000000000000355, 2.400000000000000355, 0.000000000000000000 ) ) ;
#2215=CARTESIAN_POINT ( 'NONE',  ( 8.612131858919537919, 100.0000000000000142, 19.96100069886393413 ) ) ;
#2216=ORIENTED_EDGE ( 'NONE', *, *, #1609, .T. ) ;
#2217=ORIENTED_EDGE ( 'NONE', *, *, #445, .F. ) ;
#2218=CARTESIAN_POINT ( 'NONE',  ( -15.10687288066601930, 99.49999999999998579, 15.84109048427130517 ) ) ;
#2219=CARTESIAN_POINT ( 'NONE',  ( -15.69015368034045643, 99.50000000000001421, 16.64011368054243434 ) ) ;
#2222=ORIENTED_EDGE ( 'NONE', *, *, #3890, .T. ) ;
#2223=VECTOR ( 'NONE', #3534, 1000.000000000000000 ) ;
#2224=EDGE_CURVE ( 'NONE', #1392, #7177, #1871, .T. ) ;
#2226=CARTESIAN_POINT ( 'NONE',  ( -21.59424432678268957, 99.49999999999997158, -9.639623801236600897 ) ) ;
#2228=CARTESIAN_POINT ( 'NONE',  ( 4.772556553149396308, 100.0000000000000000, -24.49721679606612312 ) ) ;
#2232=ADVANCED_FACE ( 'NONE', ( #9792 ), #1106, .T. ) ;
#2233=CARTESIAN_POINT ( 'NONE',  ( 4.232798786556307036, 99.50000000000000000, -24.34936571594186105 ) ) ;
#2234=ORIENTED_EDGE ( 'NONE', *, *, #368, .F. ) ;
#2238=EDGE_CURVE ( 'NONE', #10097, #3601, #324, .T. ) ;
#2239=VERTEX_POINT ( 'NONE', #1832 ) ;
#2240=DIRECTION ( 'NONE',  ( -0.2892158999609669712, 0.000000000000000000, -0.9572638942369904314 ) ) ;
#2242=EDGE_CURVE ( 'NONE', #7345, #6501, #8011, .T. ) ;
#2245=ORIENTED_EDGE ( 'NONE', *, *, #6517, .F. ) ;
#2246=EDGE_CURVE ( 'NONE', #9118, #369, #2749, .T. ) ;
#2247=CARTESIAN_POINT ( 'NONE',  ( -16.63177974700816009, 99.50000000000000000, 16.59747536361813403 ) ) ;
#2249=ORIENTED_EDGE ( 'NONE', *, *, #2224, .T. ) ;
#2251=EDGE_CURVE ( 'NONE', #8788, #9797, #4200, .T. ) ;
#2254=CARTESIAN_POINT ( 'NONE',  ( 1.679787559701184688E-15, 2.149999998907525356, -27.43301270000000258 ) ) ;
#2255=ORIENTED_EDGE ( 'NONE', *, *, #6056, .F. ) ;
#2256=CARTESIAN_POINT ( 'NONE',  ( -15.10382517959271098, 99.99999999999995737, 15.91526905993627317 ) ) ;
#2257=VECTOR ( 'NONE', #7383, 1000.000000000000000 ) ;
#2258=CARTESIAN_POINT ( 'NONE',  ( 4.054941747578200584, 99.99999999999998579, -24.36678493958047298 ) ) ;
#2260=B_SPLINE_SURFACE_WITH_KNOTS ( 'NONE', 3, 1, ( 
 ( #8845, #8008 ),
 ( #840, #4646 ),
 ( #6434, #6382 ),
 ( #3340, #7116 ),
 ( #4031, #7315 ),
 ( #2355, #7213 ),
 ( #4866, #9575 ),
 ( #9718, #4080 ),
 ( #5552, #6531 ),
 ( #8744, #3247 ),
 ( #1568, #8109 ) ),
 .UNSPECIFIED., .F., .F., .F.,
 ( 4, 1, 1, 1, 1, 1, 1, 1, 4 ),
 ( 2, 2 ),
 ( 0.000000000000000000, 0.09767211715481777246, 0.1989896052561311024, 0.3043518128873296535, 0.4150874769980872347, 0.5363819683935961979, 0.6738601886791220075, 0.8283091006677448798, 1.000000000000000000 ),
 ( 0.000000000000000000, 1.000000000000000000 ),
 .UNSPECIFIED. ) ;
#2261=EDGE_CURVE ( 'NONE', #9021, #519, #7740, .T. ) ;
#2262=CARTESIAN_POINT ( 'NONE',  ( -15.84348323231452049, 100.0000000000000000, 15.18005498687102772 ) ) ;
#2264=CARTESIAN_POINT ( 'NONE',  ( 3.771794781161601939, 99.49999999999998579, -21.07813736596861176 ) ) ;
#2265=ORIENTED_EDGE ( 'NONE', *, *, #2685, .T. ) ;
#2267=CARTESIAN_POINT ( 'NONE',  ( -27.43301270000000969, 2.299999998907525267, 11.36312591709335429 ) ) ;
#2269=CARTESIAN_POINT ( 'NONE',  ( 0.000000000000000000, 100.0000000000000000, -27.00000000000000355 ) ) ;
#2271=CARTESIAN_POINT ( 'NONE',  ( -11.18376618407358336, 0.5500000000000000444, 26.99999999999999645 ) ) ;
#2272=CARTESIAN_POINT ( 'NONE',  ( 9.357295078982289738, 99.50000000000004263, 20.12145687760884627 ) ) ;
#2276=CARTESIAN_POINT ( 'NONE',  ( -16.49092618789450526, 99.50000000000000000, 16.26472549871478179 ) ) ;
#2277=CARTESIAN_POINT ( 'NONE',  ( 8.091962505948220752, 99.99999999999995737, 20.48385654212622242 ) ) ;
#2280=VERTEX_POINT ( 'NONE', #1354 ) ;
#2281=CARTESIAN_POINT ( 'NONE',  ( -27.43301270000000258, 3.799999998907525711, -11.36312591709336317 ) ) ;
#2283=CARTESIAN_POINT ( 'NONE',  ( 5.242860087038358152, 100.0000000000000568, -23.52699316036146371 ) ) ;
#2286=ORIENTED_EDGE ( 'NONE', *, *, #9968, .T. ) ;
#2288=ORIENTED_EDGE ( 'NONE', *, *, #8558, .F. ) ;
#2289=VECTOR ( 'NONE', #4116, 1000.000000000000000 ) ;
#2291=CARTESIAN_POINT ( 'NONE',  ( -16.01161620991261358, 99.50000000000000000, 17.10240122391520146 ) ) ;
#2292=CARTESIAN_POINT ( 'NONE',  ( 9.263267005978743640, 99.49999999999998579, 19.65676951151765905 ) ) ;
#2295=ORIENTED_EDGE ( 'NONE', *, *, #5584, .T. ) ;
#2296=CARTESIAN_POINT ( 'NONE',  ( 2.983739933759421259, 99.49999999999998579, -23.28421226151478152 ) ) ;
#2298=CARTESIAN_POINT ( 'NONE',  ( 9.526349065647009340, 99.50000000000000000, 19.81320455978211470 ) ) ;
#2299=CARTESIAN_POINT ( 'NONE',  ( 0.000000000000000000, 100.0000000000000000, -25.00000000000000000 ) ) ;
#2300=CARTESIAN_POINT ( 'NONE',  ( -16.35834224700816009, 99.50000000000000000, 16.43761959438736397 ) ) ;
#2301=ORIENTED_EDGE ( 'NONE', *, *, #2676, .F. ) ;
#2302=CARTESIAN_POINT ( 'NONE',  ( -27.00000000000000355, 2.599999997815050534, -3.306546357697854128E-15 ) ) ;
#2303=CARTESIAN_POINT ( 'NONE',  ( -11.36312591709337561, 4.899999998907527576, 27.43301269999999548 ) ) ;
#2305=CARTESIAN_POINT ( 'NONE',  ( -20.99557965837879081, 99.99999999999997158, -10.74478602187354959 ) ) ;
#2307=CARTESIAN_POINT ( 'NONE',  ( -16.62994343074595349, 99.49999999999998579, 15.18287566599475191 ) ) ;
#2308=CARTESIAN_POINT ( 'NONE',  ( -27.43301270000000258, 3.899999998907525356, -11.36312591709336317 ) ) ;
#2309=DIRECTION ( 'NONE',  ( 0.000000000000000000, 1.000000000000000000, 0.000000000000000000 ) ) ;
#2310=DIRECTION ( 'NONE',  ( -0.9198211419112228837, 0.000000000000000000, 0.3923379498508065000 ) ) ;
#2311=CARTESIAN_POINT ( 'NONE',  ( 8.132491713109025966, 100.0000000000000000, 21.08089001807756091 ) ) ;
#2312=CARTESIAN_POINT ( 'NONE',  ( -22.58826642033182353, 99.99999999999998579, -9.883148377786627137 ) ) ;
#2314=CARTESIAN_POINT ( 'NONE',  ( 4.570993444255353921, 99.49999999999998579, -21.37574484917381668 ) ) ;
#2315=EDGE_LOOP ( 'NONE', ( #639, #1193, #9766, #6001, #7882, #10359, #3137, #9438, #1307, #1744, #3858, #1327, #6004, #7273, #3797, #5535 ) ) ;
#2317=CARTESIAN_POINT ( 'NONE',  ( 19.39806930854668110, 1.249999998907525223, -19.39806930854668110 ) ) ;
#2318=EDGE_CURVE ( 'NONE', #5272, #1184, #243, .T. ) ;
#2319=CARTESIAN_POINT ( 'NONE',  ( -15.56505537928961047, 99.50000000000002842, 14.87309967080592088 ) ) ;
#2321=CARTESIAN_POINT ( 'NONE',  ( 19.09188309203678102, 0.6999999999999999556, 19.09188309203678813 ) ) ;
#2322=CARTESIAN_POINT ( 'NONE',  ( 8.829292973371666520, 100.0000000000000142, 19.92220432019063736 ) ) ;
#2323=EDGE_LOOP ( 'NONE', ( #7748, #7808, #9311, #9330, #5771, #8232, #4312, #4481 ) ) ;
#2325=CARTESIAN_POINT ( 'NONE',  ( -16.57337958714257908, 99.49999999999998579, 15.99273699073067867 ) ) ;
#2326=CARTESIAN_POINT ( 'NONE',  ( -15.55395551812965671, 99.50000000000002842, 16.59868653893595791 ) ) ;
#2327=VERTEX_POINT ( 'NONE', #9233 ) ;
#2329=ORIENTED_EDGE ( 'NONE', *, *, #9518, .F. ) ;
#2330=CARTESIAN_POINT ( 'NONE',  ( -19.39806930854667755, 1.349999998907525534, -19.39806930854668110 ) ) ;
#2331=CARTESIAN_POINT ( 'NONE',  ( 3.701176614148623756, 100.0000000000000000, -24.64875008328975170 ) ) ;
#2334=PLANE ( 'NONE',  #4109 ) ;
#2338=CARTESIAN_POINT ( 'NONE',  ( 4.118246196500586542, 99.99999999999998579, -21.10643963665684453 ) ) ;
#2339=CARTESIAN_POINT ( 'NONE',  ( 4.739008722453744049, 99.50000000000001421, -24.06821587619827696 ) ) ;
#2342=B_SPLINE_SURFACE_WITH_KNOTS ( 'NONE', 3, 1, ( 
 ( #8056, #9676 ),
 ( #2514, #5705 ),
 ( #1718, #4912 ),
 ( #2560, #5752 ),
 ( #1517, #4710 ),
 ( #7903, #7459 ),
 ( #1909, #9141 ),
 ( #1809, #2653 ),
 ( #6673, #5001 ),
 ( #7358, #8301 ),
 ( #1031, #1132 ),
 ( #1185, #9091 ),
 ( #984, #4325 ),
 ( #4376, #8201 ),
 ( #5101, #199 ) ),
 .UNSPECIFIED., .F., .F., .F.,
 ( 4, 1, 1, 1, 1, 1, 1, 1, 1, 1, 1, 1, 4 ),
 ( 2, 2 ),
 ( 0.000000000000000000, 0.1055296353700490852, 0.2070742529895955586, 0.3056622059958778448, 0.4023599870273183998, 0.4943057198019382148, 0.5778637904027289496, 0.6550095244395398586, 0.7278863574113029200, 0.7976678238154090161, 0.8645871040366396310, 0.9319858836656568224, 1.000000000000000000 ),
 ( 0.000000000000000000, 1.000000000000000000 ),
 .UNSPECIFIED. ) ;
#2343=ORIENTED_EDGE ( 'NONE', *, *, #10127, .T. ) ;
#2344=CARTESIAN_POINT ( 'NONE',  ( -22.28738277804067636, 99.99999999999997158, -10.06255608345902886 ) ) ;
#2346=CARTESIAN_POINT ( 'NONE',  ( -18.01369080470046313, 99.50000000000000000, 17.15556831233607937 ) ) ;
#2347=FACE_OUTER_BOUND ( 'NONE', #5980, .T. ) ;
#2348=CARTESIAN_POINT ( 'NONE',  ( 27.43301269999999548, 3.499999998907525445, 11.36312591709337916 ) ) ;
#2352=VECTOR ( 'NONE', #2815, 1000.000000000000000 ) ;
#2353=CARTESIAN_POINT ( 'NONE',  ( -20.91264567078791714, 99.99999999999997158, -10.54226115003387676 ) ) ;
#2355=CARTESIAN_POINT ( 'NONE',  ( -20.79740905086423552, 99.50000000000001421, -11.06234285579171051 ) ) ;
#2356=CARTESIAN_POINT ( 'NONE',  ( -27.43301270000000258, 4.699999998907525622, -11.36312591709336317 ) ) ;
#2357=CARTESIAN_POINT ( 'NONE',  ( -15.15871127190382417, 99.99999999999997158, 15.63231653451427761 ) ) ;
#2358=CARTESIAN_POINT ( 'NONE',  ( 11.18376618407357626, 3.649999997815050357, 27.00000000000000000 ) ) ;
#2359=CARTESIAN_POINT ( 'NONE',  ( 21.43339342948717885, 99.50000000000000000, -1.392427884615384803 ) ) ;
#2363=CARTESIAN_POINT ( 'NONE',  ( 4.691018317478480526, 99.49999999999995737, -21.52316599815148024 ) ) ;
#2366=CARTESIAN_POINT ( 'NONE',  ( 19.39806930854668110, 0.4499999989075251783, -19.39806930854668110 ) ) ;
#2368=CARTESIAN_POINT ( 'NONE',  ( -11.18376618407358336, 4.549999999999999822, 26.99999999999999645 ) ) ;
#2369=CARTESIAN_POINT ( 'NONE',  ( 3.195700652717397894, 99.99999999999997158, -22.66286045753255962 ) ) ;
#2370=EDGE_CURVE ( 'NONE', #10090, #7760, #5993, .T. ) ;
#2371=ORIENTED_EDGE ( 'NONE', *, *, #5557, .F. ) ;
#2374=CARTESIAN_POINT ( 'NONE',  ( -15.33577160963320374, 99.99999999999998579, 16.45272793336155814 ) ) ;
#2376=ORIENTED_EDGE ( 'NONE', *, *, #3307, .T. ) ;
#2380=CARTESIAN_POINT ( 'NONE',  ( -11.36312591709335962, 1.299999998907525267, -27.43301270000000258 ) ) ;
#2383=CARTESIAN_POINT ( 'NONE',  ( -22.22752541189434794, 99.49999999999994316, -11.26717589342885084 ) ) ;
#2385=CARTESIAN_POINT ( 'NONE',  ( -27.00000000000000355, 1.749999997815050445, -11.18376618407357270 ) ) ;
#2386=EDGE_CURVE ( 'NONE', #2471, #2404, #7063, .T. ) ;
#2387=CARTESIAN_POINT ( 'NONE',  ( -16.81182640597031508, 100.0000000000000000, 16.36129326314865295 ) ) ;
#2388=CARTESIAN_POINT ( 'NONE',  ( 4.363164797760430424, 99.50000000000002842, -21.67376679147534446 ) ) ;
#2389=( BOUNDED_CURVE ( )  B_SPLINE_CURVE ( 2, ( #10046, #5910, #4342, #9944, #2778, #5285, #4447, #9058, #475 ),
 .UNSPECIFIED., .F., .F. ) 
 B_SPLINE_CURVE_WITH_KNOTS ( ( 3, 2, 2, 2, 3 ),
 ( 0.6071428571428570953, 0.6250000000000000000, 0.6428571428571429047, 0.6607142857142856984, 0.6785714285714286031 ),
 .UNSPECIFIED. ) 
 CURVE ( )  GEOMETRIC_REPRESENTATION_ITEM ( )  RATIONAL_B_SPLINE_CURVE ( ( 1.000000000000000000, 0.9238795325112867385, 1.000000000000000000, 0.9238795325112867385, 1.000000000000000000, 0.9238795325112867385, 1.000000000000000000, 0.9238795325112867385, 1.000000000000000000 ) ) 
 REPRESENTATION_ITEM ( '' )  );
#2390=AXIS2_PLACEMENT_3D ( 'NONE', #4355, #2048, #7538 ) ;
#2392=ORIENTED_EDGE ( 'NONE', *, *, #10016, .T. ) ;
#2395=CARTESIAN_POINT ( 'NONE',  ( -15.03963071504896121, 100.0000000000000142, 16.63526396357264758 ) ) ;
#2398=VERTEX_POINT ( 'NONE', #2858 ) ;
#2399=CARTESIAN_POINT ( 'NONE',  ( -22.00707282958688182, 99.99999999999997158, -9.748971510896797810 ) ) ;
#2400=CARTESIAN_POINT ( 'NONE',  ( -22.34945848979098670, 99.50000000000002842, -10.27225542379191481 ) ) ;
#2401=FACE_OUTER_BOUND ( 'NONE', #8600, .T. ) ;
#2402=VECTOR ( 'NONE', #3750, 1000.000000000000114 ) ;
#2403=CARTESIAN_POINT ( 'NONE',  ( -27.43301270000000258, 3.949999998907525178, -3.359575119402369376E-15 ) ) ;
#2404=VERTEX_POINT ( 'NONE', #5098 ) ;
#2407=CARTESIAN_POINT ( 'NONE',  ( -20.91430522584054330, 99.50000000000001421, -10.19152558580213608 ) ) ;
#2408=CARTESIAN_POINT ( 'NONE',  ( -19.09188309203678813, 1.099999997815050312, 19.09188309203678457 ) ) ;
#2410=CARTESIAN_POINT ( 'NONE',  ( -15.22739782325755442, 99.99999999999995737, 15.50750051783781025 ) ) ;
#2412=CARTESIAN_POINT ( 'NONE',  ( -16.18394139941567644, 99.50000000000000000, 16.57042731130403723 ) ) ;
#2413=CARTESIAN_POINT ( 'NONE',  ( 26.99999999999999645, 3.950000000000000178, 11.18376618407358691 ) ) ;
#2415=CARTESIAN_POINT ( 'NONE',  ( 4.202475441399873723, 99.50000000000000000, -24.35385978717689071 ) ) ;
#2418=CARTESIAN_POINT ( 'NONE',  ( -27.43301270000000969, 0.7999999989075252671, 11.36312591709335429 ) ) ;
#2421=CARTESIAN_POINT ( 'NONE',  ( -11.18376618407358336, 2.950000000000000178, 26.99999999999999645 ) ) ;
#2422=FACE_OUTER_BOUND ( 'NONE', #1938, .T. ) ;
#2423=EDGE_CURVE ( 'NONE', #3612, #1790, #9034, .T. ) ;
#2425=CARTESIAN_POINT ( 'NONE',  ( -20.95611194834973645, 99.50000000000000000, -10.07788454426966318 ) ) ;
#2426=VERTEX_POINT ( 'NONE', #4320 ) ;
#2429=CARTESIAN_POINT ( 'NONE',  ( -19.39806930854667755, 2.149999998907525356, -19.39806930854668110 ) ) ;
#2430=CARTESIAN_POINT ( 'NONE',  ( 3.171774962637509798, 99.50000000000000000, -24.28498992023182268 ) ) ;
#2431=PRODUCT_DEFINITION_SHAPE ( 'NONE', 'NONE',  #2680 ) ;
#2432=DIRECTION ( 'NONE',  ( 0.9985288298541962204, 0.000000000000000000, -0.05422338932609765960 ) ) ;
#2434=CARTESIAN_POINT ( 'NONE',  ( -16.57337958714257908, 99.99999999999998579, 15.99273699073067867 ) ) ;
#2435=AXIS2_PLACEMENT_3D ( 'NONE', #6046, #2240, #5383 ) ;
#2436=CARTESIAN_POINT ( 'NONE',  ( -22.67341330918043951, 99.50000000000000000, -10.57563951594260665 ) ) ;
#2437=CARTESIAN_POINT ( 'NONE',  ( 4.850954546176396320, 99.99999999999998579, -24.43907202982397209 ) ) ;
#2442=CARTESIAN_POINT ( 'NONE',  ( 4.693123912524271191, 99.50000000000002842, -24.12247278045041554 ) ) ;
#2443=CARTESIAN_POINT ( 'NONE',  ( -16.01161620991261358, 100.0000000000000000, 17.10240122391520146 ) ) ;
#2444=CARTESIAN_POINT ( 'NONE',  ( 27.21650635000000307, 0.1249999994537626252, 0.000000000000000000 ) ) ;
#2446=B_SPLINE_CURVE_WITH_KNOTS ( 'NONE', 3,
 ( #9767, #3432, #4176, #299, #8354, #5951, #5052, #3488, #9869, #9978, #1960, #6625, #6576, #5156, #2606 ),
 .UNSPECIFIED., .F., .F.,
 ( 4, 1, 1, 1, 1, 1, 1, 1, 1, 1, 1, 1, 4 ),
 ( 0.000000000000000000, 0.09895296010982183865, 0.1966578232739713550, 0.2939931048315790330, 0.3929322324600736938, 0.4463669803336778319, 0.5055752425223922764, 0.5715235163887821823, 0.6440401046887170855, 0.7229629404452876384, 0.8087840669208056221, 0.9009145765370688563, 1.000000000000000000 ),
 .UNSPECIFIED. ) ;
#2447=ORIENTED_EDGE ( 'NONE', *, *, #322, .F. ) ;
#2448=EDGE_CURVE ( 'NONE', #969, #8911, #5891, .T. ) ;
#2449=CARTESIAN_POINT ( 'NONE',  ( -21.94169572595625795, 100.0000000000000000, -9.715372641902229489 ) ) ;
#2450=ORIENTED_EDGE ( 'NONE', *, *, #9527, .F. ) ;
#2452=CARTESIAN_POINT ( 'NONE',  ( -15.03963071504896121, 99.50000000000001421, 16.63526396357264758 ) ) ;
#2453=CARTESIAN_POINT ( 'NONE',  ( 9.357295078982289738, 100.0000000000000426, 20.12145687760884627 ) ) ;
#2455=CARTESIAN_POINT ( 'NONE',  ( 3.302864939465488536, 100.0000000000000142, -22.83905924565489443 ) ) ;
#2459=CARTESIAN_POINT ( 'NONE',  ( -21.03403678956047074, 99.50000000000001421, -10.80451401317004922 ) ) ;
#2460=CARTESIAN_POINT ( 'NONE',  ( -5.039362679103552881E-15, 4.149999998907524912, 27.43301270000000258 ) ) ;
#2462=CARTESIAN_POINT ( 'NONE',  ( -15.13520964245927836, 99.49999999999998579, 15.69931698147095034 ) ) ;
#2463=VECTOR ( 'NONE', #7583, 1000.000000000000000 ) ;
#2469=CARTESIAN_POINT ( 'NONE',  ( 9.881472129446523311, 100.0000000000000284, 20.94326683228310060 ) ) ;
#2470=ORIENTED_EDGE ( 'NONE', *, *, #3419, .T. ) ;
#2471=VERTEX_POINT ( 'NONE', #1851 ) ;
#2473=CARTESIAN_POINT ( 'NONE',  ( -11.36312591709335962, 1.399999998907525578, -27.43301270000000258 ) ) ;
#2475=CARTESIAN_POINT ( 'NONE',  ( 1.679787559701184688E-15, 0.4499999989075252338, -27.43301270000000258 ) ) ;
#2476=CARTESIAN_POINT ( 'NONE',  ( -21.07003209069497984, 99.99999999999998579, -11.28505157174820361 ) ) ;
#2479=CARTESIAN_POINT ( 'NONE',  ( -21.18296228862668329, 99.50000000000002842, -10.95406920104765724 ) ) ;
#2480=ORIENTED_EDGE ( 'NONE', *, *, #6506, .F. ) ;
#2481=ORIENTED_EDGE ( 'NONE', *, *, #6348, .T. ) ;
#2482=CARTESIAN_POINT ( 'NONE',  ( 2.847408871211157155, 100.0000000000000142, -22.10537533382872510 ) ) ;
#2484=CARTESIAN_POINT ( 'NONE',  ( -27.43301270000000258, 2.199999998907525622, -11.36312591709336317 ) ) ;
#2486=EDGE_CURVE ( 'NONE', #9410, #3042, #5047, .T. ) ;
#2487=CARTESIAN_POINT ( 'NONE',  ( -22.10910773081910818, 100.0000000000000142, -11.33820747227609793 ) ) ;
#2489=CARTESIAN_POINT ( 'NONE',  ( -16.49092618789450526, 100.0000000000000000, 16.26472549871478179 ) ) ;
#2490=CARTESIAN_POINT ( 'NONE',  ( -16.84090648038580085, 99.49999999999998579, 15.49469789757679727 ) ) ;
#2491=CARTESIAN_POINT ( 'NONE',  ( 4.922541232168287983, 100.0000000000000284, -24.37252920941159928 ) ) ;
#2492=VECTOR ( 'NONE', #6820, 1000.000000000000000 ) ;
#2495=CARTESIAN_POINT ( 'NONE',  ( 4.457146071884139360, 99.50000000000001421, -24.28472590373185724 ) ) ;
#2496=EDGE_CURVE ( 'NONE', #6993, #5685, #2105, .T. ) ;
#2499=ORIENTED_EDGE ( 'NONE', *, *, #4168, .T. ) ;
#2500=EDGE_CURVE ( 'NONE', #1790, #3644, #328, .T. ) ;
#2504=ADVANCED_FACE ( 'NONE', ( #3737 ), #5978, .T. ) ;
#2505=CARTESIAN_POINT ( 'NONE',  ( -16.30857500771091040, 99.49999999999994316, 15.34700649443169063 ) ) ;
#2507=CARTESIAN_POINT ( 'NONE',  ( -5.039362679103552881E-15, 4.949999998907525622, 27.43301270000000258 ) ) ;
#2509=ADVANCED_FACE ( 'NONE', ( #1164 ), #1270, .T. ) ;
#2510=CARTESIAN_POINT ( 'NONE',  ( -20.42657152723830905, 99.50000000000000000, -10.54129411626120216 ) ) ;
#2511=CARTESIAN_POINT ( 'NONE',  ( -20.89884294283097432, 100.0000000000000142, -10.47119744953613640 ) ) ;
#2514=CARTESIAN_POINT ( 'NONE',  ( 4.061806280070601183, 99.50000000000001421, -22.51960061163626392 ) ) ;
#2515=CARTESIAN_POINT ( 'NONE',  ( 19.09188309203678813, 0.6999999978150504010, -19.09188309203678813 ) ) ;
#2517=ORIENTED_EDGE ( 'NONE', *, *, #4438, .F. ) ;
#2518=CARTESIAN_POINT ( 'NONE',  ( 3.386276725104728769, 100.0000000000000142, -24.01678749451497907 ) ) ;
#2520=B_SPLINE_SURFACE_WITH_KNOTS ( 'NONE', 3, 1, ( 
 ( #4886, #8864 ),
 ( #1690, #6357 ),
 ( #910, #3314 ),
 ( #370, #1002 ),
 ( #218, #4295 ),
 ( #1101, #5818 ),
 ( #4399, #7479 ),
 ( #7584, #9161 ),
 ( #6646, #2623 ),
 ( #268, #8174 ),
 ( #5176, #2779 ),
 ( #3403, #1878 ),
 ( #4975, #7380 ),
 ( #4195, #3458 ),
 ( #9839, #6597 ),
 ( #1929, #5864 ),
 ( #8220, #9888 ),
 ( #9787, #2672 ),
 ( #9008, #1828 ) ),
 .UNSPECIFIED., .F., .F., .F.,
 ( 4, 1, 1, 1, 1, 1, 1, 1, 1, 1, 1, 1, 1, 1, 1, 1, 4 ),
 ( 2, 2 ),
 ( 0.000000000000000000, 0.06358429906668214282, 0.1250797439647324816, 0.1854075229911844314, 0.2454523280917267347, 0.3052969617611028252, 0.3655926515411210831, 0.4275661794825392770, 0.4916205250740160460, 0.5555554127340263104, 0.6185525978810689773, 0.6803322039413655098, 0.7423868736098769849, 0.8044290668430417179, 0.8676072479036442964, 0.9329923078238739897, 1.000000000000000000 ),
 ( 0.000000000000000000, 1.000000000000000000 ),
 .UNSPECIFIED. ) ;
#2526=CARTESIAN_POINT ( 'NONE',  ( -16.12311789350856017, 99.50000000000000000, 14.86696503675854686 ) ) ;
#2527=B_SPLINE_CURVE_WITH_KNOTS ( 'NONE', 3,
 ( #4636, #6873, #605, #3745, #7660, #7829, #3902, #10014, #10188, #9223, #9282 ),
 .UNSPECIFIED., .F., .F.,
 ( 4, 1, 1, 1, 1, 1, 1, 1, 4 ),
 ( 0.000000000000000000, 0.1307887167449866828, 0.2576322083635017579, 0.3824781763252146916, 0.5056045358258490774, 0.6278910088851102911, 0.7502354365656509483, 0.8735741898580190457, 1.000000000000000000 ),
 .UNSPECIFIED. ) ;
#2528=CARTESIAN_POINT ( 'NONE',  ( -19.09188309203678457, 3.500000000000000000, -19.09188309203678813 ) ) ;
#2529=CARTESIAN_POINT ( 'NONE',  ( 2.912748042341355870, 99.49999999999998579, -22.34826719014139940 ) ) ;
#2530=CARTESIAN_POINT ( 'NONE',  ( 24.93339342948717885, 99.50000000000000000, -1.235376602564102644 ) ) ;
#2531=CARTESIAN_POINT ( 'NONE',  ( -20.93486371557392545, 99.49999999999998579, -10.61231311368802466 ) ) ;
#2532=VERTEX_POINT ( 'NONE', #2843 ) ;
#2533=ORIENTED_EDGE ( 'NONE', *, *, #2005, .F. ) ;
#2534=CARTESIAN_POINT ( 'NONE',  ( 11.36312591709336139, 4.399999998907524912, -27.43301270000000258 ) ) ;
#2535=CARTESIAN_POINT ( 'NONE',  ( 2.971063225226878046, 100.0000000000000000, -23.91837856253154015 ) ) ;
#2536=CARTESIAN_POINT ( 'NONE',  ( -21.71039561923405969, 100.0000000000000426, -11.44438725057713313 ) ) ;
#2538=CARTESIAN_POINT ( 'NONE',  ( -15.07178375341841381, 100.0000000000000000, 16.66969090848992607 ) ) ;
#2539=CARTESIAN_POINT ( 'NONE',  ( 27.00000000000000355, 1.600000000000000089, 0.000000000000000000 ) ) ;
#2540=CARTESIAN_POINT ( 'NONE',  ( 19.09188309203678102, 5.299999997815050712, 19.09188309203678813 ) ) ;
#2543=ORIENTED_EDGE ( 'NONE', *, *, #5103, .F. ) ;
#2544=LINE ( 'NONE', #8925, #5645 ) ;
#2546=CARTESIAN_POINT ( 'NONE',  ( 9.357053078540884528, 99.50000000000001421, 19.70216357796830664 ) ) ;
#2548=CIRCLE ( 'NONE', #9882, 18.00000000000000000 ) ;
#2550=ORIENTED_EDGE ( 'NONE', *, *, #4727, .F. ) ;
#2551=EDGE_CURVE ( 'NONE', #2327, #7711, #6866, .T. ) ;
#2552=CARTESIAN_POINT ( 'NONE',  ( 8.467217662126737210, 99.50000000000001421, 20.02246181083229004 ) ) ;
#2555=CARTESIAN_POINT ( 'NONE',  ( 8.540544597724410991, 100.0000000000000000, 19.98924338346217766 ) ) ;
#2557=CARTESIAN_POINT ( 'NONE',  ( 3.411785164761435674, 100.0000000000000000, -22.76693382491622231 ) ) ;
#2559=CARTESIAN_POINT ( 'NONE',  ( 7.726884419709978857, 99.50000000000000000, 20.74516479202295471 ) ) ;
#2560=CARTESIAN_POINT ( 'NONE',  ( 3.873456569393397331, 99.50000000000002842, -22.53291374702356364 ) ) ;
#2561=CARTESIAN_POINT ( 'NONE',  ( 26.99999999999999645, 1.349999997815050312, 11.18376618407358691 ) ) ;
#2563=STYLED_ITEM ( 'NONE', ( #2628 ), #1259 ) ;
#2564=CARTESIAN_POINT ( 'NONE',  ( -21.59424432678268957, 99.99999999999997158, -9.639623801236600897 ) ) ;
#2566=FACE_OUTER_BOUND ( 'NONE', #6252, .T. ) ;
#2567=VERTEX_POINT ( 'NONE', #2684 ) ;
#2569=CARTESIAN_POINT ( 'NONE',  ( -14.79004890936967875, 99.99999999999997158, 16.19006955939758541 ) ) ;
#2570=CARTESIAN_POINT ( 'NONE',  ( 2.983739933759421259, 99.99999999999998579, -23.28421226151478152 ) ) ;
#2571=CARTESIAN_POINT ( 'NONE',  ( 11.18376618407357626, 4.650000000000001243, 27.00000000000000000 ) ) ;
#2572=CARTESIAN_POINT ( 'NONE',  ( 3.195700652717397894, 99.49999999999997158, -22.66286045753255962 ) ) ;
#2573=EDGE_CURVE ( 'NONE', #6063, #5137, #3517, .T. ) ;
#2575=DIRECTION ( 'NONE',  ( 0.000000000000000000, 0.000000000000000000, -1.000000000000000000 ) ) ;
#2576=CARTESIAN_POINT ( 'NONE',  ( -20.93575003794465061, 99.99999999999998579, -10.12220034237898503 ) ) ;
#2577=ORIENTED_EDGE ( 'NONE', *, *, #9187, .T. ) ;
#2578=CARTESIAN_POINT ( 'NONE',  ( 8.132491713109025966, 99.50000000000000000, 21.08089001807756091 ) ) ;
#2580=CARTESIAN_POINT ( 'NONE',  ( -15.43596444985078975, 99.50000000000002842, 15.30036492734783593 ) ) ;
#2582=CARTESIAN_POINT ( 'NONE',  ( -22.57971655928959365, 99.50000000000000000, -10.84768434062017839 ) ) ;
#2584=CARTESIAN_POINT ( 'NONE',  ( -22.63784607493503387, 100.0000000000000142, -10.71517552924587058 ) ) ;
#2585=CARTESIAN_POINT ( 'NONE',  ( 8.337740814200648387, 100.0000000000000284, 20.10843643765939248 ) ) ;
#2588=VERTEX_POINT ( 'NONE', #5189 ) ;
#2590=CARTESIAN_POINT ( 'NONE',  ( 3.207057600658871355, 99.99999999999997158, -22.07913334414698880 ) ) ;
#2591=VECTOR ( 'NONE', #5417, 1000.000000000000000 ) ;
#2592=ADVANCED_FACE ( 'NONE', ( #5240 ), #10200, .T. ) ;
#2593=LINE ( 'NONE', #5782, #9716 ) ;
#2594=CARTESIAN_POINT ( 'NONE',  ( 4.503533123526070270, 99.99999999999998579, -24.63026223303895890 ) ) ;
#2597=DIRECTION ( 'NONE',  ( 0.000000000000000000, 0.000000000000000000, 1.000000000000000000 ) ) ;
#2599=CARTESIAN_POINT ( 'NONE',  ( 1.679787559701184688E-15, 5.324999998907524734, -27.43301270000000258 ) ) ;
#2600=VERTEX_POINT ( 'NONE', #701 ) ;
#2602=ADVANCED_FACE ( 'NONE', ( #9334 ), #7858, .T. ) ;
#2604=CARTESIAN_POINT ( 'NONE',  ( 8.429066232339796017, 99.99999999999994316, 19.67794530653910101 ) ) ;
#2605=ORIENTED_EDGE ( 'NONE', *, *, #5916, .T. ) ;
#2606=CARTESIAN_POINT ( 'NONE',  ( 9.676361905416721143, 99.50000000000001421, 21.63547735782115566 ) ) ;
#2607=CARTESIAN_POINT ( 'NONE',  ( 11.18376618407357626, 2.849999997815050978, 27.00000000000000000 ) ) ;
#2609=CARTESIAN_POINT ( 'NONE',  ( -21.87421819196487505, 99.50000000000000000, -9.684578881761979119 ) ) ;
#2610=CARTESIAN_POINT ( 'NONE',  ( -20.96643530928959365, 99.50000000000000000, -10.05541671241504886 ) ) ;
#2611=CARTESIAN_POINT ( 'NONE',  ( -22.05902956123343017, 100.0000000000000000, -10.96257574645357558 ) ) ;
#2615=CARTESIAN_POINT ( 'NONE',  ( 2.958578797724396026, 100.0000000000000000, -23.36432507653281121 ) ) ;
#2616=CARTESIAN_POINT ( 'NONE',  ( 11.36312591709336139, 1.199999998907525178, -27.43301270000000258 ) ) ;
#2618=CARTESIAN_POINT ( 'NONE',  ( -20.72805389903318130, 100.0000000000000000, -9.848585782927868237 ) ) ;
#2619=AXIS2_PLACEMENT_3D ( 'NONE', #9645, #8259, #7412 ) ;
#2621=CARTESIAN_POINT ( 'NONE',  ( -20.89169796687544789, 99.99999999999998579, -10.40078880447404330 ) ) ;
#2622=EDGE_LOOP ( 'NONE', ( #10141, #5373, #5393, #1166 ) ) ;
#2623=CARTESIAN_POINT ( 'NONE',  ( -21.20585021321354802, 99.99999999999998579, -9.381045134209834657 ) ) ;
#2625=CARTESIAN_POINT ( 'NONE',  ( 3.293272160652527258, 99.99999999999997158, -24.41359064397622802 ) ) ;
#2626=CARTESIAN_POINT ( 'NONE',  ( 9.575551604960836016, 99.50000000000001421, 20.57049984249936969 ) ) ;
#2627=ADVANCED_FACE ( 'NONE', ( #3844 ), #1504, .T. ) ;
#2628=PRESENTATION_STYLE_ASSIGNMENT (( #7532 ) ) ;
#2632=CARTESIAN_POINT ( 'NONE',  ( -22.21668755910108928, 99.50000000000004263, -9.472979539922778969 ) ) ;
#2633=CARTESIAN_POINT ( 'NONE',  ( 0.000000000000000000, 100.0000000000000000, 0.000000000000000000 ) ) ;
#2635=ORIENTED_EDGE ( 'NONE', *, *, #4929, .F. ) ;
#2636=ORIENTED_EDGE ( 'NONE', *, *, #2261, .F. ) ;
#2637=AXIS2_PLACEMENT_3D ( 'NONE', #9316, #4499, #2032 ) ;
#2638=CARTESIAN_POINT ( 'NONE',  ( -21.20999280589743918, 100.0000000000000284, -11.35389291771566000 ) ) ;
#2639=CARTESIAN_POINT ( 'NONE',  ( 3.317038232150706367, 99.99999999999995737, -21.66195598387956878 ) ) ;
#2641=CARTESIAN_POINT ( 'NONE',  ( -15.11748654497029953, 99.99999999999998579, 15.76872032455190897 ) ) ;
#2643=CARTESIAN_POINT ( 'NONE',  ( 8.149445629999579666, 99.50000000000002842, 20.33980848884064230 ) ) ;
#2644=( BOUNDED_CURVE ( )  B_SPLINE_CURVE ( 2, ( #388, #1171, #4570, #9912, #3843, #10231, #596, #6768, #8342 ),
 .UNSPECIFIED., .F., .F. ) 
 B_SPLINE_CURVE_WITH_KNOTS ( ( 3, 2, 2, 2, 3 ),
 ( 0.4642857142857143016, 0.4821428571428571508, 0.5000000000000000000, 0.5178571428571429047, 0.5357142857142856984 ),
 .UNSPECIFIED. ) 
 CURVE ( )  GEOMETRIC_REPRESENTATION_ITEM ( )  RATIONAL_B_SPLINE_CURVE ( ( 1.000000000000000000, 0.9238795325112867385, 1.000000000000000000, 0.9238795325112867385, 1.000000000000000000, 0.9238795325112867385, 1.000000000000000000, 0.9238795325112867385, 1.000000000000000000 ) ) 
 REPRESENTATION_ITEM ( '' )  );
#2645=CARTESIAN_POINT ( 'NONE',  ( 9.248677610544923766, 100.0000000000000000, 22.83089001807756446 ) ) ;
#2646=CARTESIAN_POINT ( 'NONE',  ( -21.37606745505193473, 100.0000000000000284, -11.05925878703054011 ) ) ;
#2647=VERTEX_POINT ( 'NONE', #7376 ) ;
#2648=CARTESIAN_POINT ( 'NONE',  ( 3.058419780146050648, 100.0000000000000000, -23.12871267107006545 ) ) ;
#2649=CARTESIAN_POINT ( 'NONE',  ( -5.039362679103552881E-15, 4.849999998907525089, 27.43301270000000258 ) ) ;
#2651=CARTESIAN_POINT ( 'NONE',  ( -20.42657152723830905, 99.99999999999997158, -10.54129411626120216 ) ) ;
#2652=CARTESIAN_POINT ( 'NONE',  ( 7.746148141271532950, 99.50000000000002842, 20.51930889200067298 ) ) ;
#2653=CARTESIAN_POINT ( 'NONE',  ( 3.477525819554967423, 100.0000000000000284, -22.44236894434852658 ) ) ;
#2654=CARTESIAN_POINT ( 'NONE',  ( 19.09188309203678813, 4.699999997815051067, -19.09188309203678813 ) ) ;
#2655=CARTESIAN_POINT ( 'NONE',  ( -20.42657152723830905, 99.50000000000000000, -10.54129411626120216 ) ) ;
#2656=CARTESIAN_POINT ( 'NONE',  ( -21.80427673524616239, 99.50000000000000000, -9.663674634844889866 ) ) ;
#2657=CARTESIAN_POINT ( 'NONE',  ( 3.891852272358404807, 100.0000000000000142, -22.89765557720719968 ) ) ;
#2658=EDGE_CURVE ( 'NONE', #7769, #8491, #7787, .T. ) ;
#2659=PLANE ( 'NONE',  #7265 ) ;
#2660=CARTESIAN_POINT ( 'NONE',  ( 4.750280232731688201, 99.50000000000002842, -24.05275076595185624 ) ) ;
#2663=CARTESIAN_POINT ( 'NONE',  ( -14.97579057656165169, 100.0000000000000000, 16.56690896377573452 ) ) ;
#2664=CARTESIAN_POINT ( 'NONE',  ( 2.927917759182871560, 99.99999999999997158, -23.69257214368879261 ) ) ;
#2665=CARTESIAN_POINT ( 'NONE',  ( 11.36312591709336850, 2.499999998907525445, 27.43301269999999903 ) ) ;
#2672=CARTESIAN_POINT ( 'NONE',  ( -22.05573893622344173, 99.99999999999994316, -9.391591294897233766 ) ) ;
#2673=CARTESIAN_POINT ( 'NONE',  ( -11.36312591709335962, 4.499999998907525445, -27.43301270000000258 ) ) ;
#2674=CARTESIAN_POINT ( 'NONE',  ( -16.34436021381890924, 99.50000000000000000, 15.38072013554846151 ) ) ;
#2675=( NAMED_UNIT ( * ) PLANE_ANGLE_UNIT ( ) SI_UNIT ( $, .RADIAN. ) );
#2676=EDGE_CURVE ( 'NONE', #4679, #7989, #7284, .T. ) ;
#2678=CARTESIAN_POINT ( 'NONE',  ( 8.564701892180647036, 99.50000000000000000, 19.97971282122689018 ) ) ;
#2679=CARTESIAN_POINT ( 'NONE',  ( 3.563396934924631942, 99.50000000000001421, -22.47881610735839431 ) ) ;
#2680=PRODUCT_DEFINITION ( 'UNKNOWN', '', #631, #5281 ) ;
#2681=CARTESIAN_POINT ( 'NONE',  ( -21.08523985030068459, 100.0000000000000000, -9.874866134143449159 ) ) ;
#2682=VERTEX_POINT ( 'NONE', #4099 ) ;
#2683=EDGE_CURVE ( 'NONE', #6501, #2239, #3400, .T. ) ;
#2684=CARTESIAN_POINT ( 'NONE',  ( 7.156925775808251622, 99.50000000000000000, 23.91622092442889524 ) ) ;
#2685=EDGE_CURVE ( 'NONE', #6993, #2880, #7232, .T. ) ;
#2687=EDGE_LOOP ( 'NONE', ( #6131, #6118, #754, #8186 ) ) ;
#2688=DIRECTION ( 'NONE',  ( 0.000000000000000000, 0.000000000000000000, 1.000000000000000000 ) ) ;
#2689=CARTESIAN_POINT ( 'NONE',  ( 3.283294465904739390, 100.0000000000000000, -21.71066637097430885 ) ) ;
#2690=ADVANCED_FACE ( 'NONE', ( #124 ), #3263, .T. ) ;
#2691=CARTESIAN_POINT ( 'NONE',  ( 9.184850993605147944E-16, 87.00000000000001421, 7.500000000000000000 ) ) ;
#2694=CARTESIAN_POINT ( 'NONE',  ( 8.281567445270807681, 99.50000000000000000, 20.15885744430370252 ) ) ;
#2696=DIRECTION ( 'NONE',  ( -0.000000000000000000, 1.000000000000000000, -0.000000000000000000 ) ) ;
#2697=CARTESIAN_POINT ( 'NONE',  ( -21.30928386698190025, 100.0000000000000000, -11.02857376369709996 ) ) ;
#2698=DIRECTION ( 'NONE',  ( 0.000000000000000000, 1.000000000000000000, 0.000000000000000000 ) ) ;
#2700=CARTESIAN_POINT ( 'NONE',  ( -4.959819536546781389E-15, 1.199999997815050401, 27.00000000000000355 ) ) ;
#2701=CARTESIAN_POINT ( 'NONE',  ( -19.39806930854668465, 3.249999998907525001, 19.39806930854667755 ) ) ;
#2703=CARTESIAN_POINT ( 'NONE',  ( 4.061354557346970040, 99.99999999999994316, -22.84864678426182039 ) ) ;
#2704=CARTESIAN_POINT ( 'NONE',  ( 3.949943451936506644, 99.99999999999997158, -21.41482314084395711 ) ) ;
#2705=CARTESIAN_POINT ( 'NONE',  ( -20.74358258379034936, 99.99999999999998579, -9.818556592845180120 ) ) ;
#2706=CARTESIAN_POINT ( 'NONE',  ( 27.00000000000000355, 5.399999997815051245, 0.000000000000000000 ) ) ;
#2709=CARTESIAN_POINT ( 'NONE',  ( -21.08523985030068459, 99.50000000000000000, -9.874866134143449159 ) ) ;
#2711=CARTESIAN_POINT ( 'NONE',  ( -21.33175168474226879, 99.50000000000001421, -11.03889704119913162 ) ) ;
#2712=FACE_OUTER_BOUND ( 'NONE', #6941, .T. ) ;
#2714=ORIENTED_EDGE ( 'NONE', *, *, #8288, .T. ) ;
#2718=CARTESIAN_POINT ( 'NONE',  ( -19.39806930854668465, 1.549999998907525489, 19.39806930854667755 ) ) ;
#2724=EDGE_LOOP ( 'NONE', ( #9775, #2480, #2577, #9898 ) ) ;
#2725=FACE_OUTER_BOUND ( 'NONE', #1660, .T. ) ;
#2726=CARTESIAN_POINT ( 'NONE',  ( -21.98271324694694329, 99.50000000000000000, -11.39207625356720222 ) ) ;
#2727=CARTESIAN_POINT ( 'NONE',  ( 10.72103337977569204, 100.0000000000000000, 22.20268488987243316 ) ) ;
#2729=CARTESIAN_POINT ( 'NONE',  ( 9.342627931057743140, 99.50000000000000000, 21.59831790269294771 ) ) ;
#2730=CARTESIAN_POINT ( 'NONE',  ( 4.277141017070624329, 100.0000000000000284, -21.57940364907851816 ) ) ;
#2731=CARTESIAN_POINT ( 'NONE',  ( 9.446088657802272692, 99.50000000000004263, 20.22669104216016578 ) ) ;
#2733=CARTESIAN_POINT ( 'NONE',  ( 3.291601991079349698, 99.49999999999997158, -22.28586332678438353 ) ) ;
#2734=DIRECTION ( 'NONE',  ( -0.000000000000000000, -1.000000000000000000, -0.000000000000000000 ) ) ;
#2736=CARTESIAN_POINT ( 'NONE',  ( -16.11976138926855739, 99.99999999999997158, 16.60078749809536447 ) ) ;
#2738=ORIENTED_EDGE ( 'NONE', *, *, #1843, .F. ) ;
#2739=CARTESIAN_POINT ( 'NONE',  ( -16.36254897777739004, 99.50000000000001421, 15.39785597259249350 ) ) ;
#2741=CARTESIAN_POINT ( 'NONE',  ( -22.28244091826395135, 99.50000000000000000, -10.68852969318427881 ) ) ;
#2742=CARTESIAN_POINT ( 'NONE',  ( -15.30604604128650692, 100.0000000000000000, 15.41317891555018349 ) ) ;
#2743=ORIENTED_EDGE ( 'NONE', *, *, #4990, .F. ) ;
#2744=CARTESIAN_POINT ( 'NONE',  ( -16.52157078939288937, 99.49999999999998579, 16.20087177393598665 ) ) ;
#2746=DIRECTION ( 'NONE',  ( 1.000000000000000000, 0.000000000000000000, 6.123233995736763571E-17 ) ) ;
#2747=LINE ( 'NONE', #3481, #5479 ) ;
#2748=VERTEX_POINT ( 'NONE', #7582 ) ;
#2749=B_SPLINE_CURVE_WITH_KNOTS ( 'NONE', 3,
 ( #523, #9844, #8179, #7684, #9306, #2138, #1007, #5339, #8529, #4981, #9746, #4157, #3362, #6555, #2582 ),
 .UNSPECIFIED., .F., .F.,
 ( 4, 1, 1, 1, 1, 1, 1, 1, 1, 1, 1, 1, 4 ),
 ( 0.000000000000000000, 0.08595325681623211533, 0.1695367914770939399, 0.2510169726856145700, 0.3324720360531058239, 0.4139176782331075444, 0.4946662699496591764, 0.5765962148649595997, 0.6610575120797289594, 0.7465372922784411225, 0.8302848992160567487, 0.9144215288650135998, 1.000000000000000000 ),
 .UNSPECIFIED. ) ;
#2750=EDGE_CURVE ( 'NONE', #8902, #9406, #1210, .T. ) ;
#2751=DIRECTION ( 'NONE',  ( -0.000000000000000000, 1.000000000000000000, -0.000000000000000000 ) ) ;
#2752=CARTESIAN_POINT ( 'NONE',  ( -27.43301270000000258, 3.899999998907525356, -11.36312591709336317 ) ) ;
#2754=EDGE_CURVE ( 'NONE', #728, #4302, #9837, .T. ) ;
#2755=CARTESIAN_POINT ( 'NONE',  ( 2.950788281418828429, 99.50000000000001421, -23.82341910423825837 ) ) ;
#2757=VECTOR ( 'NONE', #6777, 1000.000000000000000 ) ;
#2758=ORIENTED_EDGE ( 'NONE', *, *, #9480, .F. ) ;
#2760=CARTESIAN_POINT ( 'NONE',  ( -4.959819536546781389E-15, 5.199999997815050179, 27.00000000000000355 ) ) ;
#2761=ORIENTED_EDGE ( 'NONE', *, *, #6691, .F. ) ;
#2763=CARTESIAN_POINT ( 'NONE',  ( -20.96643530928959720, 99.50000000000001421, -10.05541671241505064 ) ) ;
#2766=CARTESIAN_POINT ( 'NONE',  ( 4.906732565843439531, 99.50000000000001421, -23.57187248890526376 ) ) ;
#2767=CARTESIAN_POINT ( 'NONE',  ( 0.000000000000000000, 85.00000000000000000, 0.000000000000000000 ) ) ;
#2771=VECTOR ( 'NONE', #2841, 1000.000000000000000 ) ;
#2772=CARTESIAN_POINT ( 'NONE',  ( 2.940192896829773250, 99.50000000000001421, -23.44521981770616037 ) ) ;
#2773=CARTESIAN_POINT ( 'NONE',  ( 11.36312591709336139, 1.999999998907525223, -27.43301270000000258 ) ) ;
#2776=CARTESIAN_POINT ( 'NONE',  ( 0.000000000000000000, 100.0000000000000000, 0.000000000000000000 ) ) ;
#2777=FACE_OUTER_BOUND ( 'NONE', #6425, .T. ) ;
#2778=CARTESIAN_POINT ( 'NONE',  ( -27.00000000000000355, 4.199999997815050179, -3.306546357697854128E-15 ) ) ;
#2779=CARTESIAN_POINT ( 'NONE',  ( -21.39817337045129619, 99.99999999999994316, -9.317726141196148504 ) ) ;
#2780=CARTESIAN_POINT ( 'NONE',  ( 4.835062408351179286, 99.50000000000000000, -21.79588013901878440 ) ) ;
#2782=CARTESIAN_POINT ( 'NONE',  ( 9.583828860305853681, 99.49999999999998579, 20.68614437522342797 ) ) ;
#2783=CARTESIAN_POINT ( 'NONE',  ( 9.513000527211589841, 100.0000000000000000, 20.35102222961602436 ) ) ;
#2784=CARTESIAN_POINT ( 'NONE',  ( 3.252389375388976323, 99.50000000000004263, -22.22144413113850447 ) ) ;
#2785=AXIS2_PLACEMENT_3D ( 'NONE', #3634, #7712, #6816 ) ;
#2788=ORIENTED_EDGE ( 'NONE', *, *, #2224, .F. ) ;
#2789=CARTESIAN_POINT ( 'NONE',  ( -15.98323291606820362, 99.99999999999998579, 16.64087298452848884 ) ) ;
#2792=ORIENTED_EDGE ( 'NONE', *, *, #1792, .T. ) ;
#2793=EDGE_CURVE ( 'NONE', #3366, #224, #2389, .T. ) ;
#2794=CARTESIAN_POINT ( 'NONE',  ( -22.17094027205346052, 99.50000000000001421, -9.884352203306939089 ) ) ;
#2795=CARTESIAN_POINT ( 'NONE',  ( -27.43301270000000969, 0.6999999989075252893, 11.36312591709335784 ) ) ;
#2796=LINE ( 'NONE', #9804, #7216 ) ;
#2797=CARTESIAN_POINT ( 'NONE',  ( -15.22739782325755442, 99.99999999999998579, 15.50750051783781025 ) ) ;
#2799=CARTESIAN_POINT ( 'NONE',  ( 0.000000000000000000, 85.00000000000000000, -25.15000000000000213 ) ) ;
#2801=EDGE_CURVE ( 'NONE', #4986, #6736, #4565, .T. ) ;
#2804=VERTEX_POINT ( 'NONE', #5968 ) ;
#2805=CARTESIAN_POINT ( 'NONE',  ( 26.99999999999999645, 1.349999997815050312, 11.18376618407358691 ) ) ;
#2807=CARTESIAN_POINT ( 'NONE',  ( -19.39806930854667755, 4.649999998907525800, -19.39806930854668110 ) ) ;
#2809=VECTOR ( 'NONE', #1255, 1000.000000000000114 ) ;
#2810=LINE ( 'NONE', #3649, #2757 ) ;
#2811=ORIENTED_EDGE ( 'NONE', *, *, #2261, .T. ) ;
#2815=DIRECTION ( 'NONE',  ( 0.2907756355032780071, 0.000000000000000000, 0.9567912676219745283 ) ) ;
#2816=CARTESIAN_POINT ( 'NONE',  ( -16.36254897777739004, 99.50000000000001421, 15.39785597259249350 ) ) ;
#2817=CARTESIAN_POINT ( 'NONE',  ( 3.573144549190039321, 99.99999999999998579, -23.04580706645134214 ) ) ;
#2818=EDGE_CURVE ( 'NONE', #6584, #7275, #10319, .T. ) ;
#2819=EDGE_LOOP ( 'NONE', ( #8359, #4591, #5070, #10010 ) ) ;
#2820=CARTESIAN_POINT ( 'NONE',  ( 4.773458297025112707, 100.0000000000000142, -24.02094923175124208 ) ) ;
#2821=CARTESIAN_POINT ( 'NONE',  ( -27.43301270000000258, 2.349999998907525534, -3.359575119402369376E-15 ) ) ;
#2822=ORIENTED_EDGE ( 'NONE', *, *, #10192, .F. ) ;
#2823=B_SPLINE_CURVE_WITH_KNOTS ( 'NONE', 3,
 ( #9488, #8016, #9681, #3301, #5609, #896, #2312, #5512, #4037, #4765, #4085, #1523, #8062, #4716, #1679 ),
 .UNSPECIFIED., .F., .F.,
 ( 4, 1, 1, 1, 1, 1, 1, 1, 1, 1, 1, 1, 4 ),
 ( 0.000000000000000000, 0.08595325681623211533, 0.1695367914770939399, 0.2510169726856145700, 0.3324720360531058239, 0.4139176782331075444, 0.4946662699496591764, 0.5765962148649595997, 0.6610575120797289594, 0.7465372922784411225, 0.8302848992160567487, 0.9144215288650135998, 1.000000000000000000 ),
 .UNSPECIFIED. ) ;
#2828=CARTESIAN_POINT ( 'NONE',  ( -27.43301270000000258, 2.999999998907525445, -11.36312591709336317 ) ) ;
#2829=DIRECTION ( 'NONE',  ( 0.000000000000000000, 1.000000000000000000, 0.000000000000000000 ) ) ;
#2831=CARTESIAN_POINT ( 'NONE',  ( 3.888553205800344248, 99.99999999999995737, -24.35333287445124739 ) ) ;
#2836=ORIENTED_EDGE ( 'NONE', *, *, #6874, .F. ) ;
#2838=CARTESIAN_POINT ( 'NONE',  ( 27.43301270000000258, 3.499999998907525445, -11.36312591709336139 ) ) ;
#2840=LINE ( 'NONE', #8436, #7947 ) ;
#2841=DIRECTION ( 'NONE',  ( -0.000000000000000000, 1.000000000000000000, -0.000000000000000000 ) ) ;
#2842=ORIENTED_EDGE ( 'NONE', *, *, #1493, .T. ) ;
#2843=CARTESIAN_POINT ( 'NONE',  ( 6.246869686064662197, 100.0000000000000000, 20.92172973853146090 ) ) ;
#2845=ORIENTED_EDGE ( 'NONE', *, *, #4349, .T. ) ;
#2846=CARTESIAN_POINT ( 'NONE',  ( -22.21584973381871464, 99.99999999999998579, -9.938501092090024969 ) ) ;
#2848=CARTESIAN_POINT ( 'NONE',  ( -27.00000000000001421, 5.049999997815051600, 11.18376618407356560 ) ) ;
#2849=CARTESIAN_POINT ( 'NONE',  ( 4.988497440555089923, 100.0000000000000284, -24.29977663856455194 ) ) ;
#2850=EDGE_CURVE ( 'NONE', #7023, #8336, #5348, .T. ) ;
#2854=CARTESIAN_POINT ( 'NONE',  ( 7.486453019397995234, 99.50000000000000000, 23.81666162955709964 ) ) ;
#2855=ORIENTED_EDGE ( 'NONE', *, *, #2909, .F. ) ;
#2857=CARTESIAN_POINT ( 'NONE',  ( 27.43301270000000258, 4.349999998907525089, 0.000000000000000000 ) ) ;
#2858=CARTESIAN_POINT ( 'NONE',  ( 3.282077632710153292, 99.50000000000000000, -23.74569985055724786 ) ) ;
#2859=CARTESIAN_POINT ( 'NONE',  ( 9.881472129446523311, 100.0000000000000142, 20.94326683228310060 ) ) ;
#2863=CARTESIAN_POINT ( 'NONE',  ( -21.59614764830937972, 100.0000000000000142, -9.292069227195950631 ) ) ;
#2864=CARTESIAN_POINT ( 'NONE',  ( 5.047889085735837611, 99.50000000000001421, -24.22022158424849536 ) ) ;
#2865=CARTESIAN_POINT ( 'NONE',  ( 19.09188309203678813, 3.299999999999999822, -19.09188309203678813 ) ) ;
#2866=DIRECTION ( 'NONE',  ( 0.000000000000000000, 0.000000000000000000, -1.000000000000000000 ) ) ;
#2868=ORIENTED_EDGE ( 'NONE', *, *, #521, .F. ) ;
#2869=CARTESIAN_POINT ( 'NONE',  ( -16.56928979259283352, 99.50000000000002842, 16.65656195153832897 ) ) ;
#2871=CARTESIAN_POINT ( 'NONE',  ( -11.36312591709335962, 2.199999998907525622, -27.43301270000000258 ) ) ;
#2872=ORIENTED_EDGE ( 'NONE', *, *, #5787, .F. ) ;
#2874=CARTESIAN_POINT ( 'NONE',  ( 3.428579745388047328, 99.99999999999995737, -21.16399209792802694 ) ) ;
#2876=CARTESIAN_POINT ( 'NONE',  ( 1.679787559701184688E-15, 4.449999998907525622, -27.43301270000000258 ) ) ;
#2877=VERTEX_POINT ( 'NONE', #2359 ) ;
#2878=CARTESIAN_POINT ( 'NONE',  ( 19.39806930854668110, 2.049999998907525711, -19.39806930854668110 ) ) ;
#2879=ORIENTED_EDGE ( 'NONE', *, *, #1907, .T. ) ;
#2880=VERTEX_POINT ( 'NONE', #2311 ) ;
#2882=CARTESIAN_POINT ( 'NONE',  ( 9.526349065647009340, 100.0000000000000000, 19.81320455978211470 ) ) ;
#2884=CARTESIAN_POINT ( 'NONE',  ( 5.725936192474917696, 100.0000000000000000, 21.08018326417248645 ) ) ;
#2885=CARTESIAN_POINT ( 'NONE',  ( 3.810791133452845703, 100.0000000000000568, -24.33305202239136733 ) ) ;
#2887=CARTESIAN_POINT ( 'NONE',  ( 3.195700652717397894, 99.99999999999997158, -22.66286045753255962 ) ) ;
#2888=ORIENTED_EDGE ( 'NONE', *, *, #966, .F. ) ;
#2889=LINE ( 'NONE', #2946, #7395 ) ;
#2890=CARTESIAN_POINT ( 'NONE',  ( -11.36312591709337383, 1.599999998907525534, 27.43301269999999548 ) ) ;
#2892=CARTESIAN_POINT ( 'NONE',  ( 27.43301270000000258, 0.2999999989075251561, 0.000000000000000000 ) ) ;
#2893=EDGE_CURVE ( 'NONE', #669, #7666, #7065, .T. ) ;
#2894=CARTESIAN_POINT ( 'NONE',  ( -19.09188309203678457, 0.3000000000000000444, -19.09188309203678813 ) ) ;
#2895=CARTESIAN_POINT ( 'NONE',  ( 9.245739950628269810, 100.0000000000000568, 20.03726560014620617 ) ) ;
#2896=VERTEX_POINT ( 'NONE', #1362 ) ;
#2897=ORIENTED_EDGE ( 'NONE', *, *, #6076, .T. ) ;
#2898=CARTESIAN_POINT ( 'NONE',  ( 4.739008722453744049, 100.0000000000000142, -24.06821587619827696 ) ) ;
#2901=EDGE_LOOP ( 'NONE', ( #5884, #1557, #3818, #6823, #2249, #732, #8229, #3585 ) ) ;
#2902=CARTESIAN_POINT ( 'NONE',  ( -22.06741020400400188, 99.50000000000004263, -9.788922322134999021 ) ) ;
#2903=CARTESIAN_POINT ( 'NONE',  ( -15.45548338988150938, 99.99999999999997158, 16.93306818456458984 ) ) ;
#2904=CARTESIAN_POINT ( 'NONE',  ( -20.96643530928959365, 99.50000000000000000, -10.05541671241504886 ) ) ;
#2906=CARTESIAN_POINT ( 'NONE',  ( 5.098880966732203035, 100.0000000000000284, -24.13374913903897223 ) ) ;
#2907=ORIENTED_EDGE ( 'NONE', *, *, #9087, .F. ) ;
#2908=CARTESIAN_POINT ( 'NONE',  ( 4.504418077186241653, 99.50000000000004263, -21.31258943653750393 ) ) ;
#2909=EDGE_CURVE ( 'NONE', #7789, #969, #1804, .T. ) ;
#2911=CARTESIAN_POINT ( 'NONE',  ( 9.526713201929464248, 100.0000000000000000, 20.38668308130821671 ) ) ;
#2912=ORIENTED_EDGE ( 'NONE', *, *, #8427, .F. ) ;
#2914=CARTESIAN_POINT ( 'NONE',  ( 19.39806930854668110, 4.449999998907525622, -19.39806930854668110 ) ) ;
#2916=CARTESIAN_POINT ( 'NONE',  ( 9.897596448871711416, 99.49999999999998579, 20.85734708541456328 ) ) ;
#2918=B_SPLINE_SURFACE_WITH_KNOTS ( 'NONE', 3, 1, ( 
 ( #3415, #2590 ),
 ( #9853, #4163 ),
 ( #5781, #6610 ),
 ( #7439, #1795 ),
 ( #9905, #8188 ),
 ( #1016, #8285 ),
 ( #5926, #4208 ),
 ( #4258, #1118 ),
 ( #1746, #2689 ),
 ( #4308, #2639 ),
 ( #9023, #5831 ),
 ( #1840, #5878 ),
 ( #7347, #7392 ),
 ( #7493, #5035 ),
 ( #9077, #4942 ),
 ( #1066, #183 ),
 ( #6563, #8235 ),
 ( #3369, #9754 ),
 ( #332, #7545 ) ),
 .UNSPECIFIED., .F., .F., .F.,
 ( 4, 1, 1, 1, 1, 1, 1, 1, 1, 1, 1, 1, 1, 1, 1, 1, 4 ),
 ( 2, 2 ),
 ( 0.000000000000000000, 0.05935611633690887623, 0.1167563879513689451, 0.1743885027374874330, 0.2308223543163396840, 0.2888100779544915953, 0.3475404098195560842, 0.4086537266250744316, 0.4723446836969566465, 0.5362968130936018873, 0.6000923674009760456, 0.6637702377379335328, 0.7274568328636339398, 0.7924602533659969028, 0.8590386936388050287, 0.9283644560612371865, 1.000000000000000000 ),
 ( 0.000000000000000000, 1.000000000000000000 ),
 .UNSPECIFIED. ) ;
#2919=CARTESIAN_POINT ( 'NONE',  ( -16.07368679829020763, 99.50000000000000000, 17.11560437002838952 ) ) ;
#2924=CARTESIAN_POINT ( 'NONE',  ( -15.76955986605724647, 99.99999999999998579, 15.18352214517458698 ) ) ;
#2925=CARTESIAN_POINT ( 'NONE',  ( 27.43301269999999548, 2.699999998907525178, 11.36312591709337916 ) ) ;
#2927=EDGE_CURVE ( 'NONE', #9400, #1992, #951, .T. ) ;
#2929=AXIS2_PLACEMENT_3D ( 'NONE', #7685, #2990, #10209 ) ;
#2931=CARTESIAN_POINT ( 'NONE',  ( 9.502908418173033667, 99.50000000000000000, 20.32929868008965002 ) ) ;
#2934=CARTESIAN_POINT ( 'NONE',  ( 11.18376618407357093, 0.7499999978150503344, -27.00000000000000355 ) ) ;
#2935=CARTESIAN_POINT ( 'NONE',  ( 27.43301270000000258, 2.749999998907525445, 0.000000000000000000 ) ) ;
#2937=CARTESIAN_POINT ( 'NONE',  ( 9.806436918512124734, 99.99999999999998579, 20.18080982695387604 ) ) ;
#2938=CARTESIAN_POINT ( 'NONE',  ( 3.970307086022987431, 100.0000000000000142, -24.36314111580913178 ) ) ;
#2939=CARTESIAN_POINT ( 'NONE',  ( -16.36470918167357169, 99.50000000000000000, 16.79054296464299867 ) ) ;
#2940=AXIS2_PLACEMENT_3D ( 'NONE', #2776, #4147, #9782 ) ;
#2941=CARTESIAN_POINT ( 'NONE',  ( -15.76955986605724647, 99.99999999999998579, 15.18352214517458698 ) ) ;
#2942=EDGE_LOOP ( 'NONE', ( #2208, #5704 ) ) ;
#2944=CARTESIAN_POINT ( 'NONE',  ( 3.105863891863242632, 100.0000000000000142, -22.59672720503480292 ) ) ;
#2945=ORIENTED_EDGE ( 'NONE', *, *, #3693, .F. ) ;
#2946=CARTESIAN_POINT ( 'NONE',  ( 8.429066232339796017, 99.50000000000000000, 19.67794530653910101 ) ) ;
#2948=CARTESIAN_POINT ( 'NONE',  ( 11.36312591709336139, 3.599999998907525089, -27.43301270000000258 ) ) ;
#2952=CARTESIAN_POINT ( 'NONE',  ( -11.18376618407358336, 2.149999999999999911, 26.99999999999999645 ) ) ;
#2955=CARTESIAN_POINT ( 'NONE',  ( -15.22739782325755442, 99.49999999999998579, 15.50750051783781025 ) ) ;
#2956=CARTESIAN_POINT ( 'NONE',  ( -15.42956291708403782, 99.49999999999998579, 16.53061251458192515 ) ) ;
#2960=VERTEX_POINT ( 'NONE', #5756 ) ;
#2961=EDGE_CURVE ( 'NONE', #8960, #8911, #3691, .T. ) ;
#2962=CARTESIAN_POINT ( 'NONE',  ( 4.259295290443009918, 99.50000000000002842, -24.34414156132068996 ) ) ;
#2963=CARTESIAN_POINT ( 'NONE',  ( 11.36312591709336139, 0.3999999989075253559, -27.43301270000000258 ) ) ;
#2964=DIRECTION ( 'NONE',  ( -0.000000000000000000, 1.000000000000000000, -0.000000000000000000 ) ) ;
#2965=VECTOR ( 'NONE', #6660, 1000.000000000000000 ) ;
#2967=CARTESIAN_POINT ( 'NONE',  ( -19.09188309203678813, 3.700000000000000178, 19.09188309203678457 ) ) ;
#2969=CIRCLE ( 'NONE', #6312, 25.00000000000000000 ) ;
#2970=CARTESIAN_POINT ( 'NONE',  ( 4.034460619503033030, 99.49999999999995737, -21.08676866017170681 ) ) ;
#2972=DIRECTION ( 'NONE',  ( -0.9572638942369904314, 0.000000000000000000, 0.2892158999609669712 ) ) ;
#2974=CARTESIAN_POINT ( 'NONE',  ( -4.959819536546781389E-15, 1.199999997815050401, 27.00000000000000355 ) ) ;
#2977=CARTESIAN_POINT ( 'NONE',  ( 9.692323321704657602, 100.0000000000000000, 21.58969587442354410 ) ) ;
#2979=CARTESIAN_POINT ( 'NONE',  ( 1.653273178848927064E-15, 5.599999997815050534, -27.00000000000000355 ) ) ;
#2980=CARTESIAN_POINT ( 'NONE',  ( 8.857094148306096315, 99.50000000000001421, 19.57755665027156766 ) ) ;
#2982=CARTESIAN_POINT ( 'NONE',  ( -16.41302370085497131, 99.49999999999998579, 15.45185748370271206 ) ) ;
#2984=CARTESIAN_POINT ( 'NONE',  ( -16.36470918167357169, 100.0000000000000000, 16.79054296464299867 ) ) ;
#2985=CARTESIAN_POINT ( 'NONE',  ( -19.39806930854668465, 0.8499999989075252005, 19.39806930854667755 ) ) ;
#2986=VERTEX_POINT ( 'NONE', #2610 ) ;
#2990=DIRECTION ( 'NONE',  ( -0.000000000000000000, -1.000000000000000000, -0.000000000000000000 ) ) ;
#2992=CARTESIAN_POINT ( 'NONE',  ( -27.43301270000000258, 4.599999998907525978, -11.36312591709336317 ) ) ;
#2993=CARTESIAN_POINT ( 'NONE',  ( 27.43301269999999548, 3.499999998907525445, 11.36312591709337738 ) ) ;
#2994=ORIENTED_EDGE ( 'NONE', *, *, #4290, .T. ) ;
#2995=ORIENTED_EDGE ( 'NONE', *, *, #5638, .T. ) ;
#2998=CARTESIAN_POINT ( 'NONE',  ( -20.42657152723830905, 99.50000000000000000, -10.54129411626120216 ) ) ;
#3000=CARTESIAN_POINT ( 'NONE',  ( 21.82251602564102910, 100.0000000000000000, -0.5181290064102563875 ) ) ;
#3001=CARTESIAN_POINT ( 'NONE',  ( 3.551917533706515417, 99.50000000000001421, -21.11785906961830150 ) ) ;
#3002=CARTESIAN_POINT ( 'NONE',  ( 3.535161742238301041, 100.0000000000000142, -24.18247714022527006 ) ) ;
#3003=ORIENTED_EDGE ( 'NONE', *, *, #5646, .T. ) ;
#3005=CARTESIAN_POINT ( 'NONE',  ( 3.948639947730041566, 99.99999999999998579, -21.07692942975820927 ) ) ;
#3008=CARTESIAN_POINT ( 'NONE',  ( -5.039362679103552881E-15, 1.649999998907525134, 27.43301270000000258 ) ) ;
#3010=CARTESIAN_POINT ( 'NONE',  ( -4.959819536546781389E-15, 3.000000000000000000, 27.00000000000000355 ) ) ;
#3011=CARTESIAN_POINT ( 'NONE',  ( 27.00000000000000355, 0.05000000000000000278, -11.18376618407356737 ) ) ;
#3012=CARTESIAN_POINT ( 'NONE',  ( 2.852289972453743161, 99.50000000000000000, -22.14293542748032451 ) ) ;
#3014=CARTESIAN_POINT ( 'NONE',  ( -16.52319226728147328, 99.49999999999998579, 15.63609008536095324 ) ) ;
#3015=CARTESIAN_POINT ( 'NONE',  ( -15.69015368034045643, 100.0000000000000142, 16.64011368054243434 ) ) ;
#3021=LINE ( 'NONE', #3071, #3525 ) ;
#3025=CARTESIAN_POINT ( 'NONE',  ( 5.047889085735837611, 100.0000000000000426, -24.22022158424849536 ) ) ;
#3027=EDGE_CURVE ( 'NONE', #9293, #647, #203, .T. ) ;
#3031=CARTESIAN_POINT ( 'NONE',  ( 1.653273178848927064E-15, 2.600000000000000533, -27.00000000000000355 ) ) ;
#3032=ORIENTED_EDGE ( 'NONE', *, *, #624, .T. ) ;
#3033=CARTESIAN_POINT ( 'NONE',  ( 9.676361905416719367, 100.0000000000000000, 21.63547735782115211 ) ) ;
#3035=EDGE_CURVE ( 'NONE', #6279, #2600, #10191, .T. ) ;
#3036=DIRECTION ( 'NONE',  ( -0.000000000000000000, 1.000000000000000000, -0.000000000000000000 ) ) ;
#3038=CARTESIAN_POINT ( 'NONE',  ( -16.52319226728147328, 99.49999999999998579, 15.63609008536095324 ) ) ;
#3040=CARTESIAN_POINT ( 'NONE',  ( -16.33590634957226229, 99.50000000000000000, 16.80570853669505382 ) ) ;
#3041=CARTESIAN_POINT ( 'NONE',  ( -27.43301270000000258, 0.7499999989075251117, -3.359575119402369376E-15 ) ) ;
#3042=VERTEX_POINT ( 'NONE', #8992 ) ;
#3046=CARTESIAN_POINT ( 'NONE',  ( 27.43301270000000258, 5.099999998907525978, -11.36312591709336139 ) ) ;
#3047=CARTESIAN_POINT ( 'NONE',  ( -27.43301270000000258, 2.349999998907525534, -3.359575119402369376E-15 ) ) ;
#3048=CARTESIAN_POINT ( 'NONE',  ( 9.666415885916139317, 100.0000000000000142, 19.95264712196244261 ) ) ;
#3054=ORIENTED_EDGE ( 'NONE', *, *, #6738, .T. ) ;
#3057=CARTESIAN_POINT ( 'NONE',  ( -27.43301270000000258, 1.399999998907525134, -11.36312591709336317 ) ) ;
#3058=DIRECTION ( 'NONE',  ( 0.000000000000000000, 1.000000000000000000, 0.000000000000000000 ) ) ;
#3060=CARTESIAN_POINT ( 'NONE',  ( -27.00000000000000355, 0.3499999999999999778, -11.18376618407357093 ) ) ;
#3061=CARTESIAN_POINT ( 'NONE',  ( 9.182805720491336032, 100.0000000000000284, 20.00174565872165289 ) ) ;
#3062=ORIENTED_EDGE ( 'NONE', *, *, #3625, .F. ) ;
#3063=( BOUNDED_CURVE ( )  B_SPLINE_CURVE ( 2, ( #941, #4134, #7317, #155, #9191, #9980, #2865, #8356, #2129 ),
 .UNSPECIFIED., .F., .F. ) 
 B_SPLINE_CURVE_WITH_KNOTS ( ( 3, 2, 2, 2, 3 ),
 ( 0.5357142857142856984, 0.5535714285714286031, 0.5714285714285713969, 0.5892857142857143016, 0.6071428571428570953 ),
 .UNSPECIFIED. ) 
 CURVE ( )  GEOMETRIC_REPRESENTATION_ITEM ( )  RATIONAL_B_SPLINE_CURVE ( ( 1.000000000000000000, 0.9238795325112867385, 1.000000000000000000, 0.9238795325112867385, 1.000000000000000000, 0.9238795325112867385, 1.000000000000000000, 0.9238795325112867385, 1.000000000000000000 ) ) 
 REPRESENTATION_ITEM ( '' )  );
#3064=LINE ( 'NONE', #1434, #8339 ) ;
#3065=CARTESIAN_POINT ( 'NONE',  ( -15.76250887235353737, 99.99999999999998579, 16.65066592061022277 ) ) ;
#3067=ORIENTED_EDGE ( 'NONE', *, *, #2486, .F. ) ;
#3068=ORIENTED_EDGE ( 'NONE', *, *, #8817, .T. ) ;
#3070=CARTESIAN_POINT ( 'NONE',  ( 19.39806930854667399, 4.149999998907525800, 19.39806930854668465 ) ) ;
#3071=CARTESIAN_POINT ( 'NONE',  ( -16.07368679829020763, 99.50000000000000000, 17.11560437002838952 ) ) ;
#3079=CARTESIAN_POINT ( 'NONE',  ( 4.633286773149219329, 100.0000000000000284, -21.44575434969419447 ) ) ;
#3080=CARTESIAN_POINT ( 'NONE',  ( -15.07178375341841381, 99.50000000000000000, 16.66969090848992607 ) ) ;
#3081=ORIENTED_EDGE ( 'NONE', *, *, #9187, .F. ) ;
#3083=CARTESIAN_POINT ( 'NONE',  ( 8.961048541867139505, 99.50000000000001421, 19.57961630251783092 ) ) ;
#3087=CARTESIAN_POINT ( 'NONE',  ( -21.96365545856212265, 100.0000000000000142, -9.726658277667754149 ) ) ;
#3088=CARTESIAN_POINT ( 'NONE',  ( 9.666415885916139317, 99.50000000000001421, 19.95264712196244261 ) ) ;
#3090=CARTESIAN_POINT ( 'NONE',  ( -22.31230063665282515, 99.49999999999997158, -10.62159318200525249 ) ) ;
#3091=EDGE_CURVE ( 'NONE', #1371, #7818, #8081, .T. ) ;
#3092=EDGE_LOOP ( 'NONE', ( #3195, #6140, #2450, #3081, #1778, #8606 ) ) ;
#3093=CARTESIAN_POINT ( 'NONE',  ( -14.78677372028383097, 99.49999999999998579, 15.63810349997947569 ) ) ;
#3094=CARTESIAN_POINT ( 'NONE',  ( -11.36312591709337561, 4.099999998907525089, 27.43301269999999548 ) ) ;
#3098=CARTESIAN_POINT ( 'NONE',  ( 3.252389375388976323, 100.0000000000000426, -22.22144413113850447 ) ) ;
#3100=CARTESIAN_POINT ( 'NONE',  ( 4.750280232731688201, 99.50000000000002842, -24.05275076595185624 ) ) ;
#3101=CARTESIAN_POINT ( 'NONE',  ( -27.43301270000000969, 1.599999998907525534, 11.36312591709335429 ) ) ;
#3104=FACE_OUTER_BOUND ( 'NONE', #6266, .T. ) ;
#3105=LINE ( 'NONE', #7960, #3318 ) ;
#3107=B_SPLINE_SURFACE_WITH_KNOTS ( 'NONE', 3, 1, ( 
 ( #5974, #9166 ),
 ( #10004, #1986 ),
 ( #4406, #9012 ),
 ( #7589, #427 ),
 ( #3406, #5234 ),
 ( #5026, #4248 ),
 ( #1320, #6077 ),
 ( #7865, #1266 ),
 ( #6186, #9326 ),
 ( #2319, #6297 ),
 ( #3888, #3677 ),
 ( #3839, #6860 ),
 ( #4455, #540 ),
 ( #4509, #7024 ),
 ( #9268, #7076 ) ),
 .UNSPECIFIED., .F., .F., .F.,
 ( 4, 1, 1, 1, 1, 1, 1, 1, 1, 1, 1, 1, 4 ),
 ( 2, 2 ),
 ( 0.000000000000000000, 0.08635447908391848115, 0.1695936995346988552, 0.2509241109261274860, 0.3325843554298174576, 0.4138183564518133073, 0.4948404748415979881, 0.5772065644957810049, 0.6619893985813737336, 0.7474108716807353892, 0.8313115314839791825, 0.9147691218156368542, 1.000000000000000000 ),
 ( 0.000000000000000000, 1.000000000000000000 ),
 .UNSPECIFIED. ) ;
#3110=CARTESIAN_POINT ( 'NONE',  ( -21.89277277937676303, 99.49999999999998579, -9.329958722595300458 ) ) ;
#3112=ORIENTED_EDGE ( 'NONE', *, *, #1493, .F. ) ;
#3114=CARTESIAN_POINT ( 'NONE',  ( -11.36312591709335962, 2.199999998907525622, -27.43301270000000258 ) ) ;
#3115=CARTESIAN_POINT ( 'NONE',  ( 0.000000000000000000, 5.000000000000004441, -27.00000000000000355 ) ) ;
#3116=CARTESIAN_POINT ( 'NONE',  ( -19.09188309203678457, 1.100000000000000089, -19.09188309203678813 ) ) ;
#3118=ORIENTED_EDGE ( 'NONE', *, *, #1609, .F. ) ;
#3119=VECTOR ( 'NONE', #6845, 1000.000000000000000 ) ;
#3120=CARTESIAN_POINT ( 'NONE',  ( -16.54512803120131181, 99.50000000000000000, 16.13427955854364626 ) ) ;
#3121=CARTESIAN_POINT ( 'NONE',  ( 8.399337394135656609, 99.49999999999998579, 20.06291166101774692 ) ) ;
#3123=VERTEX_POINT ( 'NONE', #3655 ) ;
#3124=CARTESIAN_POINT ( 'NONE',  ( -27.43301270000000258, 3.049999998907525267, -3.359575119402369376E-15 ) ) ;
#3127=CARTESIAN_POINT ( 'NONE',  ( -11.18376618407358336, 1.949999997815050401, 26.99999999999999645 ) ) ;
#3130=ADVANCED_FACE ( 'NONE', ( #3543 ), #6629, .T. ) ;
#3132=VECTOR ( 'NONE', #4793, 1000.000000000000000 ) ;
#3133=CARTESIAN_POINT ( 'NONE',  ( 4.691018317478480526, 99.99999999999995737, -21.52316599815148024 ) ) ;
#3134=CARTESIAN_POINT ( 'NONE',  ( -15.89341924297059094, 100.0000000000000142, 17.07725933521297890 ) ) ;
#3137=ORIENTED_EDGE ( 'NONE', *, *, #3357, .T. ) ;
#3141=LINE ( 'NONE', #10259, #10184 ) ;
#3144=CARTESIAN_POINT ( 'NONE',  ( -27.43301270000000969, 4.799999998907525267, 11.36312591709335784 ) ) ;
#3146=APPLICATION_CONTEXT ( 'automotive_design' ) ;
#3151=CARTESIAN_POINT ( 'NONE',  ( -20.91430522584054330, 100.0000000000000142, -10.19152558580213608 ) ) ;
#3154=CARTESIAN_POINT ( 'NONE',  ( -20.89884294283097432, 99.50000000000001421, -10.47119744953613640 ) ) ;
#3155=CARTESIAN_POINT ( 'NONE',  ( 27.00000000000000355, 1.449999997815050401, -11.18376618407356737 ) ) ;
#3156=CARTESIAN_POINT ( 'NONE',  ( -15.10687288066601930, 99.49999999999998579, 15.84109048427130517 ) ) ;
#3157=CARTESIAN_POINT ( 'NONE',  ( 3.478562133589548910, 99.99999999999997158, -24.13114810667639532 ) ) ;
#3158=CARTESIAN_POINT ( 'NONE',  ( 3.214822648120007731, 99.50000000000000000, -21.86319392453323829 ) ) ;
#3161=CARTESIAN_POINT ( 'NONE',  ( 4.034460619503033030, 99.99999999999995737, -21.08676866017170681 ) ) ;
#3163=CARTESIAN_POINT ( 'NONE',  ( -11.36312591709337383, 4.799999998907525267, 27.43301269999999548 ) ) ;
#3165=CARTESIAN_POINT ( 'NONE',  ( 4.154273145530666511, 99.50000000000000000, -22.82723029927519676 ) ) ;
#3166=CARTESIAN_POINT ( 'NONE',  ( -27.00000000000000355, 2.799999999999999822, -3.306546357697854128E-15 ) ) ;
#3167=VECTOR ( 'NONE', #8931, 1000.000000000000000 ) ;
#3169=CARTESIAN_POINT ( 'NONE',  ( 8.081885929396888102, 100.0000000000000142, 20.89785832093561169 ) ) ;
#3173=FACE_OUTER_BOUND ( 'NONE', #8422, .T. ) ;
#3174=CARTESIAN_POINT ( 'NONE',  ( 19.39806930854668110, 1.149999998907525356, -19.39806930854668110 ) ) ;
#3175=CARTESIAN_POINT ( 'NONE',  ( 3.238942592553923472, 100.0000000000000142, -24.36085717291697250 ) ) ;
#3176=CARTESIAN_POINT ( 'NONE',  ( -22.51488550592518934, 99.49999999999997158, -10.97145172607810615 ) ) ;
#3178=CARTESIAN_POINT ( 'NONE',  ( 0.000000000000000000, 100.0000000000000000, -27.00000000000000355 ) ) ;
#3179=CARTESIAN_POINT ( 'NONE',  ( 9.802580223201115217, 99.99999999999995737, 21.25247094773282086 ) ) ;
#3180=DIRECTION ( 'NONE',  ( 0.000000000000000000, 1.000000000000000000, 0.000000000000000000 ) ) ;
#3182=CARTESIAN_POINT ( 'NONE',  ( 10.85214315541671759, 99.50000000000000000, 22.51047735782115211 ) ) ;
#3187=EDGE_CURVE ( 'NONE', #9293, #4730, #7657, .T. ) ;
#3190=CARTESIAN_POINT ( 'NONE',  ( -22.34867803760930727, 99.99999999999998579, -10.48295844864103721 ) ) ;
#3191=ORIENTED_EDGE ( 'NONE', *, *, #6377, .T. ) ;
#3193=CARTESIAN_POINT ( 'NONE',  ( -14.89508182811745662, 99.49999999999997158, 15.38112983991209326 ) ) ;
#3194=CARTESIAN_POINT ( 'NONE',  ( -5.039362679103552881E-15, 3.349999998907525534, 27.43301270000000258 ) ) ;
#3195=ORIENTED_EDGE ( 'NONE', *, *, #6715, .F. ) ;
#3198=CARTESIAN_POINT ( 'NONE',  ( 3.282077632710153292, 99.99999999999997158, -23.74569985055724786 ) ) ;
#3201=CARTESIAN_POINT ( 'NONE',  ( 1.679787559701184688E-15, 5.349999998907525089, -27.43301270000000258 ) ) ;
#3202=CARTESIAN_POINT ( 'NONE',  ( -20.42657152723830905, 99.50000000000000000, -10.54129411626120216 ) ) ;
#3203=CARTESIAN_POINT ( 'NONE',  ( 3.597125852879613728, 99.99999999999998579, -24.22990373345680126 ) ) ;
#3207=CARTESIAN_POINT ( 'NONE',  ( 3.861186820804014097, 100.0000000000000426, -21.07288982789904708 ) ) ;
#3208=VERTEX_POINT ( 'NONE', #6144 ) ;
#3209=VERTEX_POINT ( 'NONE', #6871 ) ;
#3211=CARTESIAN_POINT ( 'NONE',  ( 27.43301270000000258, 1.949999998907525178, 0.000000000000000000 ) ) ;
#3212=CARTESIAN_POINT ( 'NONE',  ( 6.246869686064662197, 99.50000000000000000, 20.92172973853146090 ) ) ;
#3213=B_SPLINE_CURVE_WITH_KNOTS ( 'NONE', 3,
 ( #91, #9467, #1558, #2296, #8682, #8782, #10358, #7891, #9567, #5593, #1607 ),
 .UNSPECIFIED., .F., .F.,
 ( 4, 1, 1, 1, 1, 1, 1, 1, 4 ),
 ( 0.000000000000000000, 0.1307887167449866828, 0.2576322083635017579, 0.3824781763252146916, 0.5056045358258490774, 0.6278910088851102911, 0.7502354365656509483, 0.8735741898580190457, 1.000000000000000000 ),
 .UNSPECIFIED. ) ;
#3214=CARTESIAN_POINT ( 'NONE',  ( 11.36312591709336139, 0.3999999989075253559, -27.43301270000000258 ) ) ;
#3217=CARTESIAN_POINT ( 'NONE',  ( -21.24310748994415832, 99.99999999999995737, -10.99527971241054658 ) ) ;
#3219=CARTESIAN_POINT ( 'NONE',  ( 11.36312591709336850, 4.099999998907525089, 27.43301269999999903 ) ) ;
#3220=CARTESIAN_POINT ( 'NONE',  ( -11.18376618407356737, 1.850000000000000311, -27.00000000000000355 ) ) ;
#3221=VECTOR ( 'NONE', #659, 1000.000000000000000 ) ;
#3222=ADVANCED_FACE ( 'NONE', ( #8670 ), #7771, .T. ) ;
#3223=CARTESIAN_POINT ( 'NONE',  ( 1.653273178848927064E-15, 0.7999999978150503788, -27.00000000000000355 ) ) ;
#3225=CARTESIAN_POINT ( 'NONE',  ( -19.09188309203678813, 1.899999997815050579, 19.09188309203678457 ) ) ;
#3226=CARTESIAN_POINT ( 'NONE',  ( -22.64023588676181475, 100.0000000000000000, -10.01165679465830927 ) ) ;
#3227=CARTESIAN_POINT ( 'NONE',  ( 4.688812652749139609, 100.0000000000000142, -24.54863390154074310 ) ) ;
#3228=VECTOR ( 'NONE', #7194, 1000.000000000000000 ) ;
#3230=EDGE_LOOP ( 'NONE', ( #4585, #8662, #7224, #2517, #2543, #3909, #298, #8196 ) ) ;
#3232=CARTESIAN_POINT ( 'NONE',  ( -15.34367147589386349, 100.0000000000000426, 16.87599331055909602 ) ) ;
#3233=LINE ( 'NONE', #2444, #1373 ) ;
#3236=ORIENTED_EDGE ( 'NONE', *, *, #9066, .F. ) ;
#3237=CARTESIAN_POINT ( 'NONE',  ( -22.29247428061501779, 100.0000000000000000, -10.66603791136541624 ) ) ;
#3238=VERTEX_POINT ( 'NONE', #4519 ) ;
#3239=DIRECTION ( 'NONE',  ( 0.9789429660840185399, 0.000000000000000000, -0.2041339490496966447 ) ) ;
#3240=CARTESIAN_POINT ( 'NONE',  ( -14.79004890936967875, 99.49999999999998579, 16.19006955939758541 ) ) ;
#3241=VECTOR ( 'NONE', #2751, 1000.000000000000000 ) ;
#3242=CARTESIAN_POINT ( 'NONE',  ( 27.43301269999999548, 4.299999998907526155, 11.36312591709337916 ) ) ;
#3244=CARTESIAN_POINT ( 'NONE',  ( 4.128176300878408256, 99.50000000000001421, -21.47174600747824869 ) ) ;
#3245=CARTESIAN_POINT ( 'NONE',  ( -20.89145576992255116, 99.99999999999997158, -10.33073932272468198 ) ) ;
#3247=CARTESIAN_POINT ( 'NONE',  ( -20.45905772418405988, 100.0000000000000000, -10.59533404166311321 ) ) ;
#3248=CARTESIAN_POINT ( 'NONE',  ( 1.653273178848927064E-15, 1.599999997815050312, -27.00000000000000355 ) ) ;
#3250=FACE_OUTER_BOUND ( 'NONE', #5456, .T. ) ;
#3251=CARTESIAN_POINT ( 'NONE',  ( -15.33577160963320374, 99.49999999999998579, 16.45272793336155814 ) ) ;
#3252=EDGE_CURVE ( 'NONE', #3431, #2986, #8934, .T. ) ;
#3255=CARTESIAN_POINT ( 'NONE',  ( 9.576498344683301411, 99.99999999999998579, 20.78592410672095880 ) ) ;
#3259=CARTESIAN_POINT ( 'NONE',  ( 19.39806930854667399, 4.149999998907525800, 19.39806930854668465 ) ) ;
#3260=CARTESIAN_POINT ( 'NONE',  ( -15.24337324910153946, 99.49999999999997158, 16.81353386054630761 ) ) ;
#3261=CARTESIAN_POINT ( 'NONE',  ( 26.99999999999999645, 3.150000000000000355, 11.18376618407358691 ) ) ;
#3263=CYLINDRICAL_SURFACE ( 'NONE', #4380, 27.00000000000000355 ) ;
#3265=CARTESIAN_POINT ( 'NONE',  ( 4.750280232731688201, 100.0000000000000284, -24.05275076595185624 ) ) ;
#3267=CARTESIAN_POINT ( 'NONE',  ( 27.43301270000000258, 4.249999998907525445, 0.000000000000000000 ) ) ;
#3268=CARTESIAN_POINT ( 'NONE',  ( 2.940631318607589417, 99.50000000000000000, -23.77584808773673331 ) ) ;
#3269=B_SPLINE_SURFACE_WITH_KNOTS ( 'NONE', 3, 1, ( 
 ( #5763, #5014 ),
 ( #8951, #8211 ),
 ( #1819, #361 ),
 ( #3395, #1197 ),
 ( #5168, #5904 ),
 ( #8367, #1043 ),
 ( #4389, #4285 ),
 ( #9100, #3551 ),
 ( #9831, #4237 ),
 ( #6740, #2569 ),
 ( #7469, #6587 ),
 ( #7574, #3498 ),
 ( #1868, #2663 ),
 ( #7418, #258 ),
 ( #8264, #8164 ) ),
 .UNSPECIFIED., .F., .F., .F.,
 ( 4, 1, 1, 1, 1, 1, 1, 1, 1, 1, 1, 1, 4 ),
 ( 2, 2 ),
 ( 0.000000000000000000, 0.08490232564366416435, 0.1680779112633816463, 0.2506304657828534177, 0.3338427399641299420, 0.4169763759729993580, 0.4990117930239920674, 0.5811067191809071719, 0.6656374296971073745, 0.7500328835558887075, 0.8331455368193440014, 0.9159638734519762737, 1.000000000000000000 ),
 ( 0.000000000000000000, 1.000000000000000000 ),
 .UNSPECIFIED. ) ;
#3272=CARTESIAN_POINT ( 'NONE',  ( 2.852289972453743161, 100.0000000000000000, -22.14293542748032451 ) ) ;
#3273=AXIS2_PLACEMENT_3D ( 'NONE', #3607, #1921, #6791 ) ;
#3274=CARTESIAN_POINT ( 'NONE',  ( -22.64023588676181475, 99.50000000000000000, -10.01165679465830927 ) ) ;
#3275=CARTESIAN_POINT ( 'NONE',  ( -4.959819536546781389E-15, 2.200000000000000178, 27.00000000000000355 ) ) ;
#3282=CARTESIAN_POINT ( 'NONE',  ( -15.34367147589386349, 99.50000000000004263, 16.87599331055909602 ) ) ;
#3283=CARTESIAN_POINT ( 'NONE',  ( -14.76042637754942177, 100.0000000000000000, 16.05242888258284140 ) ) ;
#3285=CARTESIAN_POINT ( 'NONE',  ( -22.35642768247353729, 99.99999999999995737, -10.34293228154892752 ) ) ;
#3288=CARTESIAN_POINT ( 'NONE',  ( -4.959819536546781389E-15, 2.799999997815050268, 27.00000000000000355 ) ) ;
#3289=CARTESIAN_POINT ( 'NONE',  ( 8.829292973371666520, 99.99999999999998579, 19.92220432019063736 ) ) ;
#3290=EDGE_LOOP ( 'NONE', ( #8808, #1408, #3740, #2217 ) ) ;
#3292=CARTESIAN_POINT ( 'NONE',  ( 21.43339342948717885, 100.0000000000000000, -1.392427884615384803 ) ) ;
#3294=FACE_OUTER_BOUND ( 'NONE', #6918, .T. ) ;
#3295=CARTESIAN_POINT ( 'NONE',  ( 27.43301270000000258, 5.199999998907525622, -11.36312591709336139 ) ) ;
#3297=CARTESIAN_POINT ( 'NONE',  ( -15.18657300206754179, 99.50000000000000000, 16.26161032743331347 ) ) ;
#3299=CARTESIAN_POINT ( 'NONE',  ( -21.91899880027261460, 99.50000000000000000, -9.705014769524845875 ) ) ;
#3300=CARTESIAN_POINT ( 'NONE',  ( 3.282077632710153292, 100.0000000000000000, -23.74569985055724786 ) ) ;
#3301=CARTESIAN_POINT ( 'NONE',  ( -22.33111803333905243, 99.99999999999997158, -9.558150950182401573 ) ) ;
#3303=CARTESIAN_POINT ( 'NONE',  ( 3.810791133452845703, 99.50000000000005684, -24.33305202239136733 ) ) ;
#3304=ORIENTED_EDGE ( 'NONE', *, *, #3430, .F. ) ;
#3306=CARTESIAN_POINT ( 'NONE',  ( -27.43301270000000258, 4.649999998907525800, -3.359575119402369376E-15 ) ) ;
#3307=EDGE_CURVE ( 'NONE', #6092, #3729, #3021, .T. ) ;
#3310=CARTESIAN_POINT ( 'NONE',  ( 19.09188309203678813, 4.100000000000000533, -19.09188309203678813 ) ) ;
#3311=CARTESIAN_POINT ( 'NONE',  ( -20.70854316912038229, 100.0000000000000142, -10.95957977981033515 ) ) ;
#3312=DIRECTION ( 'NONE',  ( 0.000000000000000000, 0.000000000000000000, 1.000000000000000000 ) ) ;
#3313=CARTESIAN_POINT ( 'NONE',  ( -21.24310748994415832, 99.49999999999998579, -10.99527971241054658 ) ) ;
#3314=CARTESIAN_POINT ( 'NONE',  ( -20.77412980915959650, 99.99999999999991473, -9.759484723497815040 ) ) ;
#3315=CARTESIAN_POINT ( 'NONE',  ( -11.36312591709337561, 4.799999998907525267, 27.43301269999999548 ) ) ;
#3316=CARTESIAN_POINT ( 'NONE',  ( 3.606694021351891877, 99.50000000000000000, -24.61315535935035115 ) ) ;
#3317=CARTESIAN_POINT ( 'NONE',  ( -21.98271324694694329, 99.50000000000000000, -11.39207625356720222 ) ) ;
#3318=VECTOR ( 'NONE', #2310, 1000.000000000000114 ) ;
#3320=CARTESIAN_POINT ( 'NONE',  ( -16.57687742313193269, 100.0000000000000284, 15.91855687263828756 ) ) ;
#3322=CARTESIAN_POINT ( 'NONE',  ( 11.18376618407357626, 1.450000000000000400, 27.00000000000000000 ) ) ;
#3326=CARTESIAN_POINT ( 'NONE',  ( -21.56977948371741505, 99.99999999999995737, -11.44450812306045329 ) ) ;
#3330=CARTESIAN_POINT ( 'NONE',  ( -19.75840245672548789, 99.50000000000000000, -8.735905494466331689 ) ) ;
#3332=CARTESIAN_POINT ( 'NONE',  ( 8.074269155311188939, 99.50000000000001421, 20.56111086218762551 ) ) ;
#3334=CARTESIAN_POINT ( 'NONE',  ( -4.959819536546781389E-15, 1.199999997815050401, 27.00000000000000355 ) ) ;
#3335=CARTESIAN_POINT ( 'NONE',  ( -27.00000000000000355, 4.400000000000000355, -3.306546357697854128E-15 ) ) ;
#3339=CARTESIAN_POINT ( 'NONE',  ( 7.812290123947159159, 99.99999999999994316, 21.17203503082402349 ) ) ;
#3340=CARTESIAN_POINT ( 'NONE',  ( -20.97746206809550884, 99.50000000000000000, -11.22189255051946688 ) ) ;
#3341=CARTESIAN_POINT ( 'NONE',  ( 27.00000000000000355, 0.6499999978150502455, -11.18376618407356737 ) ) ;
#3344=CARTESIAN_POINT ( 'NONE',  ( -15.62070810370258833, 99.50000000000000000, 16.62245103965875970 ) ) ;
#3345=CARTESIAN_POINT ( 'NONE',  ( 27.43301270000000258, 0.2499999989075252504, 0.000000000000000000 ) ) ;
#3347=ORIENTED_EDGE ( 'NONE', *, *, #1218, .T. ) ;
#3348=ORIENTED_EDGE ( 'NONE', *, *, #5765, .T. ) ;
#3352=CARTESIAN_POINT ( 'NONE',  ( 19.09188309203678102, 3.900000000000000355, 19.09188309203678813 ) ) ;
#3356=CARTESIAN_POINT ( 'NONE',  ( -20.89884294283097432, 99.99999999999998579, -10.47119744953613640 ) ) ;
#3357=EDGE_CURVE ( 'NONE', #1485, #7448, #1303, .T. ) ;
#3358=CARTESIAN_POINT ( 'NONE',  ( 19.09188309203678813, 0.1000000000000000056, -19.09188309203678813 ) ) ;
#3360=CARTESIAN_POINT ( 'NONE',  ( 2.971063225226878046, 99.50000000000000000, -23.91837856253154015 ) ) ;
#3362=CARTESIAN_POINT ( 'NONE',  ( -22.63784607493503387, 99.50000000000001421, -10.71517552924587058 ) ) ;
#3363=CARTESIAN_POINT ( 'NONE',  ( -22.58826642033182353, 99.99999999999998579, -9.883148377786627137 ) ) ;
#3364=CARTESIAN_POINT ( 'NONE',  ( 8.281567445270807681, 100.0000000000000000, 20.15885744430370252 ) ) ;
#3366=VERTEX_POINT ( 'NONE', #8816 ) ;
#3367=ADVANCED_FACE ( 'NONE', ( #76 ), #4851, .T. ) ;
#3369=CARTESIAN_POINT ( 'NONE',  ( 3.717146347979291665, 99.50000000000000000, -21.42716062222556417 ) ) ;
#3370=CARTESIAN_POINT ( 'NONE',  ( 9.666415885916139317, 99.50000000000001421, 19.95264712196244261 ) ) ;
#3374=FACE_OUTER_BOUND ( 'NONE', #2323, .T. ) ;
#3376=LINE ( 'NONE', #6716, #8841 ) ;
#3377=CARTESIAN_POINT ( 'NONE',  ( -22.24883010645271852, 99.99999999999997158, -10.75389422444101939 ) ) ;
#3378=CARTESIAN_POINT ( 'NONE',  ( 3.207968951880266761, 99.99999999999998579, -22.92616835434091627 ) ) ;
#3379=CARTESIAN_POINT ( 'NONE',  ( 3.635130212803377781, 99.50000000000000000, -23.00575896550913768 ) ) ;
#3380=CARTESIAN_POINT ( 'NONE',  ( 8.393217272293057363, 99.99999999999994316, 19.69436072183531650 ) ) ;
#3383=CARTESIAN_POINT ( 'NONE',  ( 27.00000000000000355, 3.799999997815050268, 0.000000000000000000 ) ) ;
#3384=EDGE_CURVE ( 'NONE', #9410, #8654, #2191, .T. ) ;
#3386=AXIS2_PLACEMENT_3D ( 'NONE', #4735, #4838, #4785 ) ;
#3387=CARTESIAN_POINT ( 'NONE',  ( -21.38163724633288965, 99.50000000000005684, -9.681902434707239991 ) ) ;
#3388=CARTESIAN_POINT ( 'NONE',  ( 8.685676809262872666, 99.50000000000000000, 23.43455588346217766 ) ) ;
#3389=EDGE_CURVE ( 'NONE', #647, #7345, #9931, .T. ) ;
#3390=CARTESIAN_POINT ( 'NONE',  ( -21.33175168474226879, 100.0000000000000142, -11.03889704119913162 ) ) ;
#3391=DIRECTION ( 'NONE',  ( -0.9804671828129908340, 0.000000000000000000, 0.1966827481675937628 ) ) ;
#3395=CARTESIAN_POINT ( 'NONE',  ( -14.89508182811745662, 99.49999999999997158, 15.38112983991209326 ) ) ;
#3396=CARTESIAN_POINT ( 'NONE',  ( 21.79306891025641235, 99.50000000000000000, -1.065004006410256387 ) ) ;
#3397=CARTESIAN_POINT ( 'NONE',  ( -27.43301270000000258, 3.799999998907525711, -11.36312591709336317 ) ) ;
#3399=DIRECTION ( 'NONE',  ( 0.000000000000000000, 1.000000000000000000, 0.000000000000000000 ) ) ;
#3400=LINE ( 'NONE', #9593, #4895 ) ;
#3402=EDGE_LOOP ( 'NONE', ( #9393, #9356 ) ) ;
#3403=CARTESIAN_POINT ( 'NONE',  ( -21.49703851962343037, 99.49999999999997158, -9.300281078773625865 ) ) ;
#3404=CARTESIAN_POINT ( 'NONE',  ( -19.39806930854667755, 4.549999998907525267, -19.39806930854668110 ) ) ;
#3405=CARTESIAN_POINT ( 'NONE',  ( 9.526713201929464248, 99.50000000000000000, 20.38668308130821671 ) ) ;
#3406=CARTESIAN_POINT ( 'NONE',  ( -16.25490828497592588, 99.49999999999998579, 14.91257814242970348 ) ) ;
#3407=CARTESIAN_POINT ( 'NONE',  ( -16.33590634957226229, 100.0000000000000000, 16.80570853669505382 ) ) ;
#3408=CARTESIAN_POINT ( 'NONE',  ( 27.00000000000000355, 1.649999999999999911, -11.18376618407356915 ) ) ;
#3409=CARTESIAN_POINT ( 'NONE',  ( 8.515772100368442565, 100.0000000000000000, 20.00046577258137503 ) ) ;
#3410=EDGE_LOOP ( 'NONE', ( #7734, #810, #6127 ) ) ;
#3414=CARTESIAN_POINT ( 'NONE',  ( 0.000000000000000000, 100.0000000000000000, -27.00000000000000355 ) ) ;
#3415=CARTESIAN_POINT ( 'NONE',  ( 3.207057600658871355, 99.50000000000000000, -22.07913334414698880 ) ) ;
#3416=AXIS2_PLACEMENT_3D ( 'NONE', #1302, #679, #5397 ) ;
#3417=CARTESIAN_POINT ( 'NONE',  ( -21.33175168474226879, 99.50000000000001421, -11.03889704119913162 ) ) ;
#3419=EDGE_CURVE ( 'NONE', #4212, #7890, #9010, .T. ) ;
#3420=CIRCLE ( 'NONE', #1091, 7.500000000000000000 ) ;
#3421=LINE ( 'NONE', #6478, #4952 ) ;
#3424=AXIS2_PLACEMENT_3D ( 'NONE', #5871, #2734, #8332 ) ;
#3426=B_SPLINE_CURVE_WITH_KNOTS ( 'NONE', 3,
 ( #1413, #6956, #8591, #2407, #4758, #9627, #1671, #3154, #938, #7956, #5603, #789, #2459, #3981, #10316, #6337, #890, #47, #7167 ),
 .UNSPECIFIED., .F., .F.,
 ( 4, 1, 1, 1, 1, 1, 1, 1, 1, 1, 1, 1, 1, 1, 1, 1, 4 ),
 ( 0.000000000000000000, 0.06455295689170470474, 0.1273249605695649933, 0.1891299628201091876, 0.2499617887110622549, 0.3104215510145779122, 0.3717966107350694216, 0.4346754705585744727, 0.4991966429079077727, 0.5636107885140392293, 0.6264421791528413941, 0.6882713145562978641, 0.7491215306807221808, 0.8100115732567139126, 0.8716292230916812267, 0.9349778748807419104, 1.000000000000000000 ),
 .UNSPECIFIED. ) ;
#3427=DIRECTION ( 'NONE',  ( -0.3368610894541371747, 0.000000000000000000, 0.9415543565890243105 ) ) ;
#3428=CARTESIAN_POINT ( 'NONE',  ( 4.295198626299898237, 99.50000000000001421, -24.68029520312135361 ) ) ;
#3429=CARTESIAN_POINT ( 'NONE',  ( 7.729958523985794194, 99.50000000000001421, 20.63140804260154937 ) ) ;
#3430=EDGE_CURVE ( 'NONE', #2896, #6863, #4348, .T. ) ;
#3431=VERTEX_POINT ( 'NONE', #1782 ) ;
#3432=CARTESIAN_POINT ( 'NONE',  ( 9.838488147574068421, 99.50000000000000000, 20.25735696016189280 ) ) ;
#3433=CARTESIAN_POINT ( 'NONE',  ( -19.09188309203678813, 3.499999997815050445, 19.09188309203678457 ) ) ;
#3435=CARTESIAN_POINT ( 'NONE',  ( -20.71654887124055122, 99.50000000000001421, -9.874326132881018125 ) ) ;
#3436=CARTESIAN_POINT ( 'NONE',  ( -20.96643530928959720, 100.0000000000000142, -10.05541671241505064 ) ) ;
#3438=CARTESIAN_POINT ( 'NONE',  ( -22.28244091826395135, 99.50000000000000000, -10.68852969318427881 ) ) ;
#3439=CARTESIAN_POINT ( 'NONE',  ( 4.871887406949175769, 99.99999999999995737, -23.77896509604281405 ) ) ;
#3447=CARTESIAN_POINT ( 'NONE',  ( 3.058419780146050648, 100.0000000000000000, -23.12871267107006545 ) ) ;
#3448=CARTESIAN_POINT ( 'NONE',  ( -27.43301270000000969, 3.099999998907525089, 11.36312591709335429 ) ) ;
#3450=CARTESIAN_POINT ( 'NONE',  ( 9.676361905416721143, 100.0000000000000142, 21.63547735782115566 ) ) ;
#3452=CARTESIAN_POINT ( 'NONE',  ( -21.16695614262292580, 99.50000000000000000, -11.33496398805607441 ) ) ;
#3454=CYLINDRICAL_SURFACE ( 'NONE', #1793, 27.00000000000000355 ) ;
#3455=CARTESIAN_POINT ( 'NONE',  ( 8.429066232339796017, 100.0000000000000000, 19.67794530653910101 ) ) ;
#3456=ADVANCED_FACE ( 'NONE', ( #4297 ), #5719, .F. ) ;
#3458=CARTESIAN_POINT ( 'NONE',  ( -21.69499712064247277, 99.99999999999992895, -9.295461156691713356 ) ) ;
#3459=CARTESIAN_POINT ( 'NONE',  ( 3.977571997893210032, 100.0000000000000000, -24.70179182097838932 ) ) ;
#3461=CARTESIAN_POINT ( 'NONE',  ( -21.20999280589743918, 99.50000000000002842, -11.35389291771566000 ) ) ;
#3463=CARTESIAN_POINT ( 'NONE',  ( 11.18376618407357626, 1.249999997815050445, 27.00000000000000000 ) ) ;
#3464=CARTESIAN_POINT ( 'NONE',  ( 8.757234875838378230, 99.50000000000000000, 19.92790116963689329 ) ) ;
#3466=CARTESIAN_POINT ( 'NONE',  ( 9.576498344683301411, 99.49999999999998579, 20.78592410672095880 ) ) ;
#3467=DIRECTION ( 'NONE',  ( -0.000000000000000000, -1.000000000000000000, -0.000000000000000000 ) ) ;
#3468=ORIENTED_EDGE ( 'NONE', *, *, #8100, .F. ) ;
#3469=EDGE_CURVE ( 'NONE', #6584, #1392, #4586, .T. ) ;
#3474=LINE ( 'NONE', #281, #122 ) ;
#3475=CARTESIAN_POINT ( 'NONE',  ( -15.07178375341841559, 100.0000000000000142, 15.16157792772069968 ) ) ;
#3476=CARTESIAN_POINT ( 'NONE',  ( 4.295198626299897349, 100.0000000000000284, -24.68029520312135006 ) ) ;
#3477=CARTESIAN_POINT ( 'NONE',  ( -16.60513711880302878, 99.50000000000000000, 15.15667007515659570 ) ) ;
#3478=CARTESIAN_POINT ( 'NONE',  ( 1.653273178848927064E-15, 1.599999997815050312, -27.00000000000000355 ) ) ;
#3480=LINE ( 'NONE', #240, #8974 ) ;
#3481=CARTESIAN_POINT ( 'NONE',  ( 21.47055288461538325, 99.50000000000000000, -0.7081330128205128860 ) ) ;
#3482=EDGE_LOOP ( 'NONE', ( #5224, #3659, #4768, #2811 ) ) ;
#3484=CARTESIAN_POINT ( 'NONE',  ( 27.43301270000000258, 2.749999998907525445, 0.000000000000000000 ) ) ;
#3486=CARTESIAN_POINT ( 'NONE',  ( 4.154273145530666511, 99.99999999999997158, -22.82723029927519676 ) ) ;
#3487=CARTESIAN_POINT ( 'NONE',  ( 7.826802610544922878, 99.99999999999994316, 21.21129867192371421 ) ) ;
#3488=CARTESIAN_POINT ( 'NONE',  ( 9.881472129446523311, 99.50000000000002842, 20.94326683228310060 ) ) ;
#3489=CARTESIAN_POINT ( 'NONE',  ( -27.00000000000001421, 3.449999997815051511, 11.18376618407356382 ) ) ;
#3490=CARTESIAN_POINT ( 'NONE',  ( -21.07003209069497984, 99.49999999999998579, -11.28505157174820361 ) ) ;
#3491=CARTESIAN_POINT ( 'NONE',  ( -21.52330660073277002, 99.50000000000001421, -9.647028226243550719 ) ) ;
#3492=CARTESIAN_POINT ( 'NONE',  ( -22.11394672483139701, 99.50000000000000000, -10.91855052283267646 ) ) ;
#3494=DIRECTION ( 'NONE',  ( -0.000000000000000000, 1.000000000000000000, -0.000000000000000000 ) ) ;
#3496=EDGE_CURVE ( 'NONE', #1490, #7639, #8571, .T. ) ;
#3498=CARTESIAN_POINT ( 'NONE',  ( -14.89910828679519739, 99.99999999999995737, 16.44921749203638939 ) ) ;
#3499=CARTESIAN_POINT ( 'NONE',  ( 2.983739933759421259, 99.49999999999998579, -23.28421226151478152 ) ) ;
#3500=CARTESIAN_POINT ( 'NONE',  ( 27.43301270000000258, 2.649999998907525356, 0.000000000000000000 ) ) ;
#3501=FACE_OUTER_BOUND ( 'NONE', #8346, .T. ) ;
#3502=CARTESIAN_POINT ( 'NONE',  ( -20.63200021313574695, 100.0000000000000000, -10.19493994959453431 ) ) ;
#3503=LINE ( 'NONE', #5909, #7321 ) ;
#3506=CARTESIAN_POINT ( 'NONE',  ( 6.246869686064662197, 99.50000000000000000, 20.92172973853146090 ) ) ;
#3507=CARTESIAN_POINT ( 'NONE',  ( 3.411785164761435674, 100.0000000000000000, -22.76693382491622231 ) ) ;
#3508=CARTESIAN_POINT ( 'NONE',  ( 11.36312591709336850, 4.899999998907527576, 27.43301269999999903 ) ) ;
#3509=CARTESIAN_POINT ( 'NONE',  ( 1.679787559701184688E-15, 0.4499999989075252338, -27.43301270000000258 ) ) ;
#3511=CARTESIAN_POINT ( 'NONE',  ( 4.486604876299897349, 99.50000000000000000, -21.85617661337775885 ) ) ;
#3512=CARTESIAN_POINT ( 'NONE',  ( 4.100286767325537873, 99.50000000000000000, -22.51382885696750336 ) ) ;
#3515=ORIENTED_EDGE ( 'NONE', *, *, #5959, .T. ) ;
#3516=ORIENTED_EDGE ( 'NONE', *, *, #4103, .F. ) ;
#3517=LINE ( 'NONE', #5873, #6712 ) ;
#3519=ORIENTED_EDGE ( 'NONE', *, *, #820, .T. ) ;
#3522=CARTESIAN_POINT ( 'NONE',  ( -22.51488550592518934, 99.99999999999997158, -10.97145172607810615 ) ) ;
#3523=LINE ( 'NONE', #6708, #1276 ) ;
#3525=VECTOR ( 'NONE', #6198, 1000.000000000000227 ) ;
#3526=ORIENTED_EDGE ( 'NONE', *, *, #1028, .F. ) ;
#3530=CARTESIAN_POINT ( 'NONE',  ( 9.897596448871711416, 99.99999999999998579, 20.85734708541456328 ) ) ;
#3532=CARTESIAN_POINT ( 'NONE',  ( 0.000000000000000000, 100.0000000000000000, 0.000000000000000000 ) ) ;
#3533=CARTESIAN_POINT ( 'NONE',  ( 19.39806930854668110, 2.849999998907525089, -19.39806930854668110 ) ) ;
#3534=DIRECTION ( 'NONE',  ( -0.000000000000000000, 1.000000000000000000, -0.000000000000000000 ) ) ;
#3537=CARTESIAN_POINT ( 'NONE',  ( 7.913184448816831029, 99.50000000000000000, 20.09878816755126252 ) ) ;
#3539=CARTESIAN_POINT ( 'NONE',  ( 2.852289972453743161, 99.50000000000000000, -22.14293542748032451 ) ) ;
#3540=CARTESIAN_POINT ( 'NONE',  ( -11.18376618407356560, 4.849999997815050534, -27.00000000000000355 ) ) ;
#3543=FACE_OUTER_BOUND ( 'NONE', #6903, .T. ) ;
#3546=CARTESIAN_POINT ( 'NONE',  ( 2.852289972453743161, 100.0000000000000000, -22.14293542748032451 ) ) ;
#3551=CARTESIAN_POINT ( 'NONE',  ( -14.74935495356232984, 100.0000000000000000, 15.91322402822111926 ) ) ;
#3552=CARTESIAN_POINT ( 'NONE',  ( 5.825495487346713297, 99.50000000000000000, 20.69456627699299744 ) ) ;
#3553=AXIS2_PLACEMENT_3D ( 'NONE', #6783, #8410, #7513 ) ;
#3554=CARTESIAN_POINT ( 'NONE',  ( -19.39806930854667755, 3.749999998907525445, -19.39806930854668110 ) ) ;
#3556=CIRCLE ( 'NONE', #1722, 18.00000000000000000 ) ;
#3559=CARTESIAN_POINT ( 'NONE',  ( 10.72103337977569204, 99.50000000000000000, 22.20268488987243316 ) ) ;
#3560=CARTESIAN_POINT ( 'NONE',  ( 7.726884419709978857, 100.0000000000000000, 20.74516479202295471 ) ) ;
#3562=CARTESIAN_POINT ( 'NONE',  ( 8.393217272293057363, 99.50000000000000000, 19.69436072183531650 ) ) ;
#3565=( BOUNDED_SURFACE ( )  B_SPLINE_SURFACE ( 1, 2, ( 
 ( #7816, #3011, #8711, #4724, #3734, #1430, #2894, #3060, #9327, #7705, #751, #2271, #6133, #541, #2321, #5520, #6078, #2159, #644, #3788, #2102, #7918, #3116, #4567, #3943, #8660, #7128, #6188, #1482, #8493, #5469, #9269, #8549, #6973, #1374, #7866, #5296, #10115, #1322, #3891, #4510, #6243, #593, #2952, #7762, #9443, #10175, #4624, #2214, #696, #7078, #3840, #7025, #10228, #6299, #9497, #3166, #4189, #4046, #2421, #5720, #164, #6544, #3261, #7970, #1686, #804, #6451, #7181, #9590, #2528, #4774, #5567, #5766, #8858, #4968, #4879, #8806, #3352, #6351, #8075, #8024, #3310, #9733, #5670, #8757, #1771, #3997, #8905, #13, #4827, #2368, #904, #2571, #7329, #9641, #4094, #7280, #8954, #65, #8166 ),
 ( #6499, #9544, #5618, #3214, #2475, #1581, #1732, #4923, #118, #8120, #6399, #9688, #855, #1635, #996, #950, #7229, #4144, #10333, #2616, #6589, #4391, #5065, #1974, #5963, #7471, #2718, #5906, #8420, #7576, #1821, #3610, #261, #9939, #4239, #2773, #7420, #313, #414, #212, #7522, #1046, #6638, #9992, #8369, #2665, #9833, #9201, #3500, #6742, #363, #1872, #9780, #5221, #8316, #2828, #5118, #3448, #6686, #4287, #7371, #9879, #6793, #1147, #5811, #9156, #9102, #4338, #6009, #5857, #3554, #3397, #5170, #8267, #9053, #1199, #2026, #9002, #1251, #1095, #1923, #5017, #8213, #7687, #2876, #6060, #3827, #2992, #6899, #7009, #3770, #10212, #9427, #3665, #9251, #2084, #10041, #3046, #5342, #4441, #6226 ) ),
 .UNSPECIFIED., .F., .F., .F. ) 
 B_SPLINE_SURFACE_WITH_KNOTS ( ( 2, 2 ),
 ( 3, 2, 2, 2, 2, 2, 2, 2, 2, 2, 2, 2, 2, 2, 2, 2, 2, 2, 2, 2, 2, 2, 2, 2, 2, 2, 2, 2, 2, 2, 2, 2, 2, 2, 2, 2, 2, 2, 2, 2, 2, 2, 2, 2, 2, 2, 2, 2, 2, 2, 3 ),
 ( 0.000000000000000000, 1.000000000000000000 ),
 ( 0.000000000000000000, 0.01785714285714285615, 0.03571428571428571230, 0.05357142857142856845, 0.07142857142857142461, 0.08928571428571428770, 0.1071428571428571369, 0.1250000000000000000, 0.1428571428571428492, 0.1607142857142857262, 0.1785714285714285754, 0.1964285714285714246, 0.2142857142857142738, 0.2321428571428571508, 0.2500000000000000000, 0.2678571428571428492, 0.2857142857142856984, 0.3035714285714285476, 0.3214285714285714524, 0.3392857142857143016, 0.3571428571428571508, 0.3750000000000000000, 0.3928571428571428492, 0.4107142857142856984, 0.4285714285714285476, 0.4464285714285714524, 0.4642857142857143016, 0.4821428571428571508, 0.5000000000000000000, 0.5178571428571429047, 0.5357142857142856984, 0.5535714285714286031, 0.5714285714285713969, 0.5892857142857143016, 0.6071428571428570953, 0.6250000000000000000, 0.6428571428571429047, 0.6607142857142856984, 0.6785714285714286031, 0.6964285714285713969, 0.7142857142857143016, 0.7321428571428570953, 0.7500000000000000000, 0.7678571428571429047, 0.7857142857142856984, 0.8035714285714286031, 0.8214285714285713969, 0.8392857142857143016, 0.8571428571428570953, 0.8750000000000000000, 0.8928571428571429047 ),
 .UNSPECIFIED. ) 
 GEOMETRIC_REPRESENTATION_ITEM ( )  RATIONAL_B_SPLINE_SURFACE ( (
 ( 1.000000000000000000, 0.9238795325112867385, 1.000000000000000000, 0.9238795325112867385, 1.000000000000000000, 0.9238795325112867385, 1.000000000000000000, 0.9238795325112867385, 1.000000000000000000, 0.9238795325112867385, 1.000000000000000000, 0.9238795325112867385, 1.000000000000000000, 0.9238795325112867385, 1.000000000000000000, 0.9238795325112867385, 1.000000000000000000, 0.9238795325112867385, 1.000000000000000000, 0.9238795325112867385, 1.000000000000000000, 0.9238795325112867385, 1.000000000000000000, 0.9238795325112867385, 1.000000000000000000, 0.9238795325112867385, 1.000000000000000000, 0.9238795325112867385, 1.000000000000000000, 0.9238795325112867385, 1.000000000000000000, 0.9238795325112867385, 1.000000000000000000, 0.9238795325112867385, 1.000000000000000000, 0.9238795325112867385, 1.000000000000000000, 0.9238795325112867385, 1.000000000000000000, 0.9238795325112867385, 1.000000000000000000, 0.9238795325112867385, 1.000000000000000000, 0.9238795325112867385, 1.000000000000000000, 0.9238795325112867385, 1.000000000000000000, 0.9238795325112867385, 1.000000000000000000, 0.9238795325112867385, 1.000000000000000000, 0.9238795325112867385, 1.000000000000000000, 0.9238795325112867385, 1.000000000000000000, 0.9238795325112867385, 1.000000000000000000, 0.9238795325112867385, 1.000000000000000000, 0.9238795325112867385, 1.000000000000000000, 0.9238795325112867385, 1.000000000000000000, 0.9238795325112867385, 1.000000000000000000, 0.9238795325112867385, 1.000000000000000000, 0.9238795325112867385, 1.000000000000000000, 0.9238795325112867385, 1.000000000000000000, 0.9238795325112867385, 1.000000000000000000, 0.9238795325112867385, 1.000000000000000000, 0.9238795325112867385, 1.000000000000000000, 0.9238795325112867385, 1.000000000000000000, 0.9238795325112867385, 1.000000000000000000, 0.9238795325112867385, 1.000000000000000000, 0.9238795325112867385, 1.000000000000000000, 0.9238795325112867385, 1.000000000000000000, 0.9238795325112867385, 1.000000000000000000, 0.9238795325112867385, 1.000000000000000000, 0.9238795325112867385, 1.000000000000000000, 0.9238795325112867385, 1.000000000000000000, 0.9238795325112867385, 1.000000000000000000, 0.9238795325112867385, 1.000000000000000000, 0.9238795325112867385, 1.000000000000000000),
 ( 1.000000000000000000, 0.9238795325112867385, 1.000000000000000000, 0.9238795325112867385, 1.000000000000000000, 0.9238795325112867385, 1.000000000000000000, 0.9238795325112867385, 1.000000000000000000, 0.9238795325112867385, 1.000000000000000000, 0.9238795325112867385, 1.000000000000000000, 0.9238795325112867385, 1.000000000000000000, 0.9238795325112867385, 1.000000000000000000, 0.9238795325112867385, 1.000000000000000000, 0.9238795325112867385, 1.000000000000000000, 0.9238795325112867385, 1.000000000000000000, 0.9238795325112867385, 1.000000000000000000, 0.9238795325112867385, 1.000000000000000000, 0.9238795325112867385, 1.000000000000000000, 0.9238795325112867385, 1.000000000000000000, 0.9238795325112867385, 1.000000000000000000, 0.9238795325112867385, 1.000000000000000000, 0.9238795325112867385, 1.000000000000000000, 0.9238795325112867385, 1.000000000000000000, 0.9238795325112867385, 1.000000000000000000, 0.9238795325112867385, 1.000000000000000000, 0.9238795325112867385, 1.000000000000000000, 0.9238795325112867385, 1.000000000000000000, 0.9238795325112867385, 1.000000000000000000, 0.9238795325112867385, 1.000000000000000000, 0.9238795325112867385, 1.000000000000000000, 0.9238795325112867385, 1.000000000000000000, 0.9238795325112867385, 1.000000000000000000, 0.9238795325112867385, 1.000000000000000000, 0.9238795325112867385, 1.000000000000000000, 0.9238795325112867385, 1.000000000000000000, 0.9238795325112867385, 1.000000000000000000, 0.9238795325112867385, 1.000000000000000000, 0.9238795325112867385, 1.000000000000000000, 0.9238795325112867385, 1.000000000000000000, 0.9238795325112867385, 1.000000000000000000, 0.9238795325112867385, 1.000000000000000000, 0.9238795325112867385, 1.000000000000000000, 0.9238795325112867385, 1.000000000000000000, 0.9238795325112867385, 1.000000000000000000, 0.9238795325112867385, 1.000000000000000000, 0.9238795325112867385, 1.000000000000000000, 0.9238795325112867385, 1.000000000000000000, 0.9238795325112867385, 1.000000000000000000, 0.9238795325112867385, 1.000000000000000000, 0.9238795325112867385, 1.000000000000000000, 0.9238795325112867385, 1.000000000000000000, 0.9238795325112867385, 1.000000000000000000, 0.9238795325112867385, 1.000000000000000000, 0.9238795325112867385, 1.000000000000000000) ) ) 
 REPRESENTATION_ITEM ( '' )  SURFACE ( )  );
#3566=CARTESIAN_POINT ( 'NONE',  ( 9.563602730896748838, 99.50000000000001421, 20.87184380654744587 ) ) ;
#3567=CARTESIAN_POINT ( 'NONE',  ( 3.845216150098881513, 100.0000000000000000, -21.40922359334548020 ) ) ;
#3569=CARTESIAN_POINT ( 'NONE',  ( 11.18376618407357093, 2.550000000000000266, -27.00000000000000355 ) ) ;
#3572=ORIENTED_EDGE ( 'NONE', *, *, #10251, .T. ) ;
#3573=CARTESIAN_POINT ( 'NONE',  ( 4.906732565843439531, 100.0000000000000142, -23.57187248890526376 ) ) ;
#3576=CARTESIAN_POINT ( 'NONE',  ( -22.00707282958688182, 99.49999999999997158, -9.748971510896797810 ) ) ;
#3577=DIRECTION ( 'NONE',  ( -0.9985315370676781654, 0.000000000000000000, 0.05417351272771728926 ) ) ;
#3578=LINE ( 'NONE', #2741, #6260 ) ;
#3579=CARTESIAN_POINT ( 'NONE',  ( 4.331079892889020400, 100.0000000000000284, -24.67336562508343079 ) ) ;
#3582=VECTOR ( 'NONE', #6132, 1000.000000000000000 ) ;
#3583=CARTESIAN_POINT ( 'NONE',  ( -15.13520964245927836, 99.49999999999998579, 15.69931698147095034 ) ) ;
#3585=ORIENTED_EDGE ( 'NONE', *, *, #3638, .T. ) ;
#3586=CARTESIAN_POINT ( 'NONE',  ( 9.184850993605147944E-16, 85.00000000000000000, 7.500000000000000000 ) ) ;
#3588=ORIENTED_EDGE ( 'NONE', *, *, #4727, .T. ) ;
#3589=PLANE ( 'NONE',  #6901 ) ;
#3590=CARTESIAN_POINT ( 'NONE',  ( 11.36312591709336139, 3.699999998907525622, -27.43301270000000258 ) ) ;
#3592=CARTESIAN_POINT ( 'NONE',  ( -16.85368146453285831, 99.99999999999998579, 16.27421966797335529 ) ) ;
#3593=CARTESIAN_POINT ( 'NONE',  ( -4.959819536546781389E-15, 4.399999997815050357, 27.00000000000000355 ) ) ;
#3595=ORIENTED_EDGE ( 'NONE', *, *, #1064, .T. ) ;
#3596=CARTESIAN_POINT ( 'NONE',  ( -19.46743691185369585, 99.50000000000000000, -8.912588186774021537 ) ) ;
#3597=CARTESIAN_POINT ( 'NONE',  ( -19.09188309203678457, 4.099999997815050534, -19.09188309203678813 ) ) ;
#3598=CARTESIAN_POINT ( 'NONE',  ( 24.91446314102564230, 99.50000000000000000, -1.581029647435897578 ) ) ;
#3601=VERTEX_POINT ( 'NONE', #8628 ) ;
#3602=CARTESIAN_POINT ( 'NONE',  ( 4.829054701479813083, 99.50000000000000000, -23.91032069601275367 ) ) ;
#3603=CARTESIAN_POINT ( 'NONE',  ( 19.39806930854667399, 1.849999998907525312, 19.39806930854668465 ) ) ;
#3607=CARTESIAN_POINT ( 'NONE',  ( 0.000000000000000000, 0.000000000000000000, 0.000000000000000000 ) ) ;
#3610=CARTESIAN_POINT ( 'NONE',  ( 27.43301269999999548, 1.799999998907525267, 11.36312591709337738 ) ) ;
#3612=VERTEX_POINT ( 'NONE', #6994 ) ;
#3614=CARTESIAN_POINT ( 'NONE',  ( -15.62070810370258833, 100.0000000000000000, 16.62245103965875970 ) ) ;
#3615=CARTESIAN_POINT ( 'NONE',  ( 4.523042264738025509, 100.0000000000000142, -24.25177047807976294 ) ) ;
#3617=CARTESIAN_POINT ( 'NONE',  ( -18.01369080470046313, 99.50000000000000000, 17.15556831233607937 ) ) ;
#3620=CARTESIAN_POINT ( 'NONE',  ( 4.793167276645844410, 99.99999999999998579, -21.69837440717521204 ) ) ;
#3624=CARTESIAN_POINT ( 'NONE',  ( 27.43301270000000258, 1.049999998907525267, 0.000000000000000000 ) ) ;
#3625=EDGE_CURVE ( 'NONE', #7937, #5423, #6931, .T. ) ;
#3626=CARTESIAN_POINT ( 'NONE',  ( 27.00000000000000355, 4.850000000000000533, -11.18376618407356915 ) ) ;
#3627=CARTESIAN_POINT ( 'NONE',  ( 3.477525819554967423, 99.50000000000000000, -22.44236894434852658 ) ) ;
#3628=VECTOR ( 'NONE', #9569, 1000.000000000000000 ) ;
#3631=AXIS2_PLACEMENT_3D ( 'NONE', #2767, #4233, #5110 ) ;
#3633=ORIENTED_EDGE ( 'NONE', *, *, #3915, .T. ) ;
#3634=CARTESIAN_POINT ( 'NONE',  ( 0.000000000000000000, 100.0000000000000000, 0.000000000000000000 ) ) ;
#3635=CARTESIAN_POINT ( 'NONE',  ( -16.07368679829020763, 100.0000000000000000, 17.11560437002838952 ) ) ;
#3637=EDGE_CURVE ( 'NONE', #1777, #3208, #1178, .T. ) ;
#3638=EDGE_CURVE ( 'NONE', #3821, #2104, #9171, .T. ) ;
#3639=CARTESIAN_POINT ( 'NONE',  ( 4.100286767325537873, 100.0000000000000000, -22.51382885696750336 ) ) ;
#3640=CARTESIAN_POINT ( 'NONE',  ( -19.09188309203678457, 3.299999997815050712, -19.09188309203678813 ) ) ;
#3642=CARTESIAN_POINT ( 'NONE',  ( -27.00000000000000355, 1.200000000000000178, -3.306546357697854128E-15 ) ) ;
#3644=VERTEX_POINT ( 'NONE', #8777 ) ;
#3645=PLANE ( 'NONE',  #10262 ) ;
#3646=CARTESIAN_POINT ( 'NONE',  ( 27.43301270000000258, 3.599999998907525534, -11.36312591709336139 ) ) ;
#3647=CARTESIAN_POINT ( 'NONE',  ( 9.676361905416719367, 99.50000000000000000, 21.63547735782115211 ) ) ;
#3649=CARTESIAN_POINT ( 'NONE',  ( -16.35834224700816009, 99.50000000000000000, 16.43761959438736397 ) ) ;
#3652=CARTESIAN_POINT ( 'NONE',  ( 9.357053078540884528, 99.50000000000001421, 19.70216357796830664 ) ) ;
#3655=CARTESIAN_POINT ( 'NONE',  ( -21.94169572595625795, 100.0000000000000000, -9.715372641902229489 ) ) ;
#3657=CARTESIAN_POINT ( 'NONE',  ( -15.32348647777738826, 99.50000000000000000, 15.39505148541300450 ) ) ;
#3658=CARTESIAN_POINT ( 'NONE',  ( 19.39806930854667399, 1.049999998907525045, 19.39806930854668465 ) ) ;
#3659=ORIENTED_EDGE ( 'NONE', *, *, #2238, .F. ) ;
#3660=ADVANCED_FACE ( 'NONE', ( #6472 ), #4066, .T. ) ;
#3663=CARTESIAN_POINT ( 'NONE',  ( 3.638175769014108774, 99.99999999999995737, -21.10017783766535970 ) ) ;
#3665=CARTESIAN_POINT ( 'NONE',  ( 11.36312591709336850, 4.899999998907526688, 27.43301269999999903 ) ) ;
#3666=CARTESIAN_POINT ( 'NONE',  ( -11.36312591709335962, 2.999999998907524557, -27.43301270000000258 ) ) ;
#3668=B_SPLINE_CURVE_WITH_KNOTS ( 'NONE', 3,
 ( #9687, #1529, #5616, #4723, #4826, #2526, #750, #5718, #1730, #9049, #4187, #8313, #4336, #5063, #1145 ),
 .UNSPECIFIED., .F., .F.,
 ( 4, 1, 1, 1, 1, 1, 1, 1, 1, 1, 1, 1, 4 ),
 ( 0.000000000000000000, 0.08635447908391848115, 0.1695936995346988552, 0.2509241109261274860, 0.3325843554298174576, 0.4138183564518133073, 0.4948404748415979881, 0.5772065644957810049, 0.6619893985813737336, 0.7474108716807353892, 0.8313115314839791825, 0.9147691218156368542, 1.000000000000000000 ),
 .UNSPECIFIED. ) ;
#3669=CARTESIAN_POINT ( 'NONE',  ( -15.42956291708403782, 99.99999999999998579, 16.53061251458192515 ) ) ;
#3670=CARTESIAN_POINT ( 'NONE',  ( 8.132491713109025966, 99.50000000000000000, 21.08089001807756091 ) ) ;
#3672=CARTESIAN_POINT ( 'NONE',  ( -4.959819536546781389E-15, 4.599999999999999645, 27.00000000000000355 ) ) ;
#3674=CARTESIAN_POINT ( 'NONE',  ( 3.373335371007685435, 100.0000000000000000, -22.75111425220066863 ) ) ;
#3675=PLANE ( 'NONE',  #9643 ) ;
#3676=CARTESIAN_POINT ( 'NONE',  ( 19.39806930854667399, 2.549999998907525267, 19.39806930854668465 ) ) ;
#3677=CARTESIAN_POINT ( 'NONE',  ( -15.42740294075255925, 99.99999999999995737, 14.91894146668702348 ) ) ;
#3678=CARTESIAN_POINT ( 'NONE',  ( 9.563602730896748838, 99.50000000000001421, 20.87184380654744587 ) ) ;
#3679=FACE_OUTER_BOUND ( 'NONE', #5231, .T. ) ;
#3681=EDGE_CURVE ( 'NONE', #2280, #653, #3233, .T. ) ;
#3684=ORIENTED_EDGE ( 'NONE', *, *, #5244, .T. ) ;
#3686=CARTESIAN_POINT ( 'NONE',  ( -15.24337324910153946, 99.99999999999997158, 16.81353386054630761 ) ) ;
#3687=CARTESIAN_POINT ( 'NONE',  ( -21.18972881998075763, 99.49999999999998579, -9.781869222470191971 ) ) ;
#3689=CARTESIAN_POINT ( 'NONE',  ( 3.817429849879703241, 99.49999999999998579, -22.92346308580664171 ) ) ;
#3690=CARTESIAN_POINT ( 'NONE',  ( -11.18376618407358336, 3.750000000000000444, 26.99999999999999645 ) ) ;
#3691=B_SPLINE_CURVE_WITH_KNOTS ( 'NONE', 3,
 ( #8749, #8944, #8850, #4916, #1676, #8798, #845, #5710, #1573, #6387, #4818, #1625, #8113, #1762, #988, #7218, #4084, #1724, #9580 ),
 .UNSPECIFIED., .F., .F.,
 ( 4, 1, 1, 1, 1, 1, 1, 1, 1, 1, 1, 1, 1, 1, 1, 1, 4 ),
 ( 0.000000000000000000, 0.05935611633690887623, 0.1167563879513689451, 0.1743885027374874330, 0.2308223543163396840, 0.2888100779544915953, 0.3475404098195560842, 0.4086537266250744316, 0.4723446836969566465, 0.5362968130936018873, 0.6000923674009760456, 0.6637702377379335328, 0.7274568328636339398, 0.7924602533659969028, 0.8590386936388050287, 0.9283644560612371865, 1.000000000000000000 ),
 .UNSPECIFIED. ) ;
#3692=EDGE_LOOP ( 'NONE', ( #5573, #207, #7888, #9692 ) ) ;
#3693=EDGE_CURVE ( 'NONE', #7819, #4830, #2593, .T. ) ;
#3696=CARTESIAN_POINT ( 'NONE',  ( 26.99999999999999645, 0.7499999999999998890, 11.18376618407358691 ) ) ;
#3697=ORIENTED_EDGE ( 'NONE', *, *, #5586, .T. ) ;
#3699=CARTESIAN_POINT ( 'NONE',  ( 11.36312591709336139, 2.899999998907526244, -27.43301270000000258 ) ) ;
#3701=CARTESIAN_POINT ( 'NONE',  ( 9.902568905804752575, 99.99999999999997158, 20.48863403721516363 ) ) ;
#3702=LINE ( 'NONE', #2919, #6595 ) ;
#3703=LINE ( 'NONE', #565, #2213 ) ;
#3706=EDGE_LOOP ( 'NONE', ( #217, #9083, #327, #10236 ) ) ;
#3707=DIRECTION ( 'NONE',  ( 0.9197781680807419757, 0.000000000000000000, -0.3924386850477849520 ) ) ;
#3708=CARTESIAN_POINT ( 'NONE',  ( -5.039362679103552881E-15, 1.749999998907525223, 27.43301270000000258 ) ) ;
#3714=CARTESIAN_POINT ( 'NONE',  ( 3.106448761625311139, 99.99999999999995737, -21.38062202216113761 ) ) ;
#3717=CARTESIAN_POINT ( 'NONE',  ( -16.92301558088953328, 99.50000000000001421, 15.88693424423437683 ) ) ;
#3718=CARTESIAN_POINT ( 'NONE',  ( -19.39806930854668465, 0.8499999989075252005, 19.39806930854667755 ) ) ;
#3719=ORIENTED_EDGE ( 'NONE', *, *, #4168, .F. ) ;
#3721=EDGE_CURVE ( 'NONE', #3778, #8324, #5691, .T. ) ;
#3722=CARTESIAN_POINT ( 'NONE',  ( -16.34021191015031249, 100.0000000000000000, 16.45483272884350967 ) ) ;
#3723=FACE_OUTER_BOUND ( 'NONE', #5826, .T. ) ;
#3725=DIRECTION ( 'NONE',  ( 0.1714283378204774499, 0.000000000000000000, -0.9851965920526259968 ) ) ;
#3726=EDGE_LOOP ( 'NONE', ( #9226, #8690, #6107, #1682 ) ) ;
#3729=VERTEX_POINT ( 'NONE', #9708 ) ;
#3731=CARTESIAN_POINT ( 'NONE',  ( 1.679787559701184688E-15, 1.249999998907525223, -27.43301270000000258 ) ) ;
#3734=CARTESIAN_POINT ( 'NONE',  ( 1.653273178848927064E-15, 0.2000000000000000111, -27.00000000000000355 ) ) ;
#3735=CARTESIAN_POINT ( 'NONE',  ( 8.684839681857363658, 100.0000000000000426, 19.94043386883836178 ) ) ;
#3737=FACE_OUTER_BOUND ( 'NONE', #8066, .T. ) ;
#3738=AXIS2_PLACEMENT_3D ( 'NONE', #5791, #8888, #1025 ) ;
#3740=ORIENTED_EDGE ( 'NONE', *, *, #6262, .T. ) ;
#3742=CARTESIAN_POINT ( 'NONE',  ( 19.39806930854668110, 0.3499999989075252560, -19.39806930854668110 ) ) ;
#3743=CARTESIAN_POINT ( 'NONE',  ( -21.52330660073277002, 99.50000000000001421, -9.647028226243550719 ) ) ;
#3745=CARTESIAN_POINT ( 'NONE',  ( 2.983739933759421259, 99.99999999999998579, -23.28421226151478152 ) ) ;
#3746=CARTESIAN_POINT ( 'NONE',  ( 4.633286773149219329, 99.50000000000002842, -21.44575434969419447 ) ) ;
#3747=CARTESIAN_POINT ( 'NONE',  ( -16.76168403648438243, 100.0000000000000284, 16.44483764528499847 ) ) ;
#3749=EDGE_LOOP ( 'NONE', ( #2945, #3976, #5575, #7415 ) ) ;
#3750=DIRECTION ( 'NONE',  ( 0.05468478504300072762, 0.000000000000000000, 0.9985036676371302766 ) ) ;
#3753=EDGE_CURVE ( 'NONE', #10122, #1438, #2796, .T. ) ;
#3754=CARTESIAN_POINT ( 'NONE',  ( 9.766630880609509902, 99.50000000000002842, 21.37293705761699059 ) ) ;
#3755=B_SPLINE_SURFACE_WITH_KNOTS ( 'NONE', 3, 1, ( 
 ( #5930, #3476 ),
 ( #9856, #3579 ),
 ( #6819, #6662 ),
 ( #438, #2594 ),
 ( #9128, #1946 ),
 ( #8978, #1797 ),
 ( #7394, #2228 ),
 ( #5250, #5482 ),
 ( #4691, #8562 ),
 ( #10241, #2849 ),
 ( #7715, #3025 ),
 ( #9457, #2906 ),
 ( #5430, #497 ),
 ( #2056, #1387 ),
 ( #7039, #6146 ),
 ( #1495, #4522 ),
 ( #6201, #2113 ),
 ( #8505, #2283 ),
 ( #6033, #9399 ) ),
 .UNSPECIFIED., .F., .F., .F.,
 ( 4, 1, 1, 1, 1, 1, 1, 1, 1, 1, 1, 1, 1, 1, 1, 1, 4 ),
 ( 2, 2 ),
 ( 0.000000000000000000, 0.06533929434940796699, 0.1284421010879715219, 0.1894557237235162950, 0.2487158350925330053, 0.3070727012892665031, 0.3650088636856013702, 0.4229902474982629723, 0.4815891416229265420, 0.5404453987529589387, 0.6002338948610608238, 0.6608164219703346332, 0.7232441343194829786, 0.7881366429682739039, 0.8556965829275263724, 0.9259544997225339635, 1.000000000000000000 ),
 ( 0.000000000000000000, 1.000000000000000000 ),
 .UNSPECIFIED. ) ;
#3757=CARTESIAN_POINT ( 'NONE',  ( -22.08823018108446234, 100.0000000000000000, -9.406177930363766038 ) ) ;
#3758=CARTESIAN_POINT ( 'NONE',  ( 8.429066232339796017, 99.50000000000000000, 19.67794530653910101 ) ) ;
#3760=DIRECTION ( 'NONE',  ( 0.000000000000000000, 1.000000000000000000, 0.000000000000000000 ) ) ;
#3764=VERTEX_POINT ( 'NONE', #8393 ) ;
#3767=CARTESIAN_POINT ( 'NONE',  ( 27.21650635000000307, 0.4749999983612877563, 0.000000000000000000 ) ) ;
#3768=CARTESIAN_POINT ( 'NONE',  ( 2.843562173796539749, 99.50000000000001421, -21.91597968833000110 ) ) ;
#3770=CARTESIAN_POINT ( 'NONE',  ( -19.39806930854668465, 4.749999998907525445, 19.39806930854667755 ) ) ;
#3771=CARTESIAN_POINT ( 'NONE',  ( 1.679787559701184688E-15, 1.349999998907525312, -27.43301270000000258 ) ) ;
#3772=VERTEX_POINT ( 'NONE', #5983 ) ;
#3773=CARTESIAN_POINT ( 'NONE',  ( -15.49014769301379069, 99.99999999999997158, 16.56834637662448273 ) ) ;
#3774=FACE_OUTER_BOUND ( 'NONE', #5033, .T. ) ;
#3776=VECTOR ( 'NONE', #9104, 999.9999999999998863 ) ;
#3777=CARTESIAN_POINT ( 'NONE',  ( -16.05932294508833280, 100.0000000000000000, 15.21084698918278555 ) ) ;
#3778=VERTEX_POINT ( 'NONE', #2691 ) ;
#3780=CARTESIAN_POINT ( 'NONE',  ( 4.280752963211088336, 99.49999999999997158, -21.16602454745684270 ) ) ;
#3784=CARTESIAN_POINT ( 'NONE',  ( 19.39806930854667399, 3.349999998907525534, 19.39806930854668465 ) ) ;
#3786=EDGE_CURVE ( 'NONE', #2600, #3916, #1067, .T. ) ;
#3788=CARTESIAN_POINT ( 'NONE',  ( 11.18376618407356915, 0.9499999999999999556, -27.00000000000000355 ) ) ;
#3789=FACE_OUTER_BOUND ( 'NONE', #7110, .T. ) ;
#3792=CARTESIAN_POINT ( 'NONE',  ( -16.57330815294036697, 99.99999999999997158, 15.84440382193293217 ) ) ;
#3793=CARTESIAN_POINT ( 'NONE',  ( 8.117007248954752896, 99.50000000000001421, 20.40979824468519155 ) ) ;
#3794=ORIENTED_EDGE ( 'NONE', *, *, #2370, .T. ) ;
#3797=ORIENTED_EDGE ( 'NONE', *, *, #4110, .F. ) ;
#3798=CARTESIAN_POINT ( 'NONE',  ( 11.36312591709336850, 0.8999999989075253559, 27.43301269999999903 ) ) ;
#3803=CARTESIAN_POINT ( 'NONE',  ( 0.000000000000000000, 85.00000000000000000, -7.500000000000000000 ) ) ;
#3804=DIRECTION ( 'NONE',  ( 0.05376826219280737146, 0.000000000000000000, 0.9985534407235125975 ) ) ;
#3806=ORIENTED_EDGE ( 'NONE', *, *, #4909, .T. ) ;
#3815=CARTESIAN_POINT ( 'NONE',  ( 8.429066232339796017, 100.0000000000000000, 19.67794530653910101 ) ) ;
#3818=ORIENTED_EDGE ( 'NONE', *, *, #3693, .T. ) ;
#3819=FACE_OUTER_BOUND ( 'NONE', #6950, .T. ) ;
#3820=CARTESIAN_POINT ( 'NONE',  ( 27.43301270000000258, 0.3499999989075252005, 0.000000000000000000 ) ) ;
#3821=VERTEX_POINT ( 'NONE', #3475 ) ;
#3825=CARTESIAN_POINT ( 'NONE',  ( 3.203979444200292015, 99.50000000000000000, -21.29640115293693725 ) ) ;
#3827=CARTESIAN_POINT ( 'NONE',  ( -19.39806930854667755, 4.549999998907525267, -19.39806930854668110 ) ) ;
#3828=CARTESIAN_POINT ( 'NONE',  ( -11.36312591709335962, 2.199999998907525622, -27.43301270000000258 ) ) ;
#3829=CARTESIAN_POINT ( 'NONE',  ( 8.751508028230254865, 99.99999999999998579, 19.58480916780017722 ) ) ;
#3830=CARTESIAN_POINT ( 'NONE',  ( 4.143207896384923039, 99.49999999999998579, -24.36264353342416911 ) ) ;
#3831=CARTESIAN_POINT ( 'NONE',  ( 3.283294465904739390, 99.50000000000002842, -21.71066637097430885 ) ) ;
#3835=CARTESIAN_POINT ( 'NONE',  ( -21.94169572595625795, 99.50000000000000000, -9.715372641902229489 ) ) ;
#3837=CARTESIAN_POINT ( 'NONE',  ( 19.39806930854668110, 3.549999998907525267, -19.39806930854668110 ) ) ;
#3839=CARTESIAN_POINT ( 'NONE',  ( -15.29853103387017121, 99.50000000000001421, 14.98378122532347057 ) ) ;
#3840=CARTESIAN_POINT ( 'NONE',  ( 11.18376618407356915, 2.549999999999999822, -27.00000000000000355 ) ) ;
#3841=CARTESIAN_POINT ( 'NONE',  ( 9.404665101723468368, 100.0000000000000284, 20.17141824467128686 ) ) ;
#3842=ORIENTED_EDGE ( 'NONE', *, *, #6044, .T. ) ;
#3843=CARTESIAN_POINT ( 'NONE',  ( -27.00000000000000355, 2.799999999999999822, -3.306546357697854128E-15 ) ) ;
#3844=FACE_OUTER_BOUND ( 'NONE', #6700, .T. ) ;
#3847=ORIENTED_EDGE ( 'NONE', *, *, #3384, .T. ) ;
#3848=CARTESIAN_POINT ( 'NONE',  ( 19.39806930854668110, 3.549999998907525267, -19.39806930854668110 ) ) ;
#3850=CARTESIAN_POINT ( 'NONE',  ( -15.31787750341841559, 99.50000000000001421, 16.43551622900274722 ) ) ;
#3852=( BOUNDED_CURVE ( )  B_SPLINE_CURVE ( 2, ( #3820, #7570, #7621, #2133, #5271, #9301, #462, #7736, #3041, #6221, #2985, #9420, #7680, #4598, #3658, #7002, #622, #8469, #10206, #518, #5446, #9364, #9986, #6109, #5391, #8639, #6053, #4384, #3708, #408, #3603, #569, #8585, #6892, #6839, #8414, #10033, #2871, #6786, #10089, #2821, #6003, #9243, #9196, #6166, #2017, #5214, #2925, #1245, #2077, #5334, #4435, #1296, #8526, #1350, #6278, #7055, #7256, #10364, #6480, #3194, #4655, #39, #2348, #4705, #9570, #1612, #6330, #6375, #7846, #5547, #7897, #2403, #731, #10263, #3094, #833, #5597, #3923, #3242, #9474, #9524, #8738, #8001, #7109, #4807, #10309, #4026, #8689, #3144, #676, #2303, #2507, #6429, #1562, #7207, #4753, #5498, #9621, #5699, #1511 ),
 .UNSPECIFIED., .F., .F. ) 
 B_SPLINE_CURVE_WITH_KNOTS ( ( 3, 2, 2, 2, 2, 2, 2, 2, 2, 2, 2, 2, 2, 2, 2, 2, 2, 2, 2, 2, 2, 2, 2, 2, 2, 2, 2, 2, 2, 2, 2, 2, 2, 2, 2, 2, 2, 2, 2, 2, 2, 2, 2, 2, 2, 2, 2, 2, 2, 2, 3 ),
 ( 0.000000000000000000, 0.01785714285714285615, 0.03571428571428571230, 0.05357142857142856845, 0.07142857142857142461, 0.08928571428571428770, 0.1071428571428571369, 0.1250000000000000000, 0.1428571428571428492, 0.1607142857142857262, 0.1785714285714285754, 0.1964285714285714246, 0.2142857142857142738, 0.2321428571428571508, 0.2500000000000000000, 0.2678571428571428492, 0.2857142857142856984, 0.3035714285714285476, 0.3214285714285714524, 0.3392857142857143016, 0.3571428571428571508, 0.3750000000000000000, 0.3928571428571428492, 0.4107142857142856984, 0.4285714285714285476, 0.4464285714285714524, 0.4642857142857143016, 0.4821428571428571508, 0.5000000000000000000, 0.5178571428571429047, 0.5357142857142856984, 0.5535714285714286031, 0.5714285714285713969, 0.5892857142857143016, 0.6071428571428570953, 0.6250000000000000000, 0.6428571428571429047, 0.6607142857142856984, 0.6785714285714286031, 0.6964285714285715079, 0.7142857142857143016, 0.7321428571428570953, 0.7500000000000000000, 0.7678571428571429047, 0.7857142857142856984, 0.8035714285714286031, 0.8214285714285713969, 0.8392857142857143016, 0.8571428571428570953, 0.8750000000000000000, 0.8928571428571429047 ),
 .UNSPECIFIED. ) 
 CURVE ( )  GEOMETRIC_REPRESENTATION_ITEM ( )  RATIONAL_B_SPLINE_CURVE ( ( 1.000000000000000000, 0.9238795325112867385, 1.000000000000000000, 0.9238795325112867385, 1.000000000000000000, 0.9238795325112867385, 1.000000000000000000, 0.9238795325112867385, 1.000000000000000000, 0.9238795325112867385, 1.000000000000000000, 0.9238795325112867385, 1.000000000000000000, 0.9238795325112867385, 1.000000000000000000, 0.9238795325112867385, 1.000000000000000000, 0.9238795325112867385, 1.000000000000000000, 0.9238795325112867385, 1.000000000000000000, 0.9238795325112867385, 1.000000000000000000, 0.9238795325112867385, 1.000000000000000000, 0.9238795325112867385, 1.000000000000000000, 0.9238795325112867385, 1.000000000000000000, 0.9238795325112867385, 1.000000000000000000, 0.9238795325112867385, 1.000000000000000000, 0.9238795325112867385, 1.000000000000000000, 0.9238795325112867385, 1.000000000000000000, 0.9238795325112867385, 1.000000000000000000, 0.9238795325112867385, 1.000000000000000000, 0.9238795325112867385, 1.000000000000000000, 0.9238795325112867385, 1.000000000000000000, 0.9238795325112867385, 1.000000000000000000, 0.9238795325112867385, 1.000000000000000000, 0.9238795325112867385, 1.000000000000000000, 0.9238795325112867385, 1.000000000000000000, 0.9238795325112867385, 1.000000000000000000, 0.9238795325112867385, 1.000000000000000000, 0.9238795325112867385, 1.000000000000000000, 0.9238795325112867385, 1.000000000000000000, 0.9238795325112867385, 1.000000000000000000, 0.9238795325112867385, 1.000000000000000000, 0.9238795325112867385, 1.000000000000000000, 0.9238795325112867385, 1.000000000000000000, 0.9238795325112867385, 1.000000000000000000, 0.9238795325112867385, 1.000000000000000000, 0.9238795325112867385, 1.000000000000000000, 0.9238795325112867385, 1.000000000000000000, 0.9238795325112867385, 1.000000000000000000, 0.9238795325112867385, 1.000000000000000000, 0.9238795325112867385, 1.000000000000000000, 0.9238795325112867385, 1.000000000000000000, 0.9238795325112867385, 1.000000000000000000, 0.9238795325112867385, 1.000000000000000000, 0.9238795325112867385, 1.000000000000000000, 0.9238795325112867385, 1.000000000000000000, 0.9238795325112867385, 1.000000000000000000, 0.9238795325112867385, 1.000000000000000000, 0.9238795325112867385, 1.000000000000000000, 0.9238795325112867385, 1.000000000000000000 ) ) 
 REPRESENTATION_ITEM ( '' )  );
#3856=CARTESIAN_POINT ( 'NONE',  ( 4.504418077186241653, 100.0000000000000426, -21.31258943653750393 ) ) ;
#3857=FACE_OUTER_BOUND ( 'NONE', #6081, .T. ) ;
#3858=ORIENTED_EDGE ( 'NONE', *, *, #1949, .T. ) ;
#3859=CARTESIAN_POINT ( 'NONE',  ( 8.536201443755420115, 99.50000000000002842, 19.63502355897212581 ) ) ;
#3861=EDGE_LOOP ( 'NONE', ( #5742, #783, #9448, #1942 ) ) ;
#3866=CARTESIAN_POINT ( 'NONE',  ( -22.12191435419165941, 99.50000000000001421, -9.834338183724410598 ) ) ;
#3867=ORIENTED_EDGE ( 'NONE', *, *, #428, .T. ) ;
#3868=CARTESIAN_POINT ( 'NONE',  ( -15.34161522349497808, 99.99999999999998579, 15.37783959465231121 ) ) ;
#3869=CARTESIAN_POINT ( 'NONE',  ( 8.757234875838378230, 100.0000000000000000, 19.92790116963689329 ) ) ;
#3870=EDGE_LOOP ( 'NONE', ( #136, #5921, #330, #9703 ) ) ;
#3874=CARTESIAN_POINT ( 'NONE',  ( 4.909381318607588973, 99.50000000000000000, -23.54377677363417121 ) ) ;
#3875=CARTESIAN_POINT ( 'NONE',  ( 19.39806930854668110, 1.249999998907525223, -19.39806930854668110 ) ) ;
#3876=CARTESIAN_POINT ( 'NONE',  ( -15.32348647777738826, 99.99999999999997158, 15.39505148541300450 ) ) ;
#3878=CARTESIAN_POINT ( 'NONE',  ( 3.810791133452845703, 99.50000000000005684, -24.33305202239136733 ) ) ;
#3879=CARTESIAN_POINT ( 'NONE',  ( -19.46743691185369585, 100.0000000000000000, -8.912588186774021537 ) ) ;
#3880=CARTESIAN_POINT ( 'NONE',  ( 21.43339342948717885, 99.50000000000000000, -1.392427884615384803 ) ) ;
#3882=CARTESIAN_POINT ( 'NONE',  ( 3.739209042966563867, 100.0000000000000000, -21.42288334414699236 ) ) ;
#3886=CARTESIAN_POINT ( 'NONE',  ( 1.679787559701184688E-15, 4.449999998907525622, -27.43301270000000258 ) ) ;
#3888=CARTESIAN_POINT ( 'NONE',  ( -15.42740294075255925, 99.50000000000000000, 14.91894146668702348 ) ) ;
#3889=VECTOR ( 'NONE', #1869, 1000.000000000000000 ) ;
#3890=EDGE_CURVE ( 'NONE', #10071, #3238, #4360, .T. ) ;
#3891=CARTESIAN_POINT ( 'NONE',  ( -27.00000000000000355, 1.950000000000000400, -11.18376618407357093 ) ) ;
#3894=CARTESIAN_POINT ( 'NONE',  ( -16.56356094049941419, 99.99999999999994316, 15.77213757552179629 ) ) ;
#3895=CARTESIAN_POINT ( 'NONE',  ( -15.62070810370258833, 100.0000000000000000, 16.62245103965875970 ) ) ;
#3899=CARTESIAN_POINT ( 'NONE',  ( 19.39806930854667399, 2.549999998907525267, 19.39806930854668465 ) ) ;
#3900=CARTESIAN_POINT ( 'NONE',  ( -21.91899880027261460, 99.50000000000000000, -9.705014769524845875 ) ) ;
#3902=CARTESIAN_POINT ( 'NONE',  ( 2.928963527206765338, 99.99999999999997158, -23.52685633767685758 ) ) ;
#3903=EDGE_CURVE ( 'NONE', #2398, #827, #10035, .T. ) ;
#3904=ORIENTED_EDGE ( 'NONE', *, *, #8426, .F. ) ;
#3905=CARTESIAN_POINT ( 'NONE',  ( 4.405197143102897783, 99.49999999999995737, -21.72932741277565682 ) ) ;
#3906=AXIS2_PLACEMENT_3D ( 'NONE', #3532, #8347, #4318 ) ;
#3909=ORIENTED_EDGE ( 'NONE', *, *, #2818, .F. ) ;
#3910=CARTESIAN_POINT ( 'NONE',  ( 4.457146071884139360, 100.0000000000000284, -24.28472590373185724 ) ) ;
#3911=CARTESIAN_POINT ( 'NONE',  ( -15.58193289918752278, 99.50000000000000000, 16.98546238400348329 ) ) ;
#3912=EDGE_CURVE ( 'NONE', #3208, #6241, #3578, .T. ) ;
#3915=EDGE_CURVE ( 'NONE', #4694, #7282, #5312, .T. ) ;
#3916=VERTEX_POINT ( 'NONE', #3639 ) ;
#3917=CARTESIAN_POINT ( 'NONE',  ( -22.21584973381871464, 100.0000000000000142, -9.938501092090024969 ) ) ;
#3918=CARTESIAN_POINT ( 'NONE',  ( 9.666415885916139317, 100.0000000000000142, 19.95264712196244261 ) ) ;
#3921=ORIENTED_EDGE ( 'NONE', *, *, #6836, .T. ) ;
#3922=CARTESIAN_POINT ( 'NONE',  ( -14.75894607058735630, 99.50000000000002842, 15.77473972644577849 ) ) ;
#3923=CARTESIAN_POINT ( 'NONE',  ( 19.39806930854667399, 4.249999998907525445, 19.39806930854668465 ) ) ;
#3929=DIRECTION ( 'NONE',  ( 0.000000000000000000, 1.000000000000000000, 0.000000000000000000 ) ) ;
#3930=CARTESIAN_POINT ( 'NONE',  ( -19.39806930854668465, 4.849999998907525978, 19.39806930854667755 ) ) ;
#3931=LINE ( 'NONE', #8698, #1917 ) ;
#3932=VECTOR ( 'NONE', #3058, 1000.000000000000000 ) ;
#3933=CARTESIAN_POINT ( 'NONE',  ( 3.735769352376668184, 99.49999999999998579, -24.30643046864489420 ) ) ;
#3935=B_SPLINE_SURFACE_WITH_KNOTS ( 'NONE', 3, 1, ( 
 ( #2780, #7585 ),
 ( #4505, #423 ),
 ( #7698, #3620 ),
 ( #8602, #9436 ),
 ( #2363, #5463 ),
 ( #5514, #6181 ),
 ( #2314, #1425 ),
 ( #7807, #10222 ),
 ( #5409, #9379 ),
 ( #9491, #5611 ),
 ( #3780, #9539 ),
 ( #8653, #3938 ),
 ( #6292, #2207 ),
 ( #4613, #3161 ),
 ( #1475, #3005 ),
 ( #6344, #3207 ),
 ( #2264, #4670 ),
 ( #10276, #7861 ),
 ( #5560, #6967 ) ),
 .UNSPECIFIED., .F., .F., .F.,
 ( 4, 1, 1, 1, 1, 1, 1, 1, 1, 1, 1, 1, 1, 1, 1, 1, 4 ),
 ( 2, 2 ),
 ( 0.000000000000000000, 0.07315862907712983310, 0.1430989967074559055, 0.2105333571262071879, 0.2759142635903734653, 0.3397077151413689933, 0.4013946392018796772, 0.4627937533375801049, 0.5237250720276656057, 0.5836284080752294212, 0.6425725562371763511, 0.7010486867616194662, 0.7591976973140022178, 0.8177727706511607186, 0.8769111530050104353, 0.9375229829315941954, 1.000000000000000000 ),
 ( 0.000000000000000000, 1.000000000000000000 ),
 .UNSPECIFIED. ) ;
#3936=CARTESIAN_POINT ( 'NONE',  ( -16.07368679829020763, 100.0000000000000000, 17.11560437002838952 ) ) ;
#3938=CARTESIAN_POINT ( 'NONE',  ( 4.200543313440712190, 100.0000000000000000, -21.13206004899810608 ) ) ;
#3939=VERTEX_POINT ( 'NONE', #6818 ) ;
#3941=CARTESIAN_POINT ( 'NONE',  ( 11.36312591709336850, 4.099999998907525089, 27.43301269999999903 ) ) ;
#3943=CARTESIAN_POINT ( 'NONE',  ( -27.00000000000000355, 1.200000000000000178, -3.306546357697854128E-15 ) ) ;
#3944=CARTESIAN_POINT ( 'NONE',  ( 3.411785164761435674, 100.0000000000000000, -22.76693382491622231 ) ) ;
#3947=LINE ( 'NONE', #2530, #6641 ) ;
#3948=CARTESIAN_POINT ( 'NONE',  ( 8.122452352567329115, 99.50000000000000000, 21.04970292111833530 ) ) ;
#3952=B_SPLINE_CURVE_WITH_KNOTS ( 'NONE', 3,
 ( #9431, #10161, #9203, #7632, #3829, #6175, #6013, #9315, #1418, #472, #4553, #1360, #2882, #6796, #3048, #6119, #7013, #2937, #1254 ),
 .UNSPECIFIED., .F., .F.,
 ( 4, 1, 1, 1, 1, 1, 1, 1, 1, 1, 1, 1, 1, 1, 1, 1, 4 ),
 ( 0.000000000000000000, 0.07024023345195122559, 0.1375772235014411093, 0.2026681864156774648, 0.2655894380381068620, 0.3279415367477454546, 0.3896445486312665740, 0.4521557380645868096, 0.5154465764363311830, 0.5785479733725392704, 0.6397241484143471046, 0.6996998702489094502, 0.7590513234224176564, 0.8180896689983322423, 0.8773873076253557723, 0.9378402036119877216, 1.000000000000000000 ),
 .UNSPECIFIED. ) ;
#3953=CARTESIAN_POINT ( 'NONE',  ( -19.39806930854667755, 2.949999998907525178, -19.39806930854668110 ) ) ;
#3955=CARTESIAN_POINT ( 'NONE',  ( -22.57971655928959365, 99.50000000000000000, -10.84768434062017839 ) ) ;
#3958=CARTESIAN_POINT ( 'NONE',  ( -16.76168403648438243, 99.50000000000002842, 16.44483764528499847 ) ) ;
#3959=CARTESIAN_POINT ( 'NONE',  ( 27.00000000000000355, 4.649999997815049468, -11.18376618407356915 ) ) ;
#3961=EDGE_CURVE ( 'NONE', #8911, #3601, #5295, .T. ) ;
#3963=CARTESIAN_POINT ( 'NONE',  ( 4.523042264738025509, 100.0000000000000284, -24.25177047807976294 ) ) ;
#3967=ORIENTED_EDGE ( 'NONE', *, *, #1977, .F. ) ;
#3968=ORIENTED_EDGE ( 'NONE', *, *, #7539, .F. ) ;
#3969=CARTESIAN_POINT ( 'NONE',  ( -22.33391032228853490, 100.0000000000000284, -10.55243757774135993 ) ) ;
#3970=AXIS2_PLACEMENT_3D ( 'NONE', #1664, #1561, #6374 ) ;
#3973=CARTESIAN_POINT ( 'NONE',  ( -22.25406130147340633, 99.50000000000002842, -9.998337329044998611 ) ) ;
#3974=CARTESIAN_POINT ( 'NONE',  ( 11.18376618407357626, 2.849999997815050978, 27.00000000000000000 ) ) ;
#3975=CARTESIAN_POINT ( 'NONE',  ( 9.502908418173033667, 100.0000000000000000, 20.32929868008965002 ) ) ;
#3976=ORIENTED_EDGE ( 'NONE', *, *, #1064, .F. ) ;
#3979=CARTESIAN_POINT ( 'NONE',  ( 3.207057600658871355, 100.0000000000000000, -22.07913334414698880 ) ) ;
#3981=CARTESIAN_POINT ( 'NONE',  ( -21.07742585509981126, 99.49999999999998579, -10.85999754779651383 ) ) ;
#3982=CARTESIAN_POINT ( 'NONE',  ( -19.39806930854667755, 4.649999998907525800, -19.39806930854668110 ) ) ;
#3983=CARTESIAN_POINT ( 'NONE',  ( -20.63666786535793207, 99.99999999999998579, -10.16306733409737717 ) ) ;
#3986=CARTESIAN_POINT ( 'NONE',  ( -15.98323291606820362, 99.49999999999998579, 16.64087298452848884 ) ) ;
#3988=CARTESIAN_POINT ( 'NONE',  ( 4.835062408351179286, 100.0000000000000000, -21.79588013901878440 ) ) ;
#3991=CARTESIAN_POINT ( 'NONE',  ( -22.05573893622344173, 99.50000000000000000, -9.391591294897233766 ) ) ;
#3992=ORIENTED_EDGE ( 'NONE', *, *, #7468, .F. ) ;
#3994=CARTESIAN_POINT ( 'NONE',  ( 19.39806930854668110, 4.349999998907525089, -19.39806930854668110 ) ) ;
#3997=CARTESIAN_POINT ( 'NONE',  ( -27.00000000000000355, 4.350000000000000533, -11.18376618407357093 ) ) ;
#3999=CARTESIAN_POINT ( 'NONE',  ( 3.298672054714395063, 99.50000000000001421, -22.72039518595936869 ) ) ;
#4001=CARTESIAN_POINT ( 'NONE',  ( 8.117007248954752896, 100.0000000000000142, 20.40979824468519155 ) ) ;
#4002=VERTEX_POINT ( 'NONE', #6652 ) ;
#4005=CARTESIAN_POINT ( 'NONE',  ( -5.039362679103552881E-15, 4.049999998907525267, 27.43301270000000258 ) ) ;
#4006=CARTESIAN_POINT ( 'NONE',  ( 4.241330131419338123, 99.49999999999998579, -24.68798891778770965 ) ) ;
#4007=CARTESIAN_POINT ( 'NONE',  ( -27.00000000000000355, 0.9999999978150503344, -3.306546357697854128E-15 ) ) ;
#4009=LINE ( 'NONE', #5682, #3228 ) ;
#4010=CARTESIAN_POINT ( 'NONE',  ( -16.62994343074595349, 99.49999999999998579, 15.18287566599475191 ) ) ;
#4012=ORIENTED_EDGE ( 'NONE', *, *, #8191, .F. ) ;
#4014=CARTESIAN_POINT ( 'NONE',  ( 4.793167276645844410, 99.99999999999998579, -21.69837440717521204 ) ) ;
#4016=CARTESIAN_POINT ( 'NONE',  ( -16.35834224700816009, 99.50000000000000000, 16.43761959438736397 ) ) ;
#4017=CARTESIAN_POINT ( 'NONE',  ( -15.07178375341841559, 100.0000000000000142, 15.16157792772069968 ) ) ;
#4019=EDGE_CURVE ( 'NONE', #8640, #6767, #6384, .T. ) ;
#4020=B_SPLINE_SURFACE_WITH_KNOTS ( 'NONE', 3, 1, ( 
 ( #861, #5901 ),
 ( #2766, #252 ),
 ( #4383, #5956 ),
 ( #9149, #7569 ),
 ( #4834, #3439 ),
 ( #1966, #406 ),
 ( #3602, #9985 ),
 ( #9825, #6785 ),
 ( #6631, #2820 ),
 ( #2660, #3265 ),
 ( #7233, #8812 ) ),
 .UNSPECIFIED., .F., .F., .F.,
 ( 4, 1, 1, 1, 1, 1, 1, 1, 4 ),
 ( 2, 2 ),
 ( 0.000000000000000000, 0.1514666391271576040, 0.2940212016997327260, 0.4289076436562640482, 0.5568069201790899481, 0.6759213874835566793, 0.7888117551744765477, 0.8972989960681465593, 1.000000000000000000 ),
 ( 0.000000000000000000, 1.000000000000000000 ),
 .UNSPECIFIED. ) ;
#4021=ORIENTED_EDGE ( 'NONE', *, *, #2423, .F. ) ;
#4023=CARTESIAN_POINT ( 'NONE',  ( 0.000000000000000000, 97.50000000000000000, 0.000000000000000000 ) ) ;
#4024=CARTESIAN_POINT ( 'NONE',  ( -16.40919047799676989, 99.50000000000000000, 16.38364531277195013 ) ) ;
#4026=CARTESIAN_POINT ( 'NONE',  ( -27.43301270000000258, 4.699999998907525622, -11.36312591709336317 ) ) ;
#4028=CARTESIAN_POINT ( 'NONE',  ( 3.375079225685456041, 99.50000000000000000, -22.79123997459842954 ) ) ;
#4029=CARTESIAN_POINT ( 'NONE',  ( 4.100286767325537873, 100.0000000000000000, -22.51382885696750336 ) ) ;
#4031=CARTESIAN_POINT ( 'NONE',  ( -20.88772068548257366, 99.50000000000001421, -11.14739719174079546 ) ) ;
#4032=CARTESIAN_POINT ( 'NONE',  ( 27.43301270000000258, 5.149999998907525800, 0.000000000000000000 ) ) ;
#4034=CARTESIAN_POINT ( 'NONE',  ( -15.22320097062094568, 99.99999999999998579, 16.32303119091969634 ) ) ;
#4035=DIRECTION ( 'NONE',  ( 0.000000000000000000, 1.000000000000000000, 0.000000000000000000 ) ) ;
#4036=CARTESIAN_POINT ( 'NONE',  ( -16.24524625128438515, 99.50000000000002842, 16.53274063862002308 ) ) ;
#4037=CARTESIAN_POINT ( 'NONE',  ( -22.67573144110267336, 100.0000000000000142, -10.14737752305977381 ) ) ;
#4039=CARTESIAN_POINT ( 'NONE',  ( 9.723125805078051798, 100.0000000000000000, 21.50134635983626907 ) ) ;
#4040=VERTEX_POINT ( 'NONE', #1105 ) ;
#4042=CARTESIAN_POINT ( 'NONE',  ( 19.39806930854667399, 4.949999998907525622, 19.39806930854668465 ) ) ;
#4043=EDGE_CURVE ( 'NONE', #9118, #4569, #4298, .T. ) ;
#4046=CARTESIAN_POINT ( 'NONE',  ( -19.09188309203678813, 2.900000000000000355, 19.09188309203678457 ) ) ;
#4048=ORIENTED_EDGE ( 'NONE', *, *, #8265, .T. ) ;
#4050=DIRECTION ( 'NONE',  ( -0.000000000000000000, 1.000000000000000000, -0.000000000000000000 ) ) ;
#4053=CARTESIAN_POINT ( 'NONE',  ( -27.43301270000000258, 1.399999998907525134, -11.36312591709336317 ) ) ;
#4054=CARTESIAN_POINT ( 'NONE',  ( -4.959819536546781389E-15, 2.200000000000000178, 27.00000000000000355 ) ) ;
#4056=CARTESIAN_POINT ( 'NONE',  ( -22.33589105551819642, 99.50000000000002842, -11.18147695539509812 ) ) ;
#4058=CARTESIAN_POINT ( 'NONE',  ( -16.52157078939288937, 99.99999999999998579, 16.20087177393598665 ) ) ;
#4059=FACE_OUTER_BOUND ( 'NONE', #41, .T. ) ;
#4063=CARTESIAN_POINT ( 'NONE',  ( 4.723706824522782455, 99.50000000000000000, -24.08630974238606370 ) ) ;
#4064=CARTESIAN_POINT ( 'NONE',  ( -15.89341924297059094, 99.50000000000001421, 17.07725933521297890 ) ) ;
#4065=SHAPE_REPRESENTATION ( 'Reservoir Tank', ( #5055 ), #8584 ) ;
#4066=PLANE ( 'NONE',  #1538 ) ;
#4069=CARTESIAN_POINT ( 'NONE',  ( -22.34945848979098670, 100.0000000000000284, -10.27225542379191481 ) ) ;
#4072=CARTESIAN_POINT ( 'NONE',  ( -21.94169572595625795, 99.50000000000000000, -9.715372641902229489 ) ) ;
#4073=CARTESIAN_POINT ( 'NONE',  ( -11.18376618407356737, 2.449999997815050623, -27.00000000000000355 ) ) ;
#4074=CARTESIAN_POINT ( 'NONE',  ( 9.304660012616079001, 100.0000000000000000, 20.07619068507570859 ) ) ;
#4075=VERTEX_POINT ( 'NONE', #2783 ) ;
#4076=ADVANCED_FACE ( 'NONE', ( #221 ), #3107, .T. ) ;
#4077=DIRECTION ( 'NONE',  ( 0.000000000000000000, 1.000000000000000000, 0.000000000000000000 ) ) ;
#4078=CARTESIAN_POINT ( 'NONE',  ( -21.03403678956047074, 100.0000000000000142, -10.80451401317004922 ) ) ;
#4080=CARTESIAN_POINT ( 'NONE',  ( -20.61566945723384592, 100.0000000000000000, -10.83949095114527594 ) ) ;
#4081=CARTESIAN_POINT ( 'NONE',  ( 27.43301269999999548, 4.299999998907526155, 11.36312591709337738 ) ) ;
#4082=CARTESIAN_POINT ( 'NONE',  ( -15.13293277027690209, 99.50000000000000000, 16.13104881108577970 ) ) ;
#4083=CARTESIAN_POINT ( 'NONE',  ( 27.00000000000000355, 3.849999997815050534, -11.18376618407356915 ) ) ;
#4084=CARTESIAN_POINT ( 'NONE',  ( 3.673732336774000018, 100.0000000000000000, -21.43557726391590279 ) ) ;
#4085=CARTESIAN_POINT ( 'NONE',  ( -22.69331084068295112, 99.99999999999998579, -10.43328931840349050 ) ) ;
#4087=CARTESIAN_POINT ( 'NONE',  ( 9.873655262861264603, 100.0000000000000000, 20.34710108723753308 ) ) ;
#4088=EDGE_CURVE ( 'NONE', #669, #776, #9384, .T. ) ;
#4091=CARTESIAN_POINT ( 'NONE',  ( -11.36312591709337383, 0.8999999989075252449, 27.43301269999999548 ) ) ;
#4093=LINE ( 'NONE', #3165, #4417 ) ;
#4094=CARTESIAN_POINT ( 'NONE',  ( 27.00000000000000355, 4.800000000000000711, 0.000000000000000000 ) ) ;
#4099=CARTESIAN_POINT ( 'NONE',  ( 1.653273178848927064E-15, 0.2000000000000000111, -27.00000000000000355 ) ) ;
#4100=ORIENTED_EDGE ( 'NONE', *, *, #5883, .T. ) ;
#4102=CARTESIAN_POINT ( 'NONE',  ( 11.18376618407357093, 0.1500000000000000222, -27.00000000000000355 ) ) ;
#4103=EDGE_CURVE ( 'NONE', #10097, #9021, #5294, .T. ) ;
#4104=LINE ( 'NONE', #2727, #6614 ) ;
#4105=CARTESIAN_POINT ( 'NONE',  ( 3.472565890032746960, 100.0000000000000284, -24.54662015932514052 ) ) ;
#4106=B_SPLINE_SURFACE_WITH_KNOTS ( 'NONE', 3, 1, ( 
 ( #5900, #4182 ),
 ( #2711, #3390 ),
 ( #945, #9772 ),
 ( #6537, #304 ),
 ( #1814, #6581 ),
 ( #4138, #8258 ),
 ( #5006, #1088 ),
 ( #251, #7363 ),
 ( #5757, #5848 ),
 ( #1137, #7463 ),
 ( #5802, #9096 ),
 ( #8945, #1914 ),
 ( #5108, #2611 ),
 ( #3492, #9726 ),
 ( #6678, #4330 ),
 ( #7514, #8994 ),
 ( #8899, #9043 ),
 ( #8205, #1763 ),
 ( #3438, #6630 ) ),
 .UNSPECIFIED., .F., .F., .F.,
 ( 4, 1, 1, 1, 1, 1, 1, 1, 1, 1, 1, 1, 1, 1, 1, 1, 4 ),
 ( 2, 2 ),
 ( 0.000000000000000000, 0.06463354665699841406, 0.1274839167070160040, 0.1893660780973640267, 0.2502738481868047038, 0.3108090901939400408, 0.3728692346228669741, 0.4358265942208103261, 0.5002515515682643965, 0.5647461136436963125, 0.6273730017603231790, 0.6892793264321037672, 0.7497280364991398827, 0.8111249352628771003, 0.8723480300361200479, 0.9354359082354426480, 1.000000000000000000 ),
 ( 0.000000000000000000, 1.000000000000000000 ),
 .UNSPECIFIED. ) ;
#4108=CARTESIAN_POINT ( 'NONE',  ( -4.959819536546781389E-15, 1.999999997815050445, 27.00000000000000355 ) ) ;
#4109=AXIS2_PLACEMENT_3D ( 'NONE', #5261, #5533, #1288 ) ;
#4110=EDGE_CURVE ( 'NONE', #7728, #6767, #1048, .T. ) ;
#4111=CARTESIAN_POINT ( 'NONE',  ( -22.51767453479306980, 99.50000000000000000, -9.764155749770198511 ) ) ;
#4112=CARTESIAN_POINT ( 'NONE',  ( 5.047889085735837611, 100.0000000000000142, -24.22022158424849536 ) ) ;
#4114=ORIENTED_EDGE ( 'NONE', *, *, #9672, .T. ) ;
#4116=DIRECTION ( 'NONE',  ( -0.000000000000000000, -1.000000000000000000, -0.000000000000000000 ) ) ;
#4117=CARTESIAN_POINT ( 'NONE',  ( -15.45548338988150938, 99.49999999999997158, 16.93306818456458984 ) ) ;
#4118=CARTESIAN_POINT ( 'NONE',  ( -21.79668695291220715, 99.50000000000000000, -11.08213026643738353 ) ) ;
#4119=AXIS2_PLACEMENT_3D ( 'NONE', #2633, #3467, #4353 ) ;
#4122=CARTESIAN_POINT ( 'NONE',  ( 8.063732359723156051, 99.50000000000001421, 20.72384750152746236 ) ) ;
#4125=CARTESIAN_POINT ( 'NONE',  ( -16.25072943800822500, 100.0000000000000568, 15.30228603765648820 ) ) ;
#4126=CARTESIAN_POINT ( 'NONE',  ( -11.18376618407356737, 4.250000000000000888, -27.00000000000000355 ) ) ;
#4127=ORIENTED_EDGE ( 'NONE', *, *, #4973, .F. ) ;
#4128=CARTESIAN_POINT ( 'NONE',  ( 3.775125937424839151, 99.50000000000000000, -21.41825520325024712 ) ) ;
#4130=CARTESIAN_POINT ( 'NONE',  ( 8.322475189980043098, 99.50000000000001421, 19.72675386960232657 ) ) ;
#4133=CARTESIAN_POINT ( 'NONE',  ( -27.00000000000000355, 0.9499999978150502900, -11.18376618407357093 ) ) ;
#4134=CARTESIAN_POINT ( 'NONE',  ( 11.18376618407357626, 3.050000000000000711, 27.00000000000000000 ) ) ;
#4135=CLOSED_SHELL ( 'NONE', ( #6324, #7183, #5741, #8759, #1412, #1144, #2232, #3130, #10322, #2690, #2509, #9951, #1279, #6814, #5751, #4544, #8126, #6776, #9178, #7328, #1083, #194, #4517, #9581, #6704, #7343, #9828, #10040, #2602, #12, #746, #1678, #4854, #9757, #10300, #1389, #5977, #5354, #4933, #1221, #6884, #5949, #2091, #7940, #5327, #4534, #74, #2504, #142, #10110, #4808, #8055, #4865, #4076, #4478, #9245, #5502, #6523, #8070, #5858, #2592, #5790, #6773, #3660, #5928, #58, #4883, #10356, #5216, #6407, #7166, #8706, #683, #2627, #761, #8318, #8901, #4657, #1319, #9988, #1729, #3367, #1901, #389, #7935, #8514, #7040, #4712, #3222, #5241, #9484, #655, #7048, #10242, #491, #7932, #8104, #4861, #6620, #9016, #4580, #1148, #8192, #3456, #5016, #1599 ) ) ;
#4136=CARTESIAN_POINT ( 'NONE',  ( -16.63177974700816009, 100.0000000000000000, 16.59747536361813403 ) ) ;
#4137=CARTESIAN_POINT ( 'NONE',  ( -15.69015368034045643, 99.50000000000001421, 16.64011368054243434 ) ) ;
#4138=CARTESIAN_POINT ( 'NONE',  ( -21.58460863908062066, 99.50000000000002842, -11.10356610083683648 ) ) ;
#4143=CARTESIAN_POINT ( 'NONE',  ( -15.89341924297059094, 99.50000000000001421, 17.07725933521297890 ) ) ;
#4144=CARTESIAN_POINT ( 'NONE',  ( 27.43301270000000258, 1.099999998907525089, -11.36312591709336139 ) ) ;
#4145=ORIENTED_EDGE ( 'NONE', *, *, #9018, .T. ) ;
#4146=EDGE_CURVE ( 'NONE', #2404, #9406, #483, .T. ) ;
#4147=DIRECTION ( 'NONE',  ( -0.000000000000000000, -1.000000000000000000, -0.000000000000000000 ) ) ;
#4150=ORIENTED_EDGE ( 'NONE', *, *, #5314, .F. ) ;
#4151=ORIENTED_EDGE ( 'NONE', *, *, #5083, .T. ) ;
#4152=CARTESIAN_POINT ( 'NONE',  ( 27.43301270000000258, 4.299999998907525267, -11.36312591709336139 ) ) ;
#4153=CARTESIAN_POINT ( 'NONE',  ( 3.606694021351891877, 100.0000000000000000, -24.61315535935035115 ) ) ;
#4154=DIRECTION ( 'NONE',  ( 0.000000000000000000, 0.000000000000000000, 1.000000000000000000 ) ) ;
#4155=CIRCLE ( 'NONE', #8833, 25.15000000000000213 ) ;
#4157=CARTESIAN_POINT ( 'NONE',  ( -22.67341330918043951, 99.50000000000000000, -10.57563951594260665 ) ) ;
#4158=CARTESIAN_POINT ( 'NONE',  ( -16.62994343074595349, 99.99999999999998579, 15.18287566599475191 ) ) ;
#4162=FACE_OUTER_BOUND ( 'NONE', #10001, .T. ) ;
#4163=CARTESIAN_POINT ( 'NONE',  ( 3.204253864046738176, 99.99999999999997158, -22.06071064728738662 ) ) ;
#4164=CARTESIAN_POINT ( 'NONE',  ( -21.51485068221570174, 99.50000000000000000, -11.09552232883975087 ) ) ;
#4166=EDGE_CURVE ( 'NONE', #2986, #405, #7646, .T. ) ;
#4168=EDGE_CURVE ( 'NONE', #653, #8788, #10174, .T. ) ;
#4170=DIRECTION ( 'NONE',  ( -0.000000000000000000, 1.000000000000000000, -0.000000000000000000 ) ) ;
#4171=LINE ( 'NONE', #5744, #3167 ) ;
#4174=CARTESIAN_POINT ( 'NONE',  ( 3.504547665631520648, 99.49999999999997158, -23.10026541809159184 ) ) ;
#4175=CARTESIAN_POINT ( 'NONE',  ( -20.72805389903318130, 100.0000000000000000, -9.848585782927868237 ) ) ;
#4176=CARTESIAN_POINT ( 'NONE',  ( 9.873655262861264603, 99.50000000000000000, 20.34710108723753308 ) ) ;
#4177=CARTESIAN_POINT ( 'NONE',  ( 19.09188309203678102, 3.699999997815051067, 19.09188309203678813 ) ) ;
#4179=CARTESIAN_POINT ( 'NONE',  ( -20.79740905086423552, 99.50000000000001421, -11.06234285579171051 ) ) ;
#4182=CARTESIAN_POINT ( 'NONE',  ( -21.30928386698190025, 100.0000000000000000, -11.02857376369709996 ) ) ;
#4183=AXIS2_PLACEMENT_3D ( 'NONE', #4430, #4378, #4594 ) ;
#4187=CARTESIAN_POINT ( 'NONE',  ( -15.42740294075255925, 99.50000000000000000, 14.91894146668702348 ) ) ;
#4189=CARTESIAN_POINT ( 'NONE',  ( -27.00000000000001421, 2.850000000000000089, 11.18376618407356382 ) ) ;
#4190=CARTESIAN_POINT ( 'NONE',  ( 19.39806930854668110, 0.4499999989075251783, -19.39806930854668110 ) ) ;
#4191=DIRECTION ( 'NONE',  ( -0.000000000000000000, -1.000000000000000000, -0.000000000000000000 ) ) ;
#4193=CARTESIAN_POINT ( 'NONE',  ( -20.96129225301843135, 99.50000000000001421, -10.68089388303413934 ) ) ;
#4195=CARTESIAN_POINT ( 'NONE',  ( -21.69499712064247277, 99.49999999999998579, -9.295461156691713356 ) ) ;
#4197=CARTESIAN_POINT ( 'NONE',  ( 19.39806930854668110, 0.3499999989075252005, -19.39806930854668110 ) ) ;
#4199=CARTESIAN_POINT ( 'NONE',  ( 4.405197143102897783, 99.99999999999995737, -21.72932741277565682 ) ) ;
#4200=LINE ( 'NONE', #3767, #547 ) ;
#4201=CARTESIAN_POINT ( 'NONE',  ( -16.67860655220511035, 99.99999999999998579, 15.23428378554110374 ) ) ;
#4202=CARTESIAN_POINT ( 'NONE',  ( 4.295198626299898237, 100.0000000000000142, -24.68029520312135361 ) ) ;
#4203=ORIENTED_EDGE ( 'NONE', *, *, #2251, .F. ) ;
#4205=ORIENTED_EDGE ( 'NONE', *, *, #4220, .T. ) ;
#4207=CARTESIAN_POINT ( 'NONE',  ( 3.861186820804014097, 100.0000000000000426, -21.07288982789904708 ) ) ;
#4208=CARTESIAN_POINT ( 'NONE',  ( 3.231466532446834350, 99.99999999999994316, -21.81145066552309686 ) ) ;
#4210=CARTESIAN_POINT ( 'NONE',  ( 9.806436918512124734, 99.49999999999998579, 20.18080982695387604 ) ) ;
#4212=VERTEX_POINT ( 'NONE', #3010 ) ;
#4213=AXIS2_PLACEMENT_3D ( 'NONE', #6703, #8334, #4410 ) ;
#4220=EDGE_CURVE ( 'NONE', #6813, #872, #643, .T. ) ;
#4221=CARTESIAN_POINT ( 'NONE',  ( 0.000000000000000000, 97.50000000000000000, 0.000000000000000000 ) ) ;
#4222=CARTESIAN_POINT ( 'NONE',  ( 3.171774962637509798, 99.50000000000000000, -24.28498992023182268 ) ) ;
#4223=CARTESIAN_POINT ( 'NONE',  ( 8.223467485077383898, 99.99999999999992895, 19.78581333328655134 ) ) ;
#4226=CARTESIAN_POINT ( 'NONE',  ( 2.964854786877021642, 99.50000000000000000, -22.43901021186594846 ) ) ;
#4227=CARTESIAN_POINT ( 'NONE',  ( -19.09188309203678457, 3.299999997815050712, -19.09188309203678813 ) ) ;
#4229=CARTESIAN_POINT ( 'NONE',  ( -20.97771390646102319, 100.0000000000000284, -10.03345247102482674 ) ) ;
#4231=CARTESIAN_POINT ( 'NONE',  ( 9.342627931057743140, 99.50000000000000000, 21.59831790269294771 ) ) ;
#4232=CARTESIAN_POINT ( 'NONE',  ( 3.106448761625311139, 99.99999999999998579, -21.38062202216113761 ) ) ;
#4233=DIRECTION ( 'NONE',  ( 0.000000000000000000, 1.000000000000000000, 0.000000000000000000 ) ) ;
#4237=CARTESIAN_POINT ( 'NONE',  ( -14.76042637754942177, 99.99999999999998579, 16.05242888258284140 ) ) ;
#4239=CARTESIAN_POINT ( 'NONE',  ( 19.39806930854668110, 1.949999998907525178, -19.39806930854668110 ) ) ;
#4240=CARTESIAN_POINT ( 'NONE',  ( 3.306546357697854128E-15, 0.000000000000000000, 27.00000000000000355 ) ) ;
#4242=CARTESIAN_POINT ( 'NONE',  ( 7.486453019397995234, 99.50000000000000000, 23.81666162955709964 ) ) ;
#4243=CARTESIAN_POINT ( 'NONE',  ( 7.809833820264425519, 99.99999999999995737, 20.29999375863051370 ) ) ;
#4244=VERTEX_POINT ( 'NONE', #7278 ) ;
#4245=CARTESIAN_POINT ( 'NONE',  ( 7.913184448816831029, 99.50000000000000000, 20.09878816755126252 ) ) ;
#4246=CARTESIAN_POINT ( 'NONE',  ( 4.295198626299898237, 100.0000000000000142, -24.68029520312135361 ) ) ;
#4247=CARTESIAN_POINT ( 'NONE',  ( 3.306546357697854128E-15, 100.0000000000000000, 27.00000000000000355 ) ) ;
#4248=CARTESIAN_POINT ( 'NONE',  ( -16.12311789350856017, 99.99999999999995737, 14.86696503675854686 ) ) ;
#4250=DIRECTION ( 'NONE',  ( 0.000000000000000000, 0.000000000000000000, -1.000000000000000000 ) ) ;
#4251=CARTESIAN_POINT ( 'NONE',  ( -22.57971655928959365, 99.50000000000000000, -10.84768434062017839 ) ) ;
#4252=CARTESIAN_POINT ( 'NONE',  ( -21.73488407773357167, 100.0000000000000000, -9.647150398373231184 ) ) ;
#4253=ORIENTED_EDGE ( 'NONE', *, *, #8937, .F. ) ;
#4254=EDGE_CURVE ( 'NONE', #5320, #7728, #7662, .T. ) ;
#4257=CARTESIAN_POINT ( 'NONE',  ( -22.22752541189434794, 99.99999999999994316, -11.26717589342885084 ) ) ;
#4258=CARTESIAN_POINT ( 'NONE',  ( 3.254133136943549776, 99.50000000000000000, -21.76036676155726823 ) ) ;
#4260=CARTESIAN_POINT ( 'NONE',  ( 3.275092494823534928, 99.50000000000000000, -23.54688978826290580 ) ) ;
#4261=CARTESIAN_POINT ( 'NONE',  ( -27.00000000000000355, 3.349999997815050534, -11.18376618407357270 ) ) ;
#4265=DIRECTION ( 'NONE',  ( -0.000000000000000000, -1.000000000000000000, -0.000000000000000000 ) ) ;
#4266=CARTESIAN_POINT ( 'NONE',  ( -21.72555844818415594, 100.0000000000000142, -11.09629251537910655 ) ) ;
#4268=CARTESIAN_POINT ( 'NONE',  ( 4.054941747578200584, 99.49999999999998579, -24.36678493958047298 ) ) ;
#4269=ORIENTED_EDGE ( 'NONE', *, *, #2251, .T. ) ;
#4271=CARTESIAN_POINT ( 'NONE',  ( -27.43301270000000258, 4.699999998907525622, -11.36312591709336317 ) ) ;
#4273=CARTESIAN_POINT ( 'NONE',  ( 3.573144549190039321, 99.99999999999995737, -23.04580706645134214 ) ) ;
#4274=CARTESIAN_POINT ( 'NONE',  ( 8.322475189980043098, 99.99999999999995737, 19.72675386960232657 ) ) ;
#4275=ORIENTED_EDGE ( 'NONE', *, *, #2074, .F. ) ;
#4276=CARTESIAN_POINT ( 'NONE',  ( -20.72805389903318130, 100.0000000000000000, -9.848585782927868237 ) ) ;
#4277=CARTESIAN_POINT ( 'NONE',  ( 11.18376618407356915, 3.149999997815050801, -27.00000000000000355 ) ) ;
#4280=DIRECTION ( 'NONE',  ( 0.2907756355032780071, 0.000000000000000000, 0.9567912676219745283 ) ) ;
#4282=ORIENTED_EDGE ( 'NONE', *, *, #1843, .T. ) ;
#4283=AXIS2_PLACEMENT_3D ( 'NONE', #5865, #912, #9741 ) ;
#4285=CARTESIAN_POINT ( 'NONE',  ( -14.75894607058735630, 100.0000000000000142, 15.77473972644577849 ) ) ;
#4287=CARTESIAN_POINT ( 'NONE',  ( -11.36312591709337383, 3.199999998907524734, 27.43301269999999548 ) ) ;
#4289=VECTOR ( 'NONE', #4489, 1000.000000000000000 ) ;
#4290=EDGE_CURVE ( 'NONE', #2960, #6092, #8044, .T. ) ;
#4291=CARTESIAN_POINT ( 'NONE',  ( 0.000000000000000000, 100.0000000000000000, 0.000000000000000000 ) ) ;
#4292=VECTOR ( 'NONE', #7248, 1000.000000000000000 ) ;
#4293=CARTESIAN_POINT ( 'NONE',  ( 4.457146071884139360, 100.0000000000000142, -24.28472590373185724 ) ) ;
#4295=CARTESIAN_POINT ( 'NONE',  ( -20.89052720883767122, 99.99999999999994316, -9.602653601535816819 ) ) ;
#4296=CARTESIAN_POINT ( 'NONE',  ( -5.039362679103552881E-15, 4.849999998907525089, 27.43301270000000258 ) ) ;
#4297=FACE_OUTER_BOUND ( 'NONE', #5570, .T. ) ;
#4298=LINE ( 'NONE', #1057, #2257 ) ;
#4299=CARTESIAN_POINT ( 'NONE',  ( -16.42071764973191250, 100.0000000000000142, 16.76105279315999042 ) ) ;
#4300=CARTESIAN_POINT ( 'NONE',  ( 9.389534246205572643, 99.99999999999994316, 21.46805835725047729 ) ) ;
#4302=VERTEX_POINT ( 'NONE', #6498 ) ;
#4303=CARTESIAN_POINT ( 'NONE',  ( -15.83671465916681242, 99.50000000000000000, 16.65403364262263608 ) ) ;
#4305=EDGE_LOOP ( 'NONE', ( #3992, #7378, #6064, #4487 ) ) ;
#4306=AXIS2_PLACEMENT_3D ( 'NONE', #9783, #3399, #4971 ) ;
#4307=DIRECTION ( 'NONE',  ( -0.000000000000000000, 1.000000000000000000, -0.000000000000000000 ) ) ;
#4308=CARTESIAN_POINT ( 'NONE',  ( 3.317038232150706367, 99.49999999999998579, -21.66195598387956878 ) ) ;
#4309=CARTESIAN_POINT ( 'NONE',  ( 3.282077632710153292, 99.50000000000000000, -23.74569985055724786 ) ) ;
#4312=ORIENTED_EDGE ( 'NONE', *, *, #5630, .F. ) ;
#4313=CARTESIAN_POINT ( 'NONE',  ( -16.52157078939288937, 99.99999999999994316, 16.20087177393598665 ) ) ;
#4315=DIRECTION ( 'NONE',  ( 0.9853569121566161382, 0.000000000000000000, 0.1705044153832351028 ) ) ;
#4317=ORIENTED_EDGE ( 'NONE', *, *, #8937, .T. ) ;
#4318=DIRECTION ( 'NONE',  ( 1.000000000000000000, 0.000000000000000000, 0.000000000000000000 ) ) ;
#4319=CARTESIAN_POINT ( 'NONE',  ( -27.43301270000000258, 2.349999998907525534, -3.359575119402369376E-15 ) ) ;
#4320=CARTESIAN_POINT ( 'NONE',  ( 3.079986699855593473E-15, 0.000000000000000000, 25.15000000000000213 ) ) ;
#4322=CARTESIAN_POINT ( 'NONE',  ( 3.891852272358404807, 99.50000000000001421, -22.89765557720719968 ) ) ;
#4323=CARTESIAN_POINT ( 'NONE',  ( 4.187832255138415505, 99.99999999999998579, -21.50835573230103037 ) ) ;
#4324=ORIENTED_EDGE ( 'NONE', *, *, #780, .T. ) ;
#4325=CARTESIAN_POINT ( 'NONE',  ( 3.222930479149370253, 99.99999999999998579, -22.15251218086615381 ) ) ;
#4326=CARTESIAN_POINT ( 'NONE',  ( -4.959819536546781389E-15, 4.399999997815050357, 27.00000000000000355 ) ) ;
#4327=DIRECTION ( 'NONE',  ( -0.9198211419112228837, 0.000000000000000000, 0.3923379498508065000 ) ) ;
#4328=CARTESIAN_POINT ( 'NONE',  ( -21.87421819196487505, 100.0000000000000000, -9.684578881761979119 ) ) ;
#4329=CARTESIAN_POINT ( 'NONE',  ( 3.434779879277784609, 100.0000000000000142, -23.17575050830969374 ) ) ;
#4330=CARTESIAN_POINT ( 'NONE',  ( -22.16320288552370243, 100.0000000000000142, -10.86869938533413915 ) ) ;
#4333=ORIENTED_EDGE ( 'NONE', *, *, #5586, .F. ) ;
#4336=CARTESIAN_POINT ( 'NONE',  ( -15.17782247516205274, 99.49999999999998579, 15.06300032623928686 ) ) ;
#4337=CARTESIAN_POINT ( 'NONE',  ( 3.044406660298407452, 99.50000000000000000, -23.15442635585071685 ) ) ;
#4338=CARTESIAN_POINT ( 'NONE',  ( 11.36312591709336139, 3.599999998907525089, -27.43301270000000258 ) ) ;
#4339=CARTESIAN_POINT ( 'NONE',  ( -20.52076770522338833, 100.0000000000000000, -10.69798695537560462 ) ) ;
#4340=CARTESIAN_POINT ( 'NONE',  ( -21.30928386698190025, 99.50000000000000000, -11.02857376369709996 ) ) ;
#4341=CARTESIAN_POINT ( 'NONE',  ( 4.259295290443009918, 100.0000000000000284, -24.34414156132068996 ) ) ;
#4342=CARTESIAN_POINT ( 'NONE',  ( -19.09188309203678457, 4.099999997815050534, -19.09188309203678813 ) ) ;
#4348=LINE ( 'NONE', #1055, #356 ) ;
#4349=EDGE_CURVE ( 'NONE', #827, #7488, #4093, .T. ) ;
#4350=CARTESIAN_POINT ( 'NONE',  ( 4.486604876299897349, 100.0000000000000000, -21.85617661337775885 ) ) ;
#4351=DIRECTION ( 'NONE',  ( 0.000000000000000000, 0.000000000000000000, 1.000000000000000000 ) ) ;
#4353=DIRECTION ( 'NONE',  ( 0.000000000000000000, 0.000000000000000000, -1.000000000000000000 ) ) ;
#4354=ORIENTED_EDGE ( 'NONE', *, *, #5881, .T. ) ;
#4355=CARTESIAN_POINT ( 'NONE',  ( 0.000000000000000000, 100.0000000000000000, 0.000000000000000000 ) ) ;
#4357=ORIENTED_EDGE ( 'NONE', *, *, #7145, .T. ) ;
#4358=CARTESIAN_POINT ( 'NONE',  ( -22.28738277804067636, 99.49999999999997158, -10.06255608345902886 ) ) ;
#4359=CARTESIAN_POINT ( 'NONE',  ( 9.820792995160308791, 99.50000000000000000, 20.21220011423140761 ) ) ;
#4360=LINE ( 'NONE', #496, #8090 ) ;
#4361=CARTESIAN_POINT ( 'NONE',  ( 1.653273178848927064E-15, 3.199999997815050623, -27.00000000000000355 ) ) ;
#4363=CARTESIAN_POINT ( 'NONE',  ( -16.52319226728147328, 99.99999999999994316, 15.63609008536095324 ) ) ;
#4364=CARTESIAN_POINT ( 'NONE',  ( 4.118246196500586542, 99.49999999999998579, -21.10643963665684453 ) ) ;
#4365=ORIENTED_EDGE ( 'NONE', *, *, #2818, .T. ) ;
#4367=CARTESIAN_POINT ( 'NONE',  ( 9.563602730896748838, 100.0000000000000142, 20.87184380654744587 ) ) ;
#4370=CARTESIAN_POINT ( 'NONE',  ( 11.36312591709336139, 5.299999998907526155, -27.43301270000000258 ) ) ;
#4373=CARTESIAN_POINT ( 'NONE',  ( -18.01369080470046313, 100.0000000000000000, 17.15556831233607937 ) ) ;
#4374=CARTESIAN_POINT ( 'NONE',  ( 4.154273145530666511, 99.50000000000000000, -22.82723029927519676 ) ) ;
#4376=CARTESIAN_POINT ( 'NONE',  ( 3.212364564527730337, 99.50000000000000000, -22.10366694310577884 ) ) ;
#4377=CARTESIAN_POINT ( 'NONE',  ( -11.18376618407356560, 4.049999997815050712, -27.00000000000000355 ) ) ;
#4378=DIRECTION ( 'NONE',  ( 0.000000000000000000, 1.000000000000000000, 0.000000000000000000 ) ) ;
#4380=AXIS2_PLACEMENT_3D ( 'NONE', #8079, #908, #7526 ) ;
#4382=ORIENTED_EDGE ( 'NONE', *, *, #8558, .T. ) ;
#4383=CARTESIAN_POINT ( 'NONE',  ( 4.901590909071964042, 99.50000000000000000, -23.62641080846013608 ) ) ;
#4384=CARTESIAN_POINT ( 'NONE',  ( -11.36312591709337561, 1.699999998907525178, 27.43301269999999548 ) ) ;
#4385=ORIENTED_EDGE ( 'NONE', *, *, #3721, .T. ) ;
#4387=( BOUNDED_CURVE ( )  B_SPLINE_CURVE ( 2, ( #3223, #6410, #915, #8767, #4007, #7192, #9696, #5680, #2974 ),
 .UNSPECIFIED., .F., .F. ) 
 B_SPLINE_CURVE_WITH_KNOTS ( ( 3, 2, 2, 2, 3 ),
 ( 0.03571428571428571230, 0.05357142857142856845, 0.07142857142857142461, 0.08928571428571428770, 0.1071428571428571369 ),
 .UNSPECIFIED. ) 
 CURVE ( )  GEOMETRIC_REPRESENTATION_ITEM ( )  RATIONAL_B_SPLINE_CURVE ( ( 1.000000000000000000, 0.9238795325112867385, 1.000000000000000000, 0.9238795325112867385, 1.000000000000000000, 0.9238795325112867385, 1.000000000000000000, 0.9238795325112867385, 1.000000000000000000 ) ) 
 REPRESENTATION_ITEM ( '' )  );
#4389=CARTESIAN_POINT ( 'NONE',  ( -14.75894607058735630, 99.50000000000002842, 15.77473972644577849 ) ) ;
#4391=CARTESIAN_POINT ( 'NONE',  ( -11.36312591709335962, 1.299999998907525267, -27.43301270000000258 ) ) ;
#4394=CARTESIAN_POINT ( 'NONE',  ( -15.76250887235353737, 99.99999999999998579, 16.65066592061022277 ) ) ;
#4395=DIRECTION ( 'NONE',  ( 0.000000000000000000, 0.000000000000000000, -1.000000000000000000 ) ) ;
#4396=CARTESIAN_POINT ( 'NONE',  ( 7.826802610544922878, 100.0000000000000000, 21.21129867192371421 ) ) ;
#4397=EDGE_CURVE ( 'NONE', #7345, #4075, #9588, .T. ) ;
#4398=CARTESIAN_POINT ( 'NONE',  ( 4.143207896384923039, 99.99999999999998579, -24.36264353342416911 ) ) ;
#4399=CARTESIAN_POINT ( 'NONE',  ( -21.03505001771060634, 99.50000000000000000, -9.476849197711761263 ) ) ;
#4400=CARTESIAN_POINT ( 'NONE',  ( 21.82251602564102910, 99.50000000000000000, -0.5181290064102563875 ) ) ;
#4401=ORIENTED_EDGE ( 'NONE', *, *, #6874, .T. ) ;
#4403=CARTESIAN_POINT ( 'NONE',  ( -27.43301270000000969, 0.6999999989075252893, 11.36312591709335429 ) ) ;
#4404=B_SPLINE_CURVE_WITH_KNOTS ( 'NONE', 3,
 ( #8206, #5058, #72, #7515, #355, #1089, #4232, #8995, #7464, #9874, #5803, #5162, #1139, #2482, #3546 ),
 .UNSPECIFIED., .F., .F.,
 ( 4, 1, 1, 1, 1, 1, 1, 1, 1, 1, 1, 1, 4 ),
 ( 0.000000000000000000, 0.08963690308348271074, 0.1775767702671464110, 0.2649576542713044658, 0.3533131777157214604, 0.4402865524342069459, 0.5245518675747646853, 0.6066224975438009315, 0.6889424263984335051, 0.7698335385027974542, 0.8475882324521423206, 0.9236428641877653112, 1.000000000000000000 ),
 .UNSPECIFIED. ) ;
#4406=CARTESIAN_POINT ( 'NONE',  ( -16.49882833452567965, 99.50000000000000000, 15.05677840364783115 ) ) ;
#4407=CARTESIAN_POINT ( 'NONE',  ( 9.342627931057743140, 99.50000000000000000, 21.59831790269294771 ) ) ;
#4408=LINE ( 'NONE', #6808, #7958 ) ;
#4410=DIRECTION ( 'NONE',  ( 0.000000000000000000, -0.000000000000000000, 1.000000000000000000 ) ) ;
#4413=CARTESIAN_POINT ( 'NONE',  ( 4.523042264738025509, 99.50000000000001421, -24.25177047807976294 ) ) ;
#4414=CARTESIAN_POINT ( 'NONE',  ( 27.43301270000000258, 1.049999998907525267, 0.000000000000000000 ) ) ;
#4415=CARTESIAN_POINT ( 'NONE',  ( 3.328702480760086235, 99.49999999999997158, -23.35145716610488975 ) ) ;
#4417=VECTOR ( 'NONE', #854, 1000.000000000000114 ) ;
#4419=EDGE_CURVE ( 'NONE', #5889, #2532, #1634, .T. ) ;
#4421=CARTESIAN_POINT ( 'NONE',  ( -16.87593989452418697, 99.99999999999998579, 15.58794934546231126 ) ) ;
#4422=CARTESIAN_POINT ( 'NONE',  ( -15.15193744131588183, 99.50000000000001421, 16.74589488344418697 ) ) ;
#4423=EDGE_LOOP ( 'NONE', ( #2758, #6720, #6249, #71 ) ) ;
#4424=CARTESIAN_POINT ( 'NONE',  ( 4.909381318607588973, 99.50000000000000000, -23.54377677363417121 ) ) ;
#4425=CARTESIAN_POINT ( 'NONE',  ( -19.39806930854668465, 2.449999998907525622, 19.39806930854667755 ) ) ;
#4427=FACE_OUTER_BOUND ( 'NONE', #4423, .T. ) ;
#4428=CARTESIAN_POINT ( 'NONE',  ( -21.69499712064247277, 99.99999999999998579, -9.295461156691713356 ) ) ;
#4429=CARTESIAN_POINT ( 'NONE',  ( 8.961048541867139505, 99.50000000000001421, 19.57961630251783092 ) ) ;
#4430=CARTESIAN_POINT ( 'NONE',  ( 0.000000000000000000, 100.0000000000000000, 0.000000000000000000 ) ) ;
#4434=CARTESIAN_POINT ( 'NONE',  ( -16.49816537377288128, 100.0000000000000000, 16.70951083495554101 ) ) ;
#4435=CARTESIAN_POINT ( 'NONE',  ( 11.36312591709336139, 2.899999998907526244, -27.43301270000000258 ) ) ;
#4438=EDGE_CURVE ( 'NONE', #4897, #1073, #3668, .T. ) ;
#4439=CARTESIAN_POINT ( 'NONE',  ( 3.203979444200292015, 99.99999999999997158, -21.29640115293693725 ) ) ;
#4441=CARTESIAN_POINT ( 'NONE',  ( 11.36312591709336139, 5.199999998907525622, -27.43301270000000258 ) ) ;
#4442=CARTESIAN_POINT ( 'NONE',  ( -5.039362679103552881E-15, 0.9499999989075252893, 27.43301270000000258 ) ) ;
#4443=ORIENTED_EDGE ( 'NONE', *, *, #1477, .T. ) ;
#4445=CARTESIAN_POINT ( 'NONE',  ( -15.83671465916681242, 100.0000000000000000, 16.65403364262263608 ) ) ;
#4447=CARTESIAN_POINT ( 'NONE',  ( -19.09188309203678813, 4.299999997815050712, 19.09188309203678457 ) ) ;
#4448=CARTESIAN_POINT ( 'NONE',  ( 4.202475441399873723, 100.0000000000000000, -24.35385978717689071 ) ) ;
#4454=CARTESIAN_POINT ( 'NONE',  ( -5.039362679103552881E-15, 2.449999998907525178, 27.43301270000000258 ) ) ;
#4455=CARTESIAN_POINT ( 'NONE',  ( -15.17782247516205274, 99.49999999999998579, 15.06300032623928686 ) ) ;
#4457=CARTESIAN_POINT ( 'NONE',  ( 9.468852706215191262, 99.50000000000000000, 21.22967007823213237 ) ) ;
#4458=CARTESIAN_POINT ( 'NONE',  ( -17.94007301623892658, 99.50000000000000000, 17.49000340848992607 ) ) ;
#4459=ORIENTED_EDGE ( 'NONE', *, *, #8874, .T. ) ;
#4461=CARTESIAN_POINT ( 'NONE',  ( 9.248677610544923766, 99.50000000000000000, 22.83089001807756446 ) ) ;
#4464=CARTESIAN_POINT ( 'NONE',  ( -22.00707282958688182, 99.99999999999994316, -9.748971510896797810 ) ) ;
#4467=CARTESIAN_POINT ( 'NONE',  ( 4.061354557346970040, 99.49999999999997158, -22.84864678426182039 ) ) ;
#4471=CARTESIAN_POINT ( 'NONE',  ( -27.00000000000001421, 1.250000000000000222, 11.18376618407356560 ) ) ;
#4475=CARTESIAN_POINT ( 'NONE',  ( 11.18376618407357093, 1.549999997815050490, -27.00000000000000355 ) ) ;
#4476=CARTESIAN_POINT ( 'NONE',  ( -19.39806930854668465, 4.849999998907525978, 19.39806930854667755 ) ) ;
#4478=ADVANCED_FACE ( 'NONE', ( #209 ), #3269, .T. ) ;
#4479=VECTOR ( 'NONE', #190, 1000.000000000000000 ) ;
#4480=CARTESIAN_POINT ( 'NONE',  ( -16.63177974700816009, 100.0000000000000000, 16.59747536361813403 ) ) ;
#4481=ORIENTED_EDGE ( 'NONE', *, *, #5282, .F. ) ;
#4483=CARTESIAN_POINT ( 'NONE',  ( 4.850954546176396320, 99.49999999999998579, -24.43907202982397209 ) ) ;
#4485=CARTESIAN_POINT ( 'NONE',  ( 9.513000527211589841, 99.50000000000000000, 20.35102222961602436 ) ) ;
#4486=B_SPLINE_CURVE_WITH_KNOTS ( 'NONE', 3,
 ( #6663, #8238, #2552, #9857, #6613, #2694, #7351, #8150, #2643, #1019, #4904, #3332, #4946, #4122, #5834, #285, #8883, #5885, #1845 ),
 .UNSPECIFIED., .F., .F.,
 ( 4, 1, 1, 1, 1, 1, 1, 1, 1, 1, 1, 1, 1, 1, 1, 1, 4 ),
 ( 0.000000000000000000, 0.06282509715607415002, 0.1231380613775250599, 0.1822388757841713336, 0.2396184841454026548, 0.2973605923678978580, 0.3541959668311244203, 0.4122907788200148582, 0.4717534157231769720, 0.5322282553174864095, 0.5926403291039165078, 0.6546871955647078911, 0.7179012776534754448, 0.7839155840457150415, 0.8527518695723632636, 0.9242989153657757972, 1.000000000000000000 ),
 .UNSPECIFIED. ) ;
#4487=ORIENTED_EDGE ( 'NONE', *, *, #3252, .F. ) ;
#4488=CARTESIAN_POINT ( 'NONE',  ( -15.37731512048643268, 99.50000000000000000, 15.34394520743122214 ) ) ;
#4489=DIRECTION ( 'NONE',  ( -0.000000000000000000, 1.000000000000000000, -0.000000000000000000 ) ) ;
#4492=CARTESIAN_POINT ( 'NONE',  ( 8.612131858919537919, 99.49999999999998579, 19.96100069886393413 ) ) ;
#4493=CARTESIAN_POINT ( 'NONE',  ( 3.551917533706515417, 99.50000000000001421, -21.11785906961830150 ) ) ;
#4495=CARTESIAN_POINT ( 'NONE',  ( -16.90147242988460263, 99.49999999999998579, 15.68472263728856753 ) ) ;
#4496=CARTESIAN_POINT ( 'NONE',  ( 27.43301269999999548, 1.099999998907525089, 11.36312591709337738 ) ) ;
#4499=DIRECTION ( 'NONE',  ( -6.482089281916151093E-13, -1.000000000000000000, -1.430867686834485556E-12 ) ) ;
#4500=CARTESIAN_POINT ( 'NONE',  ( 3.673732336774000018, 99.50000000000000000, -21.43557726391590279 ) ) ;
#4501=B_SPLINE_SURFACE_WITH_KNOTS ( 'NONE', 3, 1, ( 
 ( #3657, #7790 ),
 ( #4538, #3868 ),
 ( #4488, #6219 ),
 ( #7735, #6891 ),
 ( #5445, #620 ),
 ( #7054, #2076 ),
 ( #8468, #517 ),
 ( #10088, #10261 ),
 ( #4654, #2924 ),
 ( #10205, #6108 ),
 ( #9299, #8638 ),
 ( #9195, #2015 ),
 ( #8525, #5213 ),
 ( #8413, #4906 ),
 ( #9523, #4704 ),
 ( #8101, #4125 ),
 ( #2505, #7107 ),
 ( #7896, #6428 ),
 ( #5546, #6329 ) ),
 .UNSPECIFIED., .F., .F., .F.,
 ( 4, 1, 1, 1, 1, 1, 1, 1, 1, 1, 1, 1, 1, 1, 1, 1, 4 ),
 ( 2, 2 ),
 ( 0.000000000000000000, 0.06485467887857676583, 0.1277145915909605745, 0.1892127134908106190, 0.2497332716026948729, 0.3109554005383074471, 0.3726238983726959941, 0.4350931267523188151, 0.5000867325104639827, 0.5644742510850394579, 0.6276292343746815439, 0.6888483565510189477, 0.7500704854866314664, 0.8105910435985150819, 0.8724026516570742018, 0.9351453211214243444, 1.000000000000000000 ),
 ( 0.000000000000000000, 1.000000000000000000 ),
 .UNSPECIFIED. ) ;
#4502=CARTESIAN_POINT ( 'NONE',  ( 3.320270046935387853, 99.99999999999998579, -23.88810568987970484 ) ) ;
#4505=CARTESIAN_POINT ( 'NONE',  ( 4.820889542125314620, 99.49999999999998579, -21.76289454767624676 ) ) ;
#4508=CARTESIAN_POINT ( 'NONE',  ( 27.43301269999999548, 0.9999999989075252227, 11.36312591709337738 ) ) ;
#4509=CARTESIAN_POINT ( 'NONE',  ( -15.10737684033046335, 99.50000000000000000, 15.12848924955281049 ) ) ;
#4510=CARTESIAN_POINT ( 'NONE',  ( -27.00000000000000355, 2.000000000000000000, -3.306546357697854128E-15 ) ) ;
#4514=CARTESIAN_POINT ( 'NONE',  ( 4.852629679480013891, 100.0000000000000142, -23.84752007312514621 ) ) ;
#4517=ADVANCED_FACE ( 'NONE', ( #9937, #9877 ), #412, .F. ) ;
#4518=CARTESIAN_POINT ( 'NONE',  ( -22.12191435419165941, 99.50000000000001421, -9.834338183724410598 ) ) ;
#4519=CARTESIAN_POINT ( 'NONE',  ( 2.204364238465235428E-15, 100.0000000000000000, -18.00000000000000000 ) ) ;
#4522=CARTESIAN_POINT ( 'NONE',  ( 5.226890989224467710, 100.0000000000000284, -23.72545275563321354 ) ) ;
#4523=DIRECTION ( 'NONE',  ( -0.000000000000000000, -1.000000000000000000, -0.000000000000000000 ) ) ;
#4530=CARTESIAN_POINT ( 'NONE',  ( 9.861577898019769250, 99.99999999999994316, 21.03794551367759169 ) ) ;
#4531=ORIENTED_EDGE ( 'NONE', *, *, #6072, .F. ) ;
#4532=CARTESIAN_POINT ( 'NONE',  ( 8.685676809262872666, 99.50000000000000000, 23.43455588346217766 ) ) ;
#4534=ADVANCED_FACE ( 'NONE', ( #5962 ), #1769, .T. ) ;
#4535=DIRECTION ( 'NONE',  ( 0.000000000000000000, -0.000000000000000000, 1.000000000000000000 ) ) ;
#4537=EDGE_CURVE ( 'NONE', #1184, #341, #10157, .T. ) ;
#4538=CARTESIAN_POINT ( 'NONE',  ( -15.34161522349497808, 99.49999999999998579, 15.37783959465231121 ) ) ;
#4539=VECTOR ( 'NONE', #4698, 1000.000000000000227 ) ;
#4541=VECTOR ( 'NONE', #1822, 1000.000000000000000 ) ;
#4544=ADVANCED_FACE ( 'NONE', ( #1355 ), #8530, .T. ) ;
#4546=DIRECTION ( 'NONE',  ( -0.8660254037844393737, 0.4999999999999986677, 0.000000000000000000 ) ) ;
#4549=CARTESIAN_POINT ( 'NONE',  ( -16.70213339477928471, 99.49999999999998579, 16.52464093453885852 ) ) ;
#4550=CARTESIAN_POINT ( 'NONE',  ( -19.39806930854668465, 3.249999998907525001, 19.39806930854667755 ) ) ;
#4551=ORIENTED_EDGE ( 'NONE', *, *, #9899, .T. ) ;
#4553=CARTESIAN_POINT ( 'NONE',  ( 9.357053078540884528, 100.0000000000000142, 19.70216357796830664 ) ) ;
#4554=CARTESIAN_POINT ( 'NONE',  ( -19.46743691185369585, 100.0000000000000000, -8.912588186774021537 ) ) ;
#4560=ORIENTED_EDGE ( 'NONE', *, *, #5048, .T. ) ;
#4562=CARTESIAN_POINT ( 'NONE',  ( -27.43301270000000258, 2.249999998907525001, -3.359575119402369376E-15 ) ) ;
#4564=EDGE_LOOP ( 'NONE', ( #4354, #4385, #10015, #612 ) ) ;
#4565=B_SPLINE_CURVE_WITH_KNOTS ( 'NONE', 3,
 ( #4396, #6067, #9258, #9998, #2089, #3560, #7635, #9106, #8482, #4243, #1927, #1152, #5124, #6015, #7424, #1876, #266, #5227, #3455 ),
 .UNSPECIFIED., .F., .F.,
 ( 4, 1, 1, 1, 1, 1, 1, 1, 1, 1, 1, 1, 1, 1, 1, 1, 4 ),
 ( 0.000000000000000000, 0.06839333837245492598, 0.1346519561570838353, 0.1985335841112251809, 0.2613354512981445610, 0.3228799447584090876, 0.3842093944964607433, 0.4462111754260434937, 0.5089246482083435996, 0.5715029624870164859, 0.6324491702983550123, 0.6923675070709934820, 0.7521785462597534444, 0.8119602890481165680, 0.8728645645504365946, 0.9355733815441056311, 1.000000000000000000 ),
 .UNSPECIFIED. ) ;
#4566=CARTESIAN_POINT ( 'NONE',  ( -20.96643530928959365, 99.50000000000000000, -10.05541671241504886 ) ) ;
#4567=CARTESIAN_POINT ( 'NONE',  ( -27.00000000000000355, 1.150000000000000133, -11.18376618407357093 ) ) ;
#4569=VERTEX_POINT ( 'NONE', #8589 ) ;
#4570=CARTESIAN_POINT ( 'NONE',  ( -19.09188309203678457, 2.700000000000000178, -19.09188309203678813 ) ) ;
#4571=CARTESIAN_POINT ( 'NONE',  ( 8.074269155311188939, 100.0000000000000142, 20.56111086218762551 ) ) ;
#4574=ORIENTED_EDGE ( 'NONE', *, *, #7111, .T. ) ;
#4576=LINE ( 'NONE', #9960, #8809 ) ;
#4579=CARTESIAN_POINT ( 'NONE',  ( 3.080354370726382296, 100.0000000000000426, -23.09295995363041598 ) ) ;
#4580=ADVANCED_FACE ( 'NONE', ( #5276 ), #7006, .T. ) ;
#4581=CARTESIAN_POINT ( 'NONE',  ( 4.486604876299897349, 99.50000000000000000, -21.85617661337775885 ) ) ;
#4582=CARTESIAN_POINT ( 'NONE',  ( -17.94007301623892658, 100.0000000000000000, 17.49000340848992607 ) ) ;
#4584=FACE_OUTER_BOUND ( 'NONE', #3410, .T. ) ;
#4585=ORIENTED_EDGE ( 'NONE', *, *, #3307, .F. ) ;
#4586=LINE ( 'NONE', #5489, #1556 ) ;
#4590=B_SPLINE_SURFACE_WITH_KNOTS ( 'NONE', 3, 1, ( 
 ( #4816, #7959 ),
 ( #792, #3983 ),
 ( #8796, #1621 ),
 ( #8012, #8848 ),
 ( #8255, #1084 ),
 ( #3435, #201 ),
 ( #1760, #1811 ) ),
 .UNSPECIFIED., .F., .F., .F.,
 ( 4, 1, 1, 1, 4 ),
 ( 2, 2 ),
 ( 0.000000000000000000, 0.2676680225848128147, 0.5230972062070123885, 0.7658030722156558001, 1.000000000000000000 ),
 ( 0.000000000000000000, 1.000000000000000000 ),
 .UNSPECIFIED. ) ;
#4591=ORIENTED_EDGE ( 'NONE', *, *, #5314, .T. ) ;
#4592=CARTESIAN_POINT ( 'NONE',  ( -20.95972469638759250, 100.0000000000000000, -9.536167108072199028 ) ) ;
#4593=CARTESIAN_POINT ( 'NONE',  ( 9.063633472794011325, 99.99999999999998579, 19.59517414759687526 ) ) ;
#4594=DIRECTION ( 'NONE',  ( 1.000000000000000000, 0.000000000000000000, 0.000000000000000000 ) ) ;
#4595=CARTESIAN_POINT ( 'NONE',  ( -16.57337958714257908, 99.49999999999998579, 15.99273699073067867 ) ) ;
#4597=CARTESIAN_POINT ( 'NONE',  ( -16.49816537377288128, 99.50000000000000000, 16.70951083495554101 ) ) ;
#4598=CARTESIAN_POINT ( 'NONE',  ( 11.36312591709336850, 0.9999999989075253337, 27.43301269999999903 ) ) ;
#4599=ORIENTED_EDGE ( 'NONE', *, *, #10245, .T. ) ;
#4602=VECTOR ( 'NONE', #5895, 1000.000000000000000 ) ;
#4603=CARTESIAN_POINT ( 'NONE',  ( 3.681717055787076642, 99.50000000000000000, -21.09125273517263111 ) ) ;
#4605=CARTESIAN_POINT ( 'NONE',  ( 27.00000000000000355, 0.6499999978150503566, -11.18376618407356915 ) ) ;
#4606=CARTESIAN_POINT ( 'NONE',  ( 27.43301270000000258, 3.599999998907525534, -11.36312591709336139 ) ) ;
#4607=CARTESIAN_POINT ( 'NONE',  ( -15.42740294075255925, 100.0000000000000000, 14.91894146668702348 ) ) ;
#4609=CARTESIAN_POINT ( 'NONE',  ( 3.202955020264580899, 99.50000000000000000, -21.91595956354277064 ) ) ;
#4610=AXIS2_PLACEMENT_3D ( 'NONE', #4291, #4191, #7422 ) ;
#4611=CARTESIAN_POINT ( 'NONE',  ( -15.98972951825121669, 99.99999999999997158, 15.19400804711857411 ) ) ;
#4613=CARTESIAN_POINT ( 'NONE',  ( 4.034460619503033030, 99.49999999999995737, -21.08676866017170681 ) ) ;
#4617=CIRCLE ( 'NONE', #5623, 18.00000000000000000 ) ;
#4618=CARTESIAN_POINT ( 'NONE',  ( -19.39806930854667755, 2.949999998907525178, -19.39806930854668110 ) ) ;
#4624=CARTESIAN_POINT ( 'NONE',  ( 26.99999999999999645, 2.350000000000000533, 11.18376618407358691 ) ) ;
#4625=CARTESIAN_POINT ( 'NONE',  ( 9.114876806416853938, 99.49999999999998579, 19.97295714941878231 ) ) ;
#4626=ORIENTED_EDGE ( 'NONE', *, *, #624, .F. ) ;
#4627=CARTESIAN_POINT ( 'NONE',  ( -16.57687742313193269, 99.50000000000002842, 15.91855687263828756 ) ) ;
#4629=ORIENTED_EDGE ( 'NONE', *, *, #8891, .F. ) ;
#4636=CARTESIAN_POINT ( 'NONE',  ( 3.058419780146050648, 100.0000000000000000, -23.12871267107006545 ) ) ;
#4640=CARTESIAN_POINT ( 'NONE',  ( 4.640952353770416927, 100.0000000000000142, -24.17064508475253604 ) ) ;
#4646=CARTESIAN_POINT ( 'NONE',  ( -21.13504512532655610, 100.0000000000000000, -11.31853095674525100 ) ) ;
#4649=CARTESIAN_POINT ( 'NONE',  ( 8.536201443755420115, 100.0000000000000284, 19.63502355897212581 ) ) ;
#4651=LINE ( 'NONE', #8686, #6651 ) ;
#4653=B_SPLINE_CURVE_WITH_KNOTS ( 'NONE', 3,
 ( #849, #8293, #4087, #9634, #6771, #56, #3530, #2469, #1953, #5941, #8853, #6666, #4039, #1124, #7272 ),
 .UNSPECIFIED., .F., .F.,
 ( 4, 1, 1, 1, 1, 1, 1, 1, 1, 1, 1, 1, 4 ),
 ( 0.000000000000000000, 0.09895296010982183865, 0.1966578232739713550, 0.2939931048315790330, 0.3929322324600736938, 0.4463669803336778319, 0.5055752425223922764, 0.5715235163887821823, 0.6440401046887170855, 0.7229629404452876384, 0.8087840669208056221, 0.9009145765370688563, 1.000000000000000000 ),
 .UNSPECIFIED. ) ;
#4654=CARTESIAN_POINT ( 'NONE',  ( -15.76955986605724647, 99.49999999999998579, 15.18352214517458698 ) ) ;
#4655=CARTESIAN_POINT ( 'NONE',  ( 11.36312591709336850, 3.399999998907525356, 27.43301269999999903 ) ) ;
#4657=ADVANCED_FACE ( 'NONE', ( #6224 ), #6270, .T. ) ;
#4661=CARTESIAN_POINT ( 'NONE',  ( -16.65546786808457469, 99.49999999999998579, 16.57295196178722918 ) ) ;
#4662=CARTESIAN_POINT ( 'NONE',  ( 27.43301270000000258, 1.199999998907525178, -11.36312591709336139 ) ) ;
#4663=ORIENTED_EDGE ( 'NONE', *, *, #8315, .T. ) ;
#4665=CARTESIAN_POINT ( 'NONE',  ( -15.22320097062094568, 99.50000000000001421, 16.32303119091969634 ) ) ;
#4666=CARTESIAN_POINT ( 'NONE',  ( 3.970307086022987431, 99.50000000000001421, -24.36314111580913178 ) ) ;
#4670=CARTESIAN_POINT ( 'NONE',  ( 3.771794781161601939, 99.99999999999998579, -21.07813736596861176 ) ) ;
#4671=ORIENTED_EDGE ( 'NONE', *, *, #237, .F. ) ;
#4672=EDGE_CURVE ( 'NONE', #405, #7350, #6311, .T. ) ;
#4674=CARTESIAN_POINT ( 'NONE',  ( -27.43301270000000258, 2.199999998907525622, -11.36312591709336317 ) ) ;
#4675=DIRECTION ( 'NONE',  ( -0.000000000000000000, -1.000000000000000000, -0.000000000000000000 ) ) ;
#4676=EDGE_LOOP ( 'NONE', ( #1284, #9665 ) ) ;
#4677=CARTESIAN_POINT ( 'NONE',  ( 7.826802610544922878, 100.0000000000000000, 21.21129867192371421 ) ) ;
#4678=CARTESIAN_POINT ( 'NONE',  ( 8.564701892180647036, 99.50000000000000000, 19.97971282122689018 ) ) ;
#4679=VERTEX_POINT ( 'NONE', #3292 ) ;
#4680=CARTESIAN_POINT ( 'NONE',  ( -15.11748654497029953, 99.49999999999998579, 15.76872032455190897 ) ) ;
#4681=CARTESIAN_POINT ( 'NONE',  ( 8.063732359723156051, 99.50000000000001421, 20.72384750152746236 ) ) ;
#4682=EDGE_CURVE ( 'NONE', #3916, #8960, #9035, .T. ) ;
#4683=EDGE_LOOP ( 'NONE', ( #2788, #4919, #4365, #6190 ) ) ;
#4685=ORIENTED_EDGE ( 'NONE', *, *, #651, .F. ) ;
#4687=CARTESIAN_POINT ( 'NONE',  ( 19.39806930854668110, 1.949999998907525178, -19.39806930854668110 ) ) ;
#4688=CARTESIAN_POINT ( 'NONE',  ( -21.45221949983897858, 99.50000000000000000, -9.661157428473494235 ) ) ;
#4689=B_SPLINE_SURFACE_WITH_KNOTS ( 'NONE', 3, 1, ( 
 ( #7933, #4480 ),
 ( #767, #5204 ),
 ( #10348, #2006 ),
 ( #3958, #6364 ),
 ( #9558, #2387 ),
 ( #5582, #3592 ),
 ( #1234, #4982 ),
 ( #964, #5631 ),
 ( #8821, #1696 ),
 ( #1597, #8919 ),
 ( #8036, #1010 ),
 ( #9653, #1650 ),
 ( #175, #4788 ),
 ( #2490, #869 ),
 ( #8969, #8180 ),
 ( #8088, #5683 ),
 ( #4893, #4201 ),
 ( #4010, #4158 ),
 ( #9700, #7385 ) ),
 .UNSPECIFIED., .F., .F., .F.,
 ( 4, 1, 1, 1, 1, 1, 1, 1, 1, 1, 1, 1, 1, 1, 1, 1, 4 ),
 ( 2, 2 ),
 ( 0.000000000000000000, 0.06363772181477481138, 0.1253661190162797812, 0.1854850957718461035, 0.2454326483351531030, 0.3054881917026986415, 0.3659564384638642753, 0.4275766838088623234, 0.4913505196498278993, 0.5556437034595619329, 0.6183735394983103095, 0.6802114403575724166, 0.7422401234104337719, 0.8041288543812358247, 0.8678488776753463529, 0.9326351893241184854, 1.000000000000000000 ),
 ( 0.000000000000000000, 1.000000000000000000 ),
 .UNSPECIFIED. ) ;
#4691=CARTESIAN_POINT ( 'NONE',  ( 4.922541232168287983, 99.50000000000002842, -24.37252920941159928 ) ) ;
#4692=CARTESIAN_POINT ( 'NONE',  ( 1.653273178848927064E-15, 4.799999997815051600, -27.00000000000000355 ) ) ;
#4694=VERTEX_POINT ( 'NONE', #8843 ) ;
#4695=CARTESIAN_POINT ( 'NONE',  ( 4.739008722453743161, 99.50000000000000000, -24.06821587619827341 ) ) ;
#4696=CARTESIAN_POINT ( 'NONE',  ( -20.66709314808276332, 99.50000000000002842, -10.01107456535036455 ) ) ;
#4697=ORIENTED_EDGE ( 'NONE', *, *, #2750, .T. ) ;
#4698=DIRECTION ( 'NONE',  ( -0.3368610894541371747, 0.000000000000000000, 0.9415543565890243105 ) ) ;
#4700=CARTESIAN_POINT ( 'NONE',  ( -22.33529725360453000, 99.99999999999997158, -10.20112572733487255 ) ) ;
#4701=CARTESIAN_POINT ( 'NONE',  ( 9.600410285814406919, 99.99999999999998579, 19.87914582625927196 ) ) ;
#4702=DIRECTION ( 'NONE',  ( -0.000000000000000000, 1.000000000000000000, -0.000000000000000000 ) ) ;
#4704=CARTESIAN_POINT ( 'NONE',  ( -16.18965924272485779, 99.99999999999998579, 15.26525457555968224 ) ) ;
#4705=CARTESIAN_POINT ( 'NONE',  ( 27.43301270000000258, 3.549999998907525267, 0.000000000000000000 ) ) ;
#4706=ORIENTED_EDGE ( 'NONE', *, *, #5641, .T. ) ;
#4708=CARTESIAN_POINT ( 'NONE',  ( 3.293841816516395848, 99.49999999999998579, -23.44781013845121009 ) ) ;
#4710=CARTESIAN_POINT ( 'NONE',  ( 3.764204346677844093, 100.0000000000000426, -22.52576385118515745 ) ) ;
#4711=CARTESIAN_POINT ( 'NONE',  ( -27.00000000000000355, 1.749999997815050667, -11.18376618407357093 ) ) ;
#4712=ADVANCED_FACE ( 'NONE', ( #1669 ), #9455, .T. ) ;
#4713=CARTESIAN_POINT ( 'NONE',  ( -15.13520964245927836, 99.99999999999995737, 15.69931698147095034 ) ) ;
#4714=CARTESIAN_POINT ( 'NONE',  ( 3.286905236079108672, 100.0000000000000426, -23.77014634954566574 ) ) ;
#4715=CARTESIAN_POINT ( 'NONE',  ( 3.446946945638383664, 99.49999999999997158, -21.53774374131874580 ) ) ;
#4716=CARTESIAN_POINT ( 'NONE',  ( -22.59920249870969045, 99.99999999999998579, -10.80326527670058567 ) ) ;
#4718=CARTESIAN_POINT ( 'NONE',  ( -21.11719860449141351, 99.50000000000002842, -9.425423427278841970 ) ) ;
#4719=ORIENTED_EDGE ( 'NONE', *, *, #319, .F. ) ;
#4720=VERTEX_POINT ( 'NONE', #9088 ) ;
#4722=CARTESIAN_POINT ( 'NONE',  ( -19.39806930854667755, 4.549999998907525267, -19.39806930854668110 ) ) ;
#4723=CARTESIAN_POINT ( 'NONE',  ( -16.38049141020750099, 99.50000000000004263, 14.97568473612765416 ) ) ;
#4724=CARTESIAN_POINT ( 'NONE',  ( 11.18376618407356915, 0.1499999999999999944, -27.00000000000000355 ) ) ;
#4725=CYLINDRICAL_SURFACE ( 'NONE', #2029, 27.00000000000000355 ) ;
#4727=EDGE_CURVE ( 'NONE', #533, #5515, #8168, .T. ) ;
#4729=CARTESIAN_POINT ( 'NONE',  ( 8.149445629999579666, 99.50000000000002842, 20.33980848884064230 ) ) ;
#4730=VERTEX_POINT ( 'NONE', #9816 ) ;
#4732=VERTEX_POINT ( 'NONE', #2651 ) ;
#4733=CARTESIAN_POINT ( 'NONE',  ( -19.39806930854668465, 2.349999998907525534, 19.39806930854667755 ) ) ;
#4734=CARTESIAN_POINT ( 'NONE',  ( 4.135809822336132591, 99.49999999999998579, -24.70305975188825443 ) ) ;
#4735=CARTESIAN_POINT ( 'NONE',  ( 0.000000000000000000, 100.0000000000000000, 0.000000000000000000 ) ) ;
#4737=CARTESIAN_POINT ( 'NONE',  ( 5.825495487346713297, 99.50000000000000000, 20.69456627699299744 ) ) ;
#4738=FACE_OUTER_BOUND ( 'NONE', #9365, .T. ) ;
#4739=CARTESIAN_POINT ( 'NONE',  ( 4.472992770554171216, 99.49999999999998579, -21.83386288566719458 ) ) ;
#4743=CARTESIAN_POINT ( 'NONE',  ( 4.640952353770416927, 99.50000000000000000, -24.17064508475253604 ) ) ;
#4751=CARTESIAN_POINT ( 'NONE',  ( -22.33529725360453000, 99.49999999999997158, -10.20112572733487255 ) ) ;
#4752=CARTESIAN_POINT ( 'NONE',  ( -15.07178375341841381, 99.50000000000000000, 16.66969090848992607 ) ) ;
#4753=CARTESIAN_POINT ( 'NONE',  ( 27.43301270000000258, 5.149999998907525800, 0.000000000000000000 ) ) ;
#4754=ORIENTED_EDGE ( 'NONE', *, *, #7781, .F. ) ;
#4756=CARTESIAN_POINT ( 'NONE',  ( 3.222930479149370253, 99.99999999999995737, -22.15251218086615381 ) ) ;
#4758=CARTESIAN_POINT ( 'NONE',  ( -20.89948324804827706, 99.50000000000001421, -10.26098411820691858 ) ) ;
#4759=CARTESIAN_POINT ( 'NONE',  ( -11.18376618407358336, 1.149999997815050357, 26.99999999999999645 ) ) ;
#4761=CARTESIAN_POINT ( 'NONE',  ( -15.11748654497029953, 99.49999999999998579, 15.76872032455190897 ) ) ;
#4762=CARTESIAN_POINT ( 'NONE',  ( 21.82251602564102910, 99.50000000000000000, -0.5181290064102563875 ) ) ;
#4763=CARTESIAN_POINT ( 'NONE',  ( 3.277744210708366079, 100.0000000000000142, -23.71256836663369327 ) ) ;
#4764=B_SPLINE_SURFACE_WITH_KNOTS ( 'NONE', 3, 1, ( 
 ( #9793, #1740 ),
 ( #7340, #918 ),
 ( #2632, #7243 ),
 ( #1786, #7195 ),
 ( #6465, #4937 ),
 ( #4111, #23 ),
 ( #6414, #3363 ),
 ( #3274, #3226 ),
 ( #8770, #9603 ),
 ( #7293, #132 ),
 ( #8135, #6556 ),
 ( #2436, #9747 ),
 ( #81, #2584 ),
 ( #6511, #5919 ),
 ( #4251, #5235 ) ),
 .UNSPECIFIED., .F., .F., .F.,
 ( 4, 1, 1, 1, 1, 1, 1, 1, 1, 1, 1, 1, 4 ),
 ( 2, 2 ),
 ( 0.000000000000000000, 0.08595325681623211533, 0.1695367914770939399, 0.2510169726856145700, 0.3324720360531058239, 0.4139176782331075444, 0.4946662699496591764, 0.5765962148649595997, 0.6610575120797289594, 0.7465372922784411225, 0.8302848992160567487, 0.9144215288650135998, 1.000000000000000000 ),
 ( 0.000000000000000000, 1.000000000000000000 ),
 .UNSPECIFIED. ) ;
#4765=CARTESIAN_POINT ( 'NONE',  ( -22.69253165798458127, 100.0000000000000142, -10.28928739654909563 ) ) ;
#4767=CARTESIAN_POINT ( 'NONE',  ( -21.79396932678589849, 99.50000000000000000, -9.306975108219608828 ) ) ;
#4768=ORIENTED_EDGE ( 'NONE', *, *, #4103, .T. ) ;
#4770=ORIENTED_EDGE ( 'NONE', *, *, #6044, .F. ) ;
#4772=CARTESIAN_POINT ( 'NONE',  ( -27.43301270000000969, 1.599999998907525534, 11.36312591709335429 ) ) ;
#4774=CARTESIAN_POINT ( 'NONE',  ( -27.00000000000000355, 3.550000000000000266, -11.18376618407357093 ) ) ;
#4775=CARTESIAN_POINT ( 'NONE',  ( -20.63200021313574695, 99.50000000000000000, -10.19493994959453431 ) ) ;
#4776=ORIENTED_EDGE ( 'NONE', *, *, #6072, .T. ) ;
#4777=AXIS2_PLACEMENT_3D ( 'NONE', #7461, #6578, #9678 ) ;
#4778=CARTESIAN_POINT ( 'NONE',  ( 8.467217662126737210, 100.0000000000000142, 20.02246181083229004 ) ) ;
#4779=AXIS2_PLACEMENT_3D ( 'NONE', #5030, #6699, #9068 ) ;
#4781=ORIENTED_EDGE ( 'NONE', *, *, #2496, .F. ) ;
#4782=CARTESIAN_POINT ( 'NONE',  ( 11.36312591709336139, 1.199999998907525178, -27.43301270000000258 ) ) ;
#4783=CARTESIAN_POINT ( 'NONE',  ( -27.00000000000000355, 2.000000000000000000, -3.306546357697854128E-15 ) ) ;
#4784=EDGE_CURVE ( 'NONE', #3764, #1470, #1077, .T. ) ;
#4785=DIRECTION ( 'NONE',  ( 0.000000000000000000, 0.000000000000000000, -1.000000000000000000 ) ) ;
#4788=CARTESIAN_POINT ( 'NONE',  ( -16.87593989452418697, 99.99999999999998579, 15.58794934546231126 ) ) ;
#4789=CARTESIAN_POINT ( 'NONE',  ( 27.00000000000000355, 5.399999997815051245, 0.000000000000000000 ) ) ;
#4793=DIRECTION ( 'NONE',  ( -0.000000000000000000, 1.000000000000000000, -0.000000000000000000 ) ) ;
#4794=CARTESIAN_POINT ( 'NONE',  ( -21.93524539549613550, 99.49999999999998579, -11.03420246938663318 ) ) ;
#4801=VECTOR ( 'NONE', #7398, 1000.000000000000000 ) ;
#4806=LINE ( 'NONE', #10363, #3628 ) ;
#4807=CARTESIAN_POINT ( 'NONE',  ( -11.36312591709335962, 4.599999998907525978, -27.43301270000000258 ) ) ;
#4808=ADVANCED_FACE ( 'NONE', ( #4427 ), #9292, .T. ) ;
#4811=CARTESIAN_POINT ( 'NONE',  ( 3.403200340195960738, 99.99999999999998579, -22.39827506699316118 ) ) ;
#4814=CARTESIAN_POINT ( 'NONE',  ( 19.09188309203678102, 2.099999997815050090, 19.09188309203678813 ) ) ;
#4815=B_SPLINE_CURVE_WITH_KNOTS ( 'NONE', 3,
 ( #4276, #2705, #5997, #7839, #1290, #4592, #6886, #9189, #7783, #10083, #2185, #6102, #2863, #4428, #5440, #2008, #9235, #8575, #3757 ),
 .UNSPECIFIED., .F., .F.,
 ( 4, 1, 1, 1, 1, 1, 1, 1, 1, 1, 1, 1, 1, 1, 1, 1, 4 ),
 ( 0.000000000000000000, 0.06358429906668214282, 0.1250797439647324816, 0.1854075229911844314, 0.2454523280917267347, 0.3052969617611028252, 0.3655926515411210831, 0.4275661794825392770, 0.4916205250740160460, 0.5555554127340263104, 0.6185525978810689773, 0.6803322039413655098, 0.7423868736098769849, 0.8044290668430417179, 0.8676072479036442964, 0.9329923078238739897, 1.000000000000000000 ),
 .UNSPECIFIED. ) ;
#4816=CARTESIAN_POINT ( 'NONE',  ( -20.63200021313574695, 99.50000000000000000, -10.19493994959453431 ) ) ;
#4817=CARTESIAN_POINT ( 'NONE',  ( 3.597125852879613728, 99.49999999999998579, -24.22990373345680126 ) ) ;
#4818=CARTESIAN_POINT ( 'NONE',  ( 3.356341388373609291, 100.0000000000000142, -21.61643044175963979 ) ) ;
#4819=DIRECTION ( 'NONE',  ( 0.9985355274883277454, 0.000000000000000000, -0.05409991075415103434 ) ) ;
#4820=VECTOR ( 'NONE', #265, 1000.000000000000000 ) ;
#4822=CARTESIAN_POINT ( 'NONE',  ( -20.77412980915959650, 99.49999999999997158, -9.759484723497815040 ) ) ;
#4823=ORIENTED_EDGE ( 'NONE', *, *, #2386, .F. ) ;
#4825=CARTESIAN_POINT ( 'NONE',  ( 27.43301269999999548, 4.999999998907525445, 11.36312591709337738 ) ) ;
#4826=CARTESIAN_POINT ( 'NONE',  ( -16.25490828497592588, 99.49999999999998579, 14.91257814242970348 ) ) ;
#4827=CARTESIAN_POINT ( 'NONE',  ( -19.09188309203678813, 4.500000000000000888, 19.09188309203678457 ) ) ;
#4828=VECTOR ( 'NONE', #2696, 1000.000000000000000 ) ;
#4829=CARTESIAN_POINT ( 'NONE',  ( 2.874264611687397331, 99.50000000000001421, -22.24889838548798693 ) ) ;
#4830=VERTEX_POINT ( 'NONE', #4373 ) ;
#4831=( NAMED_UNIT ( * ) PLANE_ANGLE_UNIT ( ) SI_UNIT ( $, .RADIAN. ) );
#4832=CARTESIAN_POINT ( 'NONE',  ( 11.18376618407357626, 2.049999997815050268, 27.00000000000000000 ) ) ;
#4834=CARTESIAN_POINT ( 'NONE',  ( 4.871887406949175769, 99.49999999999995737, -23.77896509604281405 ) ) ;
#4836=CARTESIAN_POINT ( 'NONE',  ( -27.43301270000000258, 3.849999998907525534, -3.359575119402369376E-15 ) ) ;
#4838=DIRECTION ( 'NONE',  ( -0.000000000000000000, -1.000000000000000000, -0.000000000000000000 ) ) ;
#4840=PLANE ( 'NONE',  #5882 ) ;
#4841=CARTESIAN_POINT ( 'NONE',  ( 19.09188309203678813, 1.700000000000000178, -19.09188309203678813 ) ) ;
#4842=CARTESIAN_POINT ( 'NONE',  ( 8.540544597724410991, 100.0000000000000000, 19.98924338346217766 ) ) ;
#4843=ORIENTED_EDGE ( 'NONE', *, *, #2909, .T. ) ;
#4844=EDGE_CURVE ( 'NONE', #9400, #8029, #2810, .T. ) ;
#4847=CARTESIAN_POINT ( 'NONE',  ( 4.358720771404392735, 100.0000000000000000, -21.20742720589606378 ) ) ;
#4848=CARTESIAN_POINT ( 'NONE',  ( -15.72775836928289017, 99.50000000000000000, 17.03252426573849476 ) ) ;
#4849=CARTESIAN_POINT ( 'NONE',  ( 9.778118981323553172, 99.49999999999998579, 20.11889122584574352 ) ) ;
#4851=B_SPLINE_SURFACE_WITH_KNOTS ( 'NONE', 3, 1, ( 
 ( #3268, #1645 ),
 ( #9599, #6461 ),
 ( #3360, #2535 ),
 ( #4932, #7979 ),
 ( #6359, #4888 ),
 ( #2430, #8131 ),
 ( #5678, #3175 ),
 ( #8084, #1692 ),
 ( #9553, #6409 ),
 ( #9506, #913 ),
 ( #7138, #4105 ),
 ( #7289, #129 ),
 ( #3316, #4153 ),
 ( #7336, #2331 ),
 ( #5528, #8721 ),
 ( #1539, #812 ),
 ( #4734, #10343 ),
 ( #4006, #7190 ),
 ( #19, #5626 ) ),
 .UNSPECIFIED., .F., .F., .F.,
 ( 4, 1, 1, 1, 1, 1, 1, 1, 1, 1, 1, 1, 1, 1, 1, 1, 4 ),
 ( 2, 2 ),
 ( 0.000000000000000000, 0.08029080299619884009, 0.1602734547033792534, 0.2412010114815648643, 0.3246404098231062685, 0.3670482715230247162, 0.4085690013065461645, 0.4496707568484641926, 0.4905395156191099670, 0.5313644394553277417, 0.5726744073239632415, 0.6138178896263115636, 0.6555018086025313773, 0.7394546411270094266, 0.8240219501092651555, 0.9101625766452680066, 1.000000000000000000 ),
 ( 0.000000000000000000, 1.000000000000000000 ),
 .UNSPECIFIED. ) ;
#4853=DIRECTION ( 'NONE',  ( 0.000000000000000000, -0.000000000000000000, 1.000000000000000000 ) ) ;
#4854=ADVANCED_FACE ( 'NONE', ( #6099 ), #10293, .T. ) ;
#4858=CARTESIAN_POINT ( 'NONE',  ( 11.18376618407357093, 3.149999997815050801, -27.00000000000000355 ) ) ;
#4859=CARTESIAN_POINT ( 'NONE',  ( 8.901217755223779449, 100.0000000000000426, 19.92336871027421097 ) ) ;
#4860=ORIENTED_EDGE ( 'NONE', *, *, #7145, .F. ) ;
#4861=ADVANCED_FACE ( 'NONE', ( #4738 ), #2334, .T. ) ;
#4863=CARTESIAN_POINT ( 'NONE',  ( 3.282077632710153292, 99.50000000000000000, -23.74569985055724786 ) ) ;
#4865=ADVANCED_FACE ( 'NONE', ( #8724 ), #4689, .T. ) ;
#4866=CARTESIAN_POINT ( 'NONE',  ( -20.70854316912038229, 99.50000000000001421, -10.95957977981033515 ) ) ;
#4867=CARTESIAN_POINT ( 'NONE',  ( 19.09188309203678813, 2.299999997815050712, -19.09188309203678813 ) ) ;
#4869=EDGE_CURVE ( 'NONE', #1454, #1485, #1436, .T. ) ;
#4870=DIRECTION ( 'NONE',  ( 1.000000000000000000, 0.000000000000000000, 0.000000000000000000 ) ) ;
#4874=CARTESIAN_POINT ( 'NONE',  ( 9.526533506306627430, 100.0000000000000000, 21.03094362668609207 ) ) ;
#4875=ORIENTED_EDGE ( 'NONE', *, *, #2754, .F. ) ;
#4877=CARTESIAN_POINT ( 'NONE',  ( 11.36312591709336139, 2.099999998907525089, -27.43301270000000258 ) ) ;
#4879=CARTESIAN_POINT ( 'NONE',  ( -4.959819536546781389E-15, 3.799999999999999822, 27.00000000000000355 ) ) ;
#4880=CARTESIAN_POINT ( 'NONE',  ( -21.16695614262292580, 100.0000000000000000, -11.33496398805607441 ) ) ;
#4881=VECTOR ( 'NONE', #6695, 1000.000000000000000 ) ;
#4883=ADVANCED_FACE ( 'NONE', ( #4059 ), #4764, .T. ) ;
#4884=DIRECTION ( 'NONE',  ( -0.000000000000000000, 1.000000000000000000, -0.000000000000000000 ) ) ;
#4885=CARTESIAN_POINT ( 'NONE',  ( -21.03403678956047074, 99.50000000000001421, -10.80451401317004922 ) ) ;
#4886=CARTESIAN_POINT ( 'NONE',  ( -20.72805389903318130, 99.50000000000000000, -9.848585782927868237 ) ) ;
#4887=CARTESIAN_POINT ( 'NONE',  ( -11.36312591709337561, 3.199999998907525178, 27.43301269999999548 ) ) ;
#4888=CARTESIAN_POINT ( 'NONE',  ( 3.097283534322414766, 100.0000000000000284, -24.18405864774921454 ) ) ;
#4889=VECTOR ( 'NONE', #5629, 1000.000000000000000 ) ;
#4890=DIRECTION ( 'NONE',  ( -0.05422338932609765960, 0.000000000000000000, -0.9985288298541962204 ) ) ;
#4892=CARTESIAN_POINT ( 'NONE',  ( -16.40919047799676989, 100.0000000000000000, 16.38364531277195013 ) ) ;
#4893=CARTESIAN_POINT ( 'NONE',  ( -16.67860655220511035, 99.49999999999998579, 15.23428378554110374 ) ) ;
#4894=CARTESIAN_POINT ( 'NONE',  ( 8.467217662126737210, 100.0000000000000142, 20.02246181083229004 ) ) ;
#4895=VECTOR ( 'NONE', #8027, 1000.000000000000000 ) ;
#4897=VERTEX_POINT ( 'NONE', #1107 ) ;
#4898=CARTESIAN_POINT ( 'NONE',  ( -22.28244091826395135, 99.99999999999997158, -10.68852969318427881 ) ) ;
#4901=CARTESIAN_POINT ( 'NONE',  ( -21.58460863908062066, 99.50000000000002842, -11.10356610083683648 ) ) ;
#4904=CARTESIAN_POINT ( 'NONE',  ( 8.091962505948220752, 99.49999999999995737, 20.48385654212622242 ) ) ;
#4906=CARTESIAN_POINT ( 'NONE',  ( -16.12578516900833137, 100.0000000000000142, 15.23469143358620492 ) ) ;
#4907=CARTESIAN_POINT ( 'NONE',  ( -19.09188309203678457, 4.299999999999999822, -19.09188309203678813 ) ) ;
#4908=ORIENTED_EDGE ( 'NONE', *, *, #9899, .F. ) ;
#4909=EDGE_CURVE ( 'NONE', #2567, #6863, #2840, .T. ) ;
#4910=CARTESIAN_POINT ( 'NONE',  ( -21.30928386698190025, 100.0000000000000000, -11.02857376369709996 ) ) ;
#4912=CARTESIAN_POINT ( 'NONE',  ( 3.986298408513477387, 100.0000000000000568, -22.53092616755505162 ) ) ;
#4913=CARTESIAN_POINT ( 'NONE',  ( -27.00000000000000355, 0.9999999978150503344, -3.306546357697854128E-15 ) ) ;
#4914=( BOUNDED_CURVE ( )  B_SPLINE_CURVE ( 2, ( #1711, #4126, #4907, #8102, #3335, #933, #148, #5286, #3672 ),
 .UNSPECIFIED., .F., .F. ) 
 B_SPLINE_CURVE_WITH_KNOTS ( ( 3, 2, 2, 2, 3 ),
 ( 0.7500000000000000000, 0.7678571428571429047, 0.7857142857142856984, 0.8035714285714286031, 0.8214285714285713969 ),
 .UNSPECIFIED. ) 
 CURVE ( )  GEOMETRIC_REPRESENTATION_ITEM ( )  RATIONAL_B_SPLINE_CURVE ( ( 1.000000000000000000, 0.9238795325112867385, 1.000000000000000000, 0.9238795325112867385, 1.000000000000000000, 0.9238795325112867385, 1.000000000000000000, 0.9238795325112867385, 1.000000000000000000 ) ) 
 REPRESENTATION_ITEM ( '' )  );
#4915=CARTESIAN_POINT ( 'NONE',  ( 3.296462644833695776, 99.50000000000001421, -23.81854410834942115 ) ) ;
#4916=CARTESIAN_POINT ( 'NONE',  ( 3.198592217420132666, 100.0000000000000000, -21.96964977087737836 ) ) ;
#4917=DIRECTION ( 'NONE',  ( 0.000000000000000000, 3.537534599156363020E-12, -1.000000000000000000 ) ) ;
#4919=ORIENTED_EDGE ( 'NONE', *, *, #3469, .F. ) ;
#4920=EDGE_LOOP ( 'NONE', ( #4875, #6855, #543, #7414 ) ) ;
#4922=CARTESIAN_POINT ( 'NONE',  ( -15.07178375341841381, 99.50000000000000000, 16.66969090848992607 ) ) ;
#4923=CARTESIAN_POINT ( 'NONE',  ( -27.43301270000000258, 0.5999999989075250895, -11.36312591709336317 ) ) ;
#4924=CARTESIAN_POINT ( 'NONE',  ( 0.000000000000000000, 100.0000000000000000, 0.000000000000000000 ) ) ;
#4926=CARTESIAN_POINT ( 'NONE',  ( -16.35834224700816009, 99.99999999999995737, 16.43761959438736397 ) ) ;
#4927=CARTESIAN_POINT ( 'NONE',  ( 19.09188309203678813, 2.299999997815050712, -19.09188309203678813 ) ) ;
#4928=ORIENTED_EDGE ( 'NONE', *, *, #4537, .F. ) ;
#4929=EDGE_CURVE ( 'NONE', #2398, #6279, #9014, .T. ) ;
#4931=VECTOR ( 'NONE', #5712, 1000.000000000000000 ) ;
#4932=CARTESIAN_POINT ( 'NONE',  ( 3.024867170474271116, 99.49999999999995737, -24.05477125543085748 ) ) ;
#4933=ADVANCED_FACE ( 'NONE', ( #9167 ), #6926, .T. ) ;
#4937=CARTESIAN_POINT ( 'NONE',  ( -22.43208371148383762, 100.0000000000000000, -9.654966607469265938 ) ) ;
#4938=CARTESIAN_POINT ( 'NONE',  ( 8.231219904624582639, 100.0000000000000000, 20.21381436664452735 ) ) ;
#4940=ORIENTED_EDGE ( 'NONE', *, *, #143, .T. ) ;
#4942=CARTESIAN_POINT ( 'NONE',  ( 3.552835461024879127, 99.99999999999997158, -21.47801279722421697 ) ) ;
#4943=CARTESIAN_POINT ( 'NONE',  ( -14.89910828679519739, 99.99999999999997158, 16.44921749203638939 ) ) ;
#4946=CARTESIAN_POINT ( 'NONE',  ( 8.064245308217579122, 99.49999999999998579, 20.64099956338070641 ) ) ;
#4949=CARTESIAN_POINT ( 'NONE',  ( -22.28244091826395135, 100.0000000000000000, -10.68852969318427881 ) ) ;
#4950=CARTESIAN_POINT ( 'NONE',  ( 4.320351800798612807, 99.49999999999995737, -21.62386382141117736 ) ) ;
#4952=VECTOR ( 'NONE', #1800, 1000.000000000000000 ) ;
#4953=CARTESIAN_POINT ( 'NONE',  ( 3.977571997893210032, 99.50000000000000000, -24.70179182097838932 ) ) ;
#4954=CARTESIAN_POINT ( 'NONE',  ( 4.232447118646125439, 99.99999999999995737, -21.54138831197867887 ) ) ;
#4956=CARTESIAN_POINT ( 'NONE',  ( 27.00000000000000355, 4.649999997815049468, -11.18376618407356737 ) ) ;
#4965=CARTESIAN_POINT ( 'NONE',  ( 7.156925775808251622, 99.50000000000000000, 23.91622092442889524 ) ) ;
#4968=CARTESIAN_POINT ( 'NONE',  ( -11.18376618407358336, 3.750000000000000000, 26.99999999999999645 ) ) ;
#4969=CARTESIAN_POINT ( 'NONE',  ( 3.105863891863242632, 100.0000000000000142, -22.59672720503480292 ) ) ;
#4971=DIRECTION ( 'NONE',  ( 0.000000000000000000, -0.000000000000000000, 1.000000000000000000 ) ) ;
#4972=CARTESIAN_POINT ( 'NONE',  ( -20.95611194834973645, 99.99999999999997158, -10.07788454426966318 ) ) ;
#4973=EDGE_CURVE ( 'NONE', #2426, #2647, #9107, .T. ) ;
#4974=ORIENTED_EDGE ( 'NONE', *, *, #4419, .T. ) ;
#4975=CARTESIAN_POINT ( 'NONE',  ( -21.59614764830937972, 99.50000000000001421, -9.292069227195950631 ) ) ;
#4977=CARTESIAN_POINT ( 'NONE',  ( -15.56095293356939813, 99.50000000000001421, 15.23332223661997453 ) ) ;
#4978=CARTESIAN_POINT ( 'NONE',  ( -21.16695614262292580, 100.0000000000000000, -11.33496398805607441 ) ) ;
#4981=CARTESIAN_POINT ( 'NONE',  ( -22.69253165798458127, 99.50000000000001421, -10.28928739654909563 ) ) ;
#4982=CARTESIAN_POINT ( 'NONE',  ( -16.88522588321459494, 100.0000000000000284, 16.18266969485829421 ) ) ;
#4983=CARTESIAN_POINT ( 'NONE',  ( 4.599186066243659887, 100.0000000000000284, -24.59301055568561623 ) ) ;
#4984=EDGE_CURVE ( 'NONE', #7488, #7789, #2168, .T. ) ;
#4986=VERTEX_POINT ( 'NONE', #4677 ) ;
#4987=VERTEX_POINT ( 'NONE', #5360 ) ;
#4990=EDGE_CURVE ( 'NONE', #2804, #358, #1530, .T. ) ;
#4991=CARTESIAN_POINT ( 'NONE',  ( 9.600410285814406919, 99.49999999999998579, 19.87914582625927196 ) ) ;
#4993=DIRECTION ( 'NONE',  ( 1.320207234900709352E-11, 1.000000000000000000, 2.368819407112974206E-12 ) ) ;
#4998=CARTESIAN_POINT ( 'NONE',  ( 3.689266881520847807, 99.50000000000000000, -22.97735580002706968 ) ) ;
#4999=CARTESIAN_POINT ( 'NONE',  ( 3.949943451936506644, 99.50000000000000000, -21.41482314084395711 ) ) ;
#5001=CARTESIAN_POINT ( 'NONE',  ( 3.403200340195960738, 100.0000000000000142, -22.39827506699316118 ) ) ;
#5002=CARTESIAN_POINT ( 'NONE',  ( 19.09188309203678102, 2.899999997815050357, 19.09188309203678813 ) ) ;
#5003=CARTESIAN_POINT ( 'NONE',  ( -21.13504512532655610, 99.50000000000000000, -11.31853095674525100 ) ) ;
#5004=CARTESIAN_POINT ( 'NONE',  ( -21.04016555629948826, 100.0000000000000142, -9.929603401003973318 ) ) ;
#5005=DIRECTION ( 'NONE',  ( 0.000000000000000000, 0.000000000000000000, -1.000000000000000000 ) ) ;
#5006=CARTESIAN_POINT ( 'NONE',  ( -21.65488089977124275, 99.49999999999997158, -11.10326233039539723 ) ) ;
#5009=ORIENTED_EDGE ( 'NONE', *, *, #10100, .F. ) ;
#5010=VECTOR ( 'NONE', #1721, 999.9999999999998863 ) ;
#5011=ORIENTED_EDGE ( 'NONE', *, *, #9313, .T. ) ;
#5014=CARTESIAN_POINT ( 'NONE',  ( -15.07178375341841381, 99.99999999999998579, 15.16157792772069790 ) ) ;
#5015=CARTESIAN_POINT ( 'NONE',  ( 9.820792995160308791, 99.50000000000000000, 20.21220011423140761 ) ) ;
#5016=ADVANCED_FACE ( 'NONE', ( #10283 ), #3565, .F. ) ;
#5017=CARTESIAN_POINT ( 'NONE',  ( 27.43301270000000258, 4.299999998907525267, -11.36312591709336139 ) ) ;
#5018=CARTESIAN_POINT ( 'NONE',  ( 27.43301270000000258, 0.3499999989075252005, 0.000000000000000000 ) ) ;
#5020=DIRECTION ( 'NONE',  ( -0.8547548816071318667, 0.000000000000000000, 0.5190318799156541374 ) ) ;
#5021=CARTESIAN_POINT ( 'NONE',  ( 26.99999999999999645, 2.149999997815051245, 11.18376618407358691 ) ) ;
#5023=CARTESIAN_POINT ( 'NONE',  ( 7.809833820264425519, 99.49999999999995737, 20.29999375863051370 ) ) ;
#5024=CARTESIAN_POINT ( 'NONE',  ( 3.701176614148623756, 100.0000000000000000, -24.64875008328975170 ) ) ;
#5025=CARTESIAN_POINT ( 'NONE',  ( -15.32348647777738826, 99.50000000000000000, 15.39505148541300450 ) ) ;
#5026=CARTESIAN_POINT ( 'NONE',  ( -16.12311789350856017, 99.50000000000000000, 14.86696503675854686 ) ) ;
#5028=EDGE_CURVE ( 'NONE', #9655, #7619, #5278, .T. ) ;
#5029=CARTESIAN_POINT ( 'NONE',  ( 9.575551604960836016, 99.50000000000001421, 20.57049984249936969 ) ) ;
#5030=CARTESIAN_POINT ( 'NONE',  ( 27.43301270000000258, 0.2999999989075251561, 0.000000000000000000 ) ) ;
#5031=ORIENTED_EDGE ( 'NONE', *, *, #1028, .T. ) ;
#5033=EDGE_LOOP ( 'NONE', ( #698, #8540, #2062, #9445, #2288, #2533, #5548, #4021, #6607, #3062, #5828, #4781 ) ) ;
#5034=CARTESIAN_POINT ( 'NONE',  ( -22.10910773081910818, 100.0000000000000142, -11.33820747227609793 ) ) ;
#5035=CARTESIAN_POINT ( 'NONE',  ( 3.497829868842083023, 99.99999999999997158, -21.50512556757917793 ) ) ;
#5036=DIRECTION ( 'NONE',  ( -0.1697592580069431922, 0.000000000000000000, 0.9854855627156250408 ) ) ;
#5037=CARTESIAN_POINT ( 'NONE',  ( -21.30928386698190025, 99.50000000000000000, -11.02857376369709996 ) ) ;
#5041=LINE ( 'NONE', #7446, #279 ) ;
#5044=EDGE_LOOP ( 'NONE', ( #9148, #2222, #7965, #8556 ) ) ;
#5045=CARTESIAN_POINT ( 'NONE',  ( -15.31787750341841559, 99.50000000000000000, 16.43551622900274722 ) ) ;
#5046=CARTESIAN_POINT ( 'NONE',  ( 11.36312591709336139, 1.299999998907525267, -27.43301270000000258 ) ) ;
#5047=LINE ( 'NONE', #8249, #1548 ) ;
#5048=EDGE_CURVE ( 'NONE', #9797, #358, #6766, .T. ) ;
#5050=CARTESIAN_POINT ( 'NONE',  ( 4.187832255138415505, 99.50000000000001421, -21.50835573230103037 ) ) ;
#5051=ORIENTED_EDGE ( 'NONE', *, *, #5633, .F. ) ;
#5052=CARTESIAN_POINT ( 'NONE',  ( 9.897596448871711416, 99.49999999999998579, 20.85734708541456328 ) ) ;
#5053=CARTESIAN_POINT ( 'NONE',  ( 27.00000000000000355, 5.449999997815051067, -11.18376618407356737 ) ) ;
#5054=PLANE ( 'NONE',  #6852 ) ;
#5055=AXIS2_PLACEMENT_3D ( 'NONE', #9842, #4154, #9744 ) ;
#5057=DIRECTION ( 'NONE',  ( -0.9567206510497618943, 0.000000000000000000, 0.2910078965507976179 ) ) ;
#5058=CARTESIAN_POINT ( 'NONE',  ( 3.638175769014108774, 99.99999999999998579, -21.10017783766535970 ) ) ;
#5060=ORIENTED_EDGE ( 'NONE', *, *, #9459, .T. ) ;
#5063=CARTESIAN_POINT ( 'NONE',  ( -15.10737684033046335, 99.50000000000000000, 15.12848924955281049 ) ) ;
#5064=CARTESIAN_POINT ( 'NONE',  ( 2.928963527206765338, 99.49999999999997158, -23.52685633767685758 ) ) ;
#5065=CARTESIAN_POINT ( 'NONE',  ( -19.39806930854667755, 1.349999998907525534, -19.39806930854668110 ) ) ;
#5066=DIRECTION ( 'NONE',  ( -0.2907782774943305504, 0.000000000000000000, -0.9567904646982169359 ) ) ;
#5067=FACE_OUTER_BOUND ( 'NONE', #9059, .T. ) ;
#5068=DIRECTION ( 'NONE',  ( 0.000000000000000000, 0.000000000000000000, 1.000000000000000000 ) ) ;
#5070=ORIENTED_EDGE ( 'NONE', *, *, #2658, .T. ) ;
#5071=CARTESIAN_POINT ( 'NONE',  ( 7.771508748547515388, 99.50000000000001421, 20.40818475981234315 ) ) ;
#5073=CARTESIAN_POINT ( 'NONE',  ( 9.526533506306627430, 99.50000000000000000, 21.03094362668609207 ) ) ;
#5074=CARTESIAN_POINT ( 'NONE',  ( 27.00000000000000355, 4.800000000000000711, 0.000000000000000000 ) ) ;
#5076=CARTESIAN_POINT ( 'NONE',  ( -16.36470918167357169, 100.0000000000000000, 16.79054296464299867 ) ) ;
#5077=CARTESIAN_POINT ( 'NONE',  ( 9.547662139763570366, 99.99999999999991473, 20.94662037603165672 ) ) ;
#5078=CARTESIAN_POINT ( 'NONE',  ( -15.07178375341841559, 99.50000000000001421, 15.16157792772069968 ) ) ;
#5080=CARTESIAN_POINT ( 'NONE',  ( -16.24524625128438515, 100.0000000000000284, 16.53274063862002308 ) ) ;
#5082=ORIENTED_EDGE ( 'NONE', *, *, #4784, .F. ) ;
#5083=EDGE_CURVE ( 'NONE', #5876, #2748, #6416, .T. ) ;
#5084=CARTESIAN_POINT ( 'NONE',  ( -22.35642768247353729, 99.49999999999995737, -10.34293228154892752 ) ) ;
#5086=AXIS2_PLACEMENT_3D ( 'NONE', #7612, #507, #8459 ) ;
#5089=B_SPLINE_CURVE_WITH_KNOTS ( 'NONE', 3,
 ( #5986, #8506, #2176, #390, #1391, #3746, #5375, #2908, #441, #8564, #6093, #10017, #4364, #2970, #9227, #9285, #1336, #1281, #2118 ),
 .UNSPECIFIED., .F., .F.,
 ( 4, 1, 1, 1, 1, 1, 1, 1, 1, 1, 1, 1, 1, 1, 1, 1, 4 ),
 ( 0.000000000000000000, 0.07315862907712983310, 0.1430989967074559055, 0.2105333571262071879, 0.2759142635903734653, 0.3397077151413689933, 0.4013946392018796772, 0.4627937533375801049, 0.5237250720276656057, 0.5836284080752294212, 0.6425725562371763511, 0.7010486867616194662, 0.7591976973140022178, 0.8177727706511607186, 0.8769111530050104353, 0.9375229829315941954, 1.000000000000000000 ),
 .UNSPECIFIED. ) ;
#5091=DIRECTION ( 'NONE',  ( 0.9569724629708533659, 0.000000000000000000, -0.2901787468363226097 ) ) ;
#5092=DIRECTION ( 'NONE',  ( -0.000000000000000000, 1.000000000000000000, -0.000000000000000000 ) ) ;
#5093=VECTOR ( 'NONE', #6756, 1000.000000000000000 ) ;
#5094=CARTESIAN_POINT ( 'NONE',  ( 0.000000000000000000, 100.0000000000000000, 0.000000000000000000 ) ) ;
#5096=LINE ( 'NONE', #1074, #5223 ) ;
#5097=CARTESIAN_POINT ( 'NONE',  ( -11.36312591709335962, 3.799999998907525711, -27.43301270000000258 ) ) ;
#5098=CARTESIAN_POINT ( 'NONE',  ( 3.061616997868383043E-15, 97.50000000000000000, 25.00000000000000000 ) ) ;
#5100=CARTESIAN_POINT ( 'NONE',  ( 7.753999887479250397, 99.50000000000000000, 20.97676509141502166 ) ) ;
#5101=CARTESIAN_POINT ( 'NONE',  ( 3.207057600658871355, 99.50000000000000000, -22.07913334414698880 ) ) ;
#5102=CARTESIAN_POINT ( 'NONE',  ( 11.18376618407356915, 5.549999997815052488, -27.00000000000000355 ) ) ;
#5103=EDGE_CURVE ( 'NONE', #7275, #4897, #7677, .T. ) ;
#5108=CARTESIAN_POINT ( 'NONE',  ( -22.05902956123343017, 99.50000000000000000, -10.96257574645357558 ) ) ;
#5110=DIRECTION ( 'NONE',  ( 0.000000000000000000, 0.000000000000000000, 1.000000000000000000 ) ) ;
#5116=DIRECTION ( 'NONE',  ( 0.9567904646982170469, 0.000000000000000000, -0.2907782774943306059 ) ) ;
#5117=LINE ( 'NONE', #3396, #3889 ) ;
#5118=CARTESIAN_POINT ( 'NONE',  ( -27.43301270000000258, 3.049999998907525267, -3.359575119402369376E-15 ) ) ;
#5119=CARTESIAN_POINT ( 'NONE',  ( -19.39806930854667755, 0.6499999989075252449, -19.39806930854668110 ) ) ;
#5120=AXIS2_PLACEMENT_3D ( 'NONE', #3506, #6692, #7528 ) ;
#5121=DIRECTION ( 'NONE',  ( -0.000000000000000000, 1.000000000000000000, -0.000000000000000000 ) ) ;
#5123=CARTESIAN_POINT ( 'NONE',  ( 4.693123912524271191, 100.0000000000000284, -24.12247278045041554 ) ) ;
#5124=CARTESIAN_POINT ( 'NONE',  ( 7.978247738654171251, 100.0000000000000000, 20.00924965157036794 ) ) ;
#5125=CARTESIAN_POINT ( 'NONE',  ( 8.429066232339796017, 99.50000000000000000, 19.67794530653910101 ) ) ;
#5128=CARTESIAN_POINT ( 'NONE',  ( -15.69732130854469432, 99.50000000000001421, 15.19348709373450035 ) ) ;
#5129=FILL_AREA_STYLE ('',( #1056 ) ) ;
#5130=CARTESIAN_POINT ( 'NONE',  ( 11.18376618407357626, 4.650000000000000355, 27.00000000000000000 ) ) ;
#5132=CARTESIAN_POINT ( 'NONE',  ( 9.526713201929464248, 99.99999999999994316, 20.38668308130821671 ) ) ;
#5133=LINE ( 'NONE', #7591, #2771 ) ;
#5134=ORIENTED_EDGE ( 'NONE', *, *, #3091, .F. ) ;
#5135=CARTESIAN_POINT ( 'NONE',  ( -16.30427144417478402, 99.49999999999998579, 16.48895498912494517 ) ) ;
#5137=VERTEX_POINT ( 'NONE', #577 ) ;
#5138=CARTESIAN_POINT ( 'NONE',  ( -22.33589105551819642, 99.50000000000002842, -11.18147695539509812 ) ) ;
#5139=LINE ( 'NONE', #4359, #2965 ) ;
#5140=CARTESIAN_POINT ( 'NONE',  ( -11.18376618407358336, 5.149999997815050357, 26.99999999999999645 ) ) ;
#5141=CARTESIAN_POINT ( 'NONE',  ( -15.10687288066601930, 99.99999999999998579, 15.84109048427130517 ) ) ;
#5142=EDGE_CURVE ( 'NONE', #2986, #1777, #3426, .T. ) ;
#5144=ORIENTED_EDGE ( 'NONE', *, *, #9143, .F. ) ;
#5145=FACE_OUTER_BOUND ( 'NONE', #2687, .T. ) ;
#5147=CARTESIAN_POINT ( 'NONE',  ( -22.05902956123343017, 100.0000000000000000, -10.96257574645357558 ) ) ;
#5148=DIRECTION ( 'NONE',  ( -0.000000000000000000, 1.000000000000000000, -0.000000000000000000 ) ) ;
#5149=ORIENTED_EDGE ( 'NONE', *, *, #7717, .T. ) ;
#5150=FACE_OUTER_BOUND ( 'NONE', #3749, .T. ) ;
#5151=CARTESIAN_POINT ( 'NONE',  ( 19.39806930854668110, 5.249999998907525445, -19.39806930854668110 ) ) ;
#5153=CARTESIAN_POINT ( 'NONE',  ( 3.824506687597884369, 99.50000000000002842, -24.68145443631992109 ) ) ;
#5154=CARTESIAN_POINT ( 'NONE',  ( 7.771508748547515388, 99.99999999999995737, 20.40818475981234315 ) ) ;
#5155=ORIENTED_EDGE ( 'NONE', *, *, #5638, .F. ) ;
#5156=CARTESIAN_POINT ( 'NONE',  ( 9.692323321704657602, 99.50000000000001421, 21.58969587442354410 ) ) ;
#5157=CARTESIAN_POINT ( 'NONE',  ( -27.00000000000000355, 2.549999997815051156, -11.18376618407357093 ) ) ;
#5159=CARTESIAN_POINT ( 'NONE',  ( -21.18972881998075763, 99.99999999999998579, -9.781869222470191971 ) ) ;
#5160=CARTESIAN_POINT ( 'NONE',  ( 0.000000000000000000, 100.0000000000000000, 0.000000000000000000 ) ) ;
#5161=ORIENTED_EDGE ( 'NONE', *, *, #1641, .F. ) ;
#5162=CARTESIAN_POINT ( 'NONE',  ( 2.843562173796539749, 100.0000000000000142, -21.91597968833000110 ) ) ;
#5166=EDGE_CURVE ( 'NONE', #2280, #8581, #6763, .T. ) ;
#5168=CARTESIAN_POINT ( 'NONE',  ( -14.83363727892122519, 99.50000000000001421, 15.50654517199034466 ) ) ;
#5169=CARTESIAN_POINT ( 'NONE',  ( 2.940192896829773250, 100.0000000000000142, -23.44521981770616037 ) ) ;
#5170=CARTESIAN_POINT ( 'NONE',  ( -27.43301270000000258, 3.849999998907525534, -3.359575119402369376E-15 ) ) ;
#5171=CARTESIAN_POINT ( 'NONE',  ( -4.959819536546781389E-15, 0.6000000000000000888, 27.00000000000000355 ) ) ;
#5172=CARTESIAN_POINT ( 'NONE',  ( -16.25490828497592588, 99.99999999999998579, 14.91257814242970348 ) ) ;
#5173=DIRECTION ( 'NONE',  ( 0.000000000000000000, 0.000000000000000000, 1.000000000000000000 ) ) ;
#5175=( BOUNDED_CURVE ( )  B_SPLINE_CURVE ( 2, ( #6822, #6264, #6991, #3696, #8568, #10196, #1338, #7720, #9463 ),
 .UNSPECIFIED., .F., .F. ) 
 B_SPLINE_CURVE_WITH_KNOTS ( ( 3, 2, 2, 2, 3 ),
 ( 0.1071428571428571369, 0.1250000000000000000, 0.1428571428571428492, 0.1607142857142857262, 0.1785714285714285754 ),
 .UNSPECIFIED. ) 
 CURVE ( )  GEOMETRIC_REPRESENTATION_ITEM ( )  RATIONAL_B_SPLINE_CURVE ( ( 1.000000000000000000, 0.9238795325112867385, 1.000000000000000000, 0.9238795325112867385, 1.000000000000000000, 0.9238795325112867385, 1.000000000000000000, 0.9238795325112867385, 1.000000000000000000 ) ) 
 REPRESENTATION_ITEM ( '' )  );
#5176=CARTESIAN_POINT ( 'NONE',  ( -21.39817337045129619, 99.50000000000001421, -9.317726141196148504 ) ) ;
#5177=CARTESIAN_POINT ( 'NONE',  ( -21.56977948371741505, 99.49999999999995737, -11.44450812306045329 ) ) ;
#5178=EDGE_LOOP ( 'NONE', ( #9549, #2245, #8310, #6459 ) ) ;
#5179=FACE_BOUND ( 'NONE', #3402, .T. ) ;
#5183=B_SPLINE_CURVE_WITH_KNOTS ( 'NONE', 3,
 ( #4842, #3409, #4894, #1598, #2585, #3364, #4938, #9795, #6512, #5583, #9654, #8771, #176, #8089, #1741, #919, #8822, #8037, #9701 ),
 .UNSPECIFIED., .F., .F.,
 ( 4, 1, 1, 1, 1, 1, 1, 1, 1, 1, 1, 1, 1, 1, 1, 1, 4 ),
 ( 0.000000000000000000, 0.06282509715607415002, 0.1231380613775250599, 0.1822388757841713336, 0.2396184841454026548, 0.2973605923678978580, 0.3541959668311244203, 0.4122907788200148582, 0.4717534157231769720, 0.5322282553174864095, 0.5926403291039165078, 0.6546871955647078911, 0.7179012776534754448, 0.7839155840457150415, 0.8527518695723632636, 0.9242989153657757972, 1.000000000000000000 ),
 .UNSPECIFIED. ) ;
#5185=CARTESIAN_POINT ( 'NONE',  ( 9.563602730896748838, 99.99999999999994316, 20.87184380654744587 ) ) ;
#5187=CARTESIAN_POINT ( 'NONE',  ( -21.31369174262763622, 99.99999999999997158, -9.710155485040722567 ) ) ;
#5189=CARTESIAN_POINT ( 'NONE',  ( -21.16695614262292580, 99.50000000000000000, -11.33496398805607441 ) ) ;
#5191=EDGE_LOOP ( 'NONE', ( #2888, #6195, #508, #2265 ) ) ;
#5193=CARTESIAN_POINT ( 'NONE',  ( 19.39806930854667399, 0.9499999989075252893, 19.39806930854668465 ) ) ;
#5195=CARTESIAN_POINT ( 'NONE',  ( -15.11611088805441661, 100.0000000000000000, 16.06180012866831319 ) ) ;
#5196=ORIENTED_EDGE ( 'NONE', *, *, #4019, .F. ) ;
#5198=CARTESIAN_POINT ( 'NONE',  ( -16.79604063091391097, 100.0000000000000000, 15.40463673182947701 ) ) ;
#5199=CARTESIAN_POINT ( 'NONE',  ( -15.07178375341841381, 100.0000000000000000, 16.66969090848992607 ) ) ;
#5201=CARTESIAN_POINT ( 'NONE',  ( 5.243816414761435674, 99.50000000000000000, -23.48558366465980995 ) ) ;
#5204=CARTESIAN_POINT ( 'NONE',  ( -16.65546786808457469, 99.99999999999998579, 16.57295196178722918 ) ) ;
#5205=ORIENTED_EDGE ( 'NONE', *, *, #9048, .T. ) ;
#5206=CARTESIAN_POINT ( 'NONE',  ( 1.679787559701184688E-15, 5.349999998907525089, -27.43301270000000258 ) ) ;
#5209=CARTESIAN_POINT ( 'NONE',  ( -16.63177974700816009, 99.50000000000000000, 16.59747536361813403 ) ) ;
#5211=VECTOR ( 'NONE', #6669, 1000.000000000000114 ) ;
#5213=CARTESIAN_POINT ( 'NONE',  ( -16.05932294508833280, 100.0000000000000000, 15.21084698918278555 ) ) ;
#5214=CARTESIAN_POINT ( 'NONE',  ( 19.39806930854667399, 2.649999998907525356, 19.39806930854668465 ) ) ;
#5215=ORIENTED_EDGE ( 'NONE', *, *, #3681, .T. ) ;
#5216=ADVANCED_FACE ( 'NONE', ( #1619 ), #2260, .T. ) ;
#5221=CARTESIAN_POINT ( 'NONE',  ( -11.36312591709335962, 2.899999998907525356, -27.43301270000000258 ) ) ;
#5223=VECTOR ( 'NONE', #8296, 1000.000000000000000 ) ;
#5224=ORIENTED_EDGE ( 'NONE', *, *, #5883, .F. ) ;
#5226=PLANE ( 'NONE',  #2637 ) ;
#5227=CARTESIAN_POINT ( 'NONE',  ( 8.393217272293057363, 100.0000000000000000, 19.69436072183531650 ) ) ;
#5228=CARTESIAN_POINT ( 'NONE',  ( -15.56095293356939813, 100.0000000000000142, 15.23332223661997453 ) ) ;
#5231=EDGE_LOOP ( 'NONE', ( #5196, #5149, #3519, #503 ) ) ;
#5233=CARTESIAN_POINT ( 'NONE',  ( -11.36312591709337383, 0.7999999989075252671, 27.43301269999999548 ) ) ;
#5234=CARTESIAN_POINT ( 'NONE',  ( -16.25490828497592588, 99.99999999999994316, 14.91257814242970348 ) ) ;
#5235=CARTESIAN_POINT ( 'NONE',  ( -22.57971655928959365, 100.0000000000000000, -10.84768434062017839 ) ) ;
#5236=B_SPLINE_CURVE_WITH_KNOTS ( 'NONE', 3,
 ( #9279, #656, #549, #3686, #5427, #2903, #6870, #1440, #1330, #5306, #3635 ),
 .UNSPECIFIED., .F., .F.,
 ( 4, 1, 1, 1, 1, 1, 1, 1, 4 ),
 ( 0.000000000000000000, 0.09809051273808343241, 0.1997563395654988194, 0.3058527769869914259, 0.4162847437678430240, 0.5377099880548563693, 0.6743560419832976827, 0.8289895874771281425, 1.000000000000000000 ),
 .UNSPECIFIED. ) ;
#5238=ORIENTED_EDGE ( 'NONE', *, *, #4397, .T. ) ;
#5240=FACE_OUTER_BOUND ( 'NONE', #6, .T. ) ;
#5241=ADVANCED_FACE ( 'NONE', ( #3294 ), #2342, .T. ) ;
#5243=VERTEX_POINT ( 'NONE', #9038 ) ;
#5244=EDGE_CURVE ( 'NONE', #7666, #5650, #9052, .T. ) ;
#5245=CARTESIAN_POINT ( 'NONE',  ( -22.33529725360453000, 99.99999999999994316, -10.20112572733487255 ) ) ;
#5246=FACE_OUTER_BOUND ( 'NONE', #1324, .T. ) ;
#5249=DIRECTION ( 'NONE',  ( 0.05376826219280737146, 0.000000000000000000, 0.9985534407235125975 ) ) ;
#5250=CARTESIAN_POINT ( 'NONE',  ( 4.850954546176396320, 99.49999999999998579, -24.43907202982397209 ) ) ;
#5254=CARTESIAN_POINT ( 'NONE',  ( -16.62994343074595349, 99.99999999999998579, 15.18287566599475191 ) ) ;
#5256=ORIENTED_EDGE ( 'NONE', *, *, #4784, .T. ) ;
#5257=CARTESIAN_POINT ( 'NONE',  ( 27.00000000000000355, 1.449999997815050401, -11.18376618407356915 ) ) ;
#5258=CARTESIAN_POINT ( 'NONE',  ( 27.43301270000000258, 2.799999998907525267, -11.36312591709336139 ) ) ;
#5261=CARTESIAN_POINT ( 'NONE',  ( 21.79306891025641235, 99.50000000000000000, -1.065004006410256387 ) ) ;
#5262=VECTOR ( 'NONE', #998, 1000.000000000000000 ) ;
#5263=ORIENTED_EDGE ( 'NONE', *, *, #6476, .T. ) ;
#5264=CARTESIAN_POINT ( 'NONE',  ( 9.820792995160308791, 99.50000000000000000, 20.21220011423140761 ) ) ;
#5265=CARTESIAN_POINT ( 'NONE',  ( 4.503533123526070270, 99.49999999999995737, -24.63026223303895890 ) ) ;
#5267=CARTESIAN_POINT ( 'NONE',  ( -16.52157078939288937, 99.49999999999998579, 16.20087177393598665 ) ) ;
#5269=ORIENTED_EDGE ( 'NONE', *, *, #9785, .T. ) ;
#5270=CARTESIAN_POINT ( 'NONE',  ( -16.56928979259283352, 100.0000000000000284, 16.65656195153832897 ) ) ;
#5271=CARTESIAN_POINT ( 'NONE',  ( 1.679787559701184688E-15, 0.5499999989075251561, -27.43301270000000258 ) ) ;
#5272=VERTEX_POINT ( 'NONE', #6779 ) ;
#5275=CARTESIAN_POINT ( 'NONE',  ( 9.114876806416853938, 99.49999999999998579, 19.97295714941878231 ) ) ;
#5276=FACE_OUTER_BOUND ( 'NONE', #7053, .T. ) ;
#5278=LINE ( 'NONE', #10095, #3119 ) ;
#5279=CARTESIAN_POINT ( 'NONE',  ( 27.43301270000000258, 1.949999998907525178, 0.000000000000000000 ) ) ;
#5281=PRODUCT_DEFINITION_CONTEXT ( 'detailed design', #3146, 'design' ) ;
#5282=EDGE_CURVE ( 'NONE', #3939, #834, #7562, .T. ) ;
#5283=CARTESIAN_POINT ( 'NONE',  ( -15.10737684033046335, 100.0000000000000000, 15.12848924955281049 ) ) ;
#5285=CARTESIAN_POINT ( 'NONE',  ( -27.00000000000001421, 4.249999997815050001, 11.18376618407356560 ) ) ;
#5286=CARTESIAN_POINT ( 'NONE',  ( -11.18376618407358336, 4.549999999999999822, 26.99999999999999645 ) ) ;
#5287=VECTOR ( 'NONE', #1384, 1000.000000000000000 ) ;
#5291=ORIENTED_EDGE ( 'NONE', *, *, #2238, .T. ) ;
#5292=CARTESIAN_POINT ( 'NONE',  ( 19.39806930854668110, 2.749999998907525001, -19.39806930854668110 ) ) ;
#5294=LINE ( 'NONE', #8607, #1068 ) ;
#5295=B_SPLINE_CURVE_WITH_KNOTS ( 'NONE', 3,
 ( #8224, #271, #3567, #5822, #6601, #6806, #9894, #6024, #2730, #9843, #1212, #4199, #5918, #9064, #4350 ),
 .UNSPECIFIED., .F., .F.,
 ( 4, 1, 1, 1, 1, 1, 1, 1, 1, 1, 1, 1, 4 ),
 ( 0.000000000000000000, 0.1166921615859537187, 0.2277195327244859735, 0.3361971884410420164, 0.4453256767247914527, 0.5018483577356800396, 0.5617326728321133666, 0.6243107931132723110, 0.6909729641497043273, 0.7615676753376537933, 0.8363829297815326136, 0.9156607463298391814, 0.9999999999999998890 ),
 .UNSPECIFIED. ) ;
#5296=CARTESIAN_POINT ( 'NONE',  ( 1.653273178848927064E-15, 1.800000000000000266, -27.00000000000000355 ) ) ;
#5298=CARTESIAN_POINT ( 'NONE',  ( 2.859712287474666770, 100.0000000000000000, -22.17872625191749236 ) ) ;
#5301=DIRECTION ( 'NONE',  ( 0.9197781680807419757, 0.000000000000000000, -0.3924386850477849520 ) ) ;
#5304=CARTESIAN_POINT ( 'NONE',  ( -22.25406130147340633, 100.0000000000000000, -9.998337329044998611 ) ) ;
#5305=EDGE_CURVE ( 'NONE', #5423, #3612, #2446, .T. ) ;
#5306=CARTESIAN_POINT ( 'NONE',  ( -16.01161620991261358, 100.0000000000000000, 17.10240122391520146 ) ) ;
#5308=CARTESIAN_POINT ( 'NONE',  ( 4.154273145530666511, 99.50000000000000000, -22.82723029927519676 ) ) ;
#5310=CARTESIAN_POINT ( 'NONE',  ( 3.058419780146050648, 100.0000000000000000, -23.12871267107006545 ) ) ;
#5312=( BOUNDED_CURVE ( )  B_SPLINE_CURVE ( 2, ( #282, #6710, #9906, #9126, #437, #2848, #2055, #5140, #8340 ),
 .UNSPECIFIED., .F., .T. ) 
 B_SPLINE_CURVE_WITH_KNOTS ( ( 3, 2, 2, 2, 3 ),
 ( 0.7500000000000000000, 0.7678571428571429047, 0.7857142857142856984, 0.8035714285714286031, 0.8214285714285713969 ),
 .UNSPECIFIED. ) 
 CURVE ( )  GEOMETRIC_REPRESENTATION_ITEM ( )  RATIONAL_B_SPLINE_CURVE ( ( 1.000000000000000000, 0.9238795325112867385, 1.000000000000000000, 0.9238795325112867385, 1.000000000000000000, 0.9238795325112867385, 1.000000000000000000, 0.9238795325112867385, 1.000000000000000000 ) ) 
 REPRESENTATION_ITEM ( '' )  );
#5313=B_SPLINE_CURVE_WITH_KNOTS ( 'NONE', 3,
 ( #9995, #10216, #2201, #6848, #5172, #9373, #8371, #1309, #2087, #8595, #4607, #2030, #9256, #5283, #8423 ),
 .UNSPECIFIED., .F., .F.,
 ( 4, 1, 1, 1, 1, 1, 1, 1, 1, 1, 1, 1, 4 ),
 ( 0.000000000000000000, 0.08635447908391848115, 0.1695936995346988552, 0.2509241109261274860, 0.3325843554298174576, 0.4138183564518133073, 0.4948404748415979881, 0.5772065644957810049, 0.6619893985813737336, 0.7474108716807353892, 0.8313115314839791825, 0.9147691218156368542, 1.000000000000000000 ),
 .UNSPECIFIED. ) ;
#5314=EDGE_CURVE ( 'NONE', #7448, #7769, #8988, .T. ) ;
#5316=CARTESIAN_POINT ( 'NONE',  ( 5.243816414761435674, 100.0000000000000000, -23.48558366465980995 ) ) ;
#5317=EDGE_CURVE ( 'NONE', #717, #4569, #4815, .T. ) ;
#5320=VERTEX_POINT ( 'NONE', #5206 ) ;
#5321=LINE ( 'NONE', #4424, #380 ) ;
#5325=CARTESIAN_POINT ( 'NONE',  ( 9.910564025336874749, 99.50000000000001421, 20.75459158945058036 ) ) ;
#5327=ADVANCED_FACE ( 'NONE', ( #8461 ), #509, .T. ) ;
#5332=ORIENTED_EDGE ( 'NONE', *, *, #9066, .T. ) ;
#5334=CARTESIAN_POINT ( 'NONE',  ( 19.39806930854668110, 2.849999998907525089, -19.39806930854668110 ) ) ;
#5338=SHAPE_DEFINITION_REPRESENTATION ( #2431, #4065 ) ;
#5339=CARTESIAN_POINT ( 'NONE',  ( -22.64023588676181475, 99.50000000000000000, -10.01165679465830927 ) ) ;
#5342=CARTESIAN_POINT ( 'NONE',  ( 19.39806930854668110, 5.149999998907524912, -19.39806930854668110 ) ) ;
#5343=CARTESIAN_POINT ( 'NONE',  ( -27.43301270000000258, 3.099999998907525089, -11.36312591709336317 ) ) ;
#5346=CARTESIAN_POINT ( 'NONE',  ( -16.24524625128438515, 100.0000000000000284, 16.53274063862002308 ) ) ;
#5348=LINE ( 'NONE', #3879, #9901 ) ;
#5349=CARTESIAN_POINT ( 'NONE',  ( 0.000000000000000000, 87.00000000000001421, 0.000000000000000000 ) ) ;
#5350=ORIENTED_EDGE ( 'NONE', *, *, #3721, .F. ) ;
#5352=CARTESIAN_POINT ( 'NONE',  ( -22.22752541189434794, 99.49999999999994316, -11.26717589342885084 ) ) ;
#5353=ORIENTED_EDGE ( 'NONE', *, *, #9785, .F. ) ;
#5354=ADVANCED_FACE ( 'NONE', ( #6942 ), #1455, .T. ) ;
#5355=DIRECTION ( 'NONE',  ( 0.000000000000000000, -0.000000000000000000, 1.000000000000000000 ) ) ;
#5356=CARTESIAN_POINT ( 'NONE',  ( -27.43301270000000258, 3.049999998907525267, -3.359575119402369376E-15 ) ) ;
#5360=CARTESIAN_POINT ( 'NONE',  ( -20.63200021313574695, 100.0000000000000000, -10.19493994959453431 ) ) ;
#5361=CARTESIAN_POINT ( 'NONE',  ( 8.901217755223779449, 100.0000000000000711, 19.92336871027421097 ) ) ;
#5362=ORIENTED_EDGE ( 'NONE', *, *, #4984, .F. ) ;
#5363=CARTESIAN_POINT ( 'NONE',  ( -16.57330815294036697, 99.50000000000001421, 15.84440382193293217 ) ) ;
#5364=CARTESIAN_POINT ( 'NONE',  ( 8.102924533678123709, 99.50000000000000000, 20.98904009517733726 ) ) ;
#5369=CARTESIAN_POINT ( 'NONE',  ( -20.97771390646102319, 99.50000000000002842, -10.03345247102482674 ) ) ;
#5372=LINE ( 'NONE', #1595, #9055 ) ;
#5373=ORIENTED_EDGE ( 'NONE', *, *, #4110, .T. ) ;
#5374=CARTESIAN_POINT ( 'NONE',  ( 1.653273178848927064E-15, 5.599999997815050534, -27.00000000000000355 ) ) ;
#5375=CARTESIAN_POINT ( 'NONE',  ( 4.570993444255353921, 99.49999999999998579, -21.37574484917381668 ) ) ;
#5376=CARTESIAN_POINT ( 'NONE',  ( -19.09188309203678813, 1.300000000000000266, 19.09188309203678457 ) ) ;
#5377=CARTESIAN_POINT ( 'NONE',  ( -16.07368679829020763, 100.0000000000000000, 17.11560437002838952 ) ) ;
#5382=EDGE_LOOP ( 'NONE', ( #7605, #588, #5942, #7823 ) ) ;
#5383=DIRECTION ( 'NONE',  ( -0.9572638942369904314, 0.000000000000000000, 0.2892158999609669712 ) ) ;
#5384=CARTESIAN_POINT ( 'NONE',  ( 8.465276868207817884, 100.0000000000000142, 19.66343818277063704 ) ) ;
#5385=B_SPLINE_CURVE_WITH_KNOTS ( 'NONE', 3,
 ( #5727, #6598, #9009, #1829, #9890, #1003, #9788, #2625, #1931, #7480, #8913, #320, #7335, #5024, #8221, #3459, #269, #1736, #4246 ),
 .UNSPECIFIED., .F., .F.,
 ( 4, 1, 1, 1, 1, 1, 1, 1, 1, 1, 1, 1, 1, 1, 1, 1, 4 ),
 ( 0.000000000000000000, 0.08029080299619884009, 0.1602734547033792534, 0.2412010114815648643, 0.3246404098231062685, 0.3670482715230247162, 0.4085690013065461645, 0.4496707568484641926, 0.4905395156191099670, 0.5313644394553277417, 0.5726744073239632415, 0.6138178896263115636, 0.6555018086025313773, 0.7394546411270094266, 0.8240219501092651555, 0.9101625766452680066, 1.000000000000000000 ),
 .UNSPECIFIED. ) ;
#5387=CARTESIAN_POINT ( 'NONE',  ( -16.56356094049941419, 99.49999999999997158, 15.77213757552179629 ) ) ;
#5388=EDGE_LOOP ( 'NONE', ( #2047, #7952, #5931, #3347 ) ) ;
#5389=CARTESIAN_POINT ( 'NONE',  ( -16.42071764973191250, 100.0000000000000142, 16.76105279315999042 ) ) ;
#5390=VECTOR ( 'NONE', #5036, 1000.000000000000114 ) ;
#5391=CARTESIAN_POINT ( 'NONE',  ( -27.43301270000000258, 1.549999998907525267, -3.359575119402369376E-15 ) ) ;
#5393=ORIENTED_EDGE ( 'NONE', *, *, #1977, .T. ) ;
#5394=EDGE_CURVE ( 'NONE', #872, #5320, #9314, .T. ) ;
#5397=DIRECTION ( 'NONE',  ( 0.000000000000000000, -0.000000000000000000, 1.000000000000000000 ) ) ;
#5399=CARTESIAN_POINT ( 'NONE',  ( -16.74216497804568604, 99.50000000000001421, 15.31795814478965312 ) ) ;
#5400=CARTESIAN_POINT ( 'NONE',  ( -11.36312591709337383, 0.8999999989075252449, 27.43301269999999548 ) ) ;
#5403=DIRECTION ( 'NONE',  ( -0.8616861851997287269, 0.000000000000000000, 0.5074415416931677969 ) ) ;
#5405=CARTESIAN_POINT ( 'NONE',  ( 2.837666006185522782, 99.50000000000000000, -22.03040394835428373 ) ) ;
#5406=CARTESIAN_POINT ( 'NONE',  ( 5.243816414761435674, 99.50000000000000000, -23.48558366465980995 ) ) ;
#5407=EDGE_LOOP ( 'NONE', ( #2301, #10277, #6617, #179 ) ) ;
#5409=CARTESIAN_POINT ( 'NONE',  ( 4.433602057339688152, 99.50000000000000000, -21.25644978738549540 ) ) ;
#5410=ORIENTED_EDGE ( 'NONE', *, *, #967, .T. ) ;
#5412=CARTESIAN_POINT ( 'NONE',  ( 27.43301270000000258, 1.099999998907525089, -11.36312591709336139 ) ) ;
#5417=DIRECTION ( 'NONE',  ( -0.000000000000000000, -1.000000000000000000, -0.000000000000000000 ) ) ;
#5418=CARTESIAN_POINT ( 'NONE',  ( 8.540544597724410991, 100.0000000000000284, 19.98924338346217766 ) ) ;
#5420=CARTESIAN_POINT ( 'NONE',  ( -16.45635306197508996, 99.50000000000000000, 15.51056558312563105 ) ) ;
#5421=CARTESIAN_POINT ( 'NONE',  ( 8.187169943530866689, 99.99999999999998579, 20.27434297626003712 ) ) ;
#5423=VERTEX_POINT ( 'NONE', #5264 ) ;
#5425=ORIENTED_EDGE ( 'NONE', *, *, #5787, .T. ) ;
#5426=B_SPLINE_CURVE_WITH_KNOTS ( 'NONE', 3,
 ( #2697, #8243, #2646, #5788, #5939, #8982, #5836, #4266, #5745, #339, #8195, #9132, #5147, #1175, #1071, #9914, #3377, #6524, #4949 ),
 .UNSPECIFIED., .F., .F.,
 ( 4, 1, 1, 1, 1, 1, 1, 1, 1, 1, 1, 1, 1, 1, 1, 1, 4 ),
 ( 0.000000000000000000, 0.06463354665699841406, 0.1274839167070160040, 0.1893660780973640267, 0.2502738481868047038, 0.3108090901939400408, 0.3728692346228669741, 0.4358265942208103261, 0.5002515515682643965, 0.5647461136436963125, 0.6273730017603231790, 0.6892793264321037672, 0.7497280364991398827, 0.8111249352628771003, 0.8723480300361200479, 0.9354359082354426480, 1.000000000000000000 ),
 .UNSPECIFIED. ) ;
#5427=CARTESIAN_POINT ( 'NONE',  ( -15.34367147589386349, 100.0000000000000426, 16.87599331055909602 ) ) ;
#5428=CARTESIAN_POINT ( 'NONE',  ( -21.24882413972086681, 99.50000000000002842, -9.742484589929601313 ) ) ;
#5430=CARTESIAN_POINT ( 'NONE',  ( 5.142436925601051811, 99.49999999999995737, -24.04117066426968563 ) ) ;
#5434=ORIENTED_EDGE ( 'NONE', *, *, #8411, .F. ) ;
#5435=CARTESIAN_POINT ( 'NONE',  ( 3.124251205490514494, 99.50000000000000000, -23.02140944421609703 ) ) ;
#5437=ORIENTED_EDGE ( 'NONE', *, *, #9704, .T. ) ;
#5440=CARTESIAN_POINT ( 'NONE',  ( -21.79396932678589849, 100.0000000000000000, -9.306975108219608828 ) ) ;
#5441=CARTESIAN_POINT ( 'NONE',  ( 4.331079892889020400, 99.50000000000000000, -24.67336562508343079 ) ) ;
#5442=EDGE_CURVE ( 'NONE', #6092, #498, #3702, .T. ) ;
#5443=CARTESIAN_POINT ( 'NONE',  ( -22.28244091826395135, 100.0000000000000000, -10.68852969318427881 ) ) ;
#5445=CARTESIAN_POINT ( 'NONE',  ( -15.49723655759404295, 99.49999999999997158, 15.26389171799780264 ) ) ;
#5446=CARTESIAN_POINT ( 'NONE',  ( 1.679787559701184688E-15, 1.349999998907525312, -27.43301270000000258 ) ) ;
#5454=CARTESIAN_POINT ( 'NONE',  ( 4.739008722453744049, 99.50000000000001421, -24.06821587619827696 ) ) ;
#5455=CARTESIAN_POINT ( 'NONE',  ( -27.43301270000000969, 3.199999998907525178, 11.36312591709335429 ) ) ;
#5456=EDGE_LOOP ( 'NONE', ( #9337, #4253, #7844, #922 ) ) ;
#5458=CARTESIAN_POINT ( 'NONE',  ( -15.22739782325755442, 99.49999999999998579, 15.50750051783781025 ) ) ;
#5461=LINE ( 'NONE', #8650, #4931 ) ;
#5463=CARTESIAN_POINT ( 'NONE',  ( 4.691018317478480526, 99.99999999999995737, -21.52316599815148024 ) ) ;
#5466=CARTESIAN_POINT ( 'NONE',  ( -19.39806930854667755, 2.149999998907525356, -19.39806930854668110 ) ) ;
#5469=CARTESIAN_POINT ( 'NONE',  ( 19.09188309203678102, 1.500000000000000000, 19.09188309203678813 ) ) ;
#5470=CARTESIAN_POINT ( 'NONE',  ( 9.044794778432494908, 100.0000000000000426, 19.94873160813952140 ) ) ;
#5472=CARTESIAN_POINT ( 'NONE',  ( -16.45391695211397831, 99.50000000000004263, 16.32580124622701589 ) ) ;
#5476=ORIENTED_EDGE ( 'NONE', *, *, #9469, .T. ) ;
#5477=CARTESIAN_POINT ( 'NONE',  ( -11.36312591709335962, 3.699999998907525622, -27.43301270000000258 ) ) ;
#5479=VECTOR ( 'NONE', #5148, 1000.000000000000000 ) ;
#5482=CARTESIAN_POINT ( 'NONE',  ( 4.850954546176396320, 100.0000000000000142, -24.43907202982397209 ) ) ;
#5483=ORIENTED_EDGE ( 'NONE', *, *, #4438, .T. ) ;
#5486=CARTESIAN_POINT ( 'NONE',  ( 4.232798786556307036, 99.50000000000000000, -24.34936571594186105 ) ) ;
#5488=ORIENTED_EDGE ( 'NONE', *, *, #5630, .T. ) ;
#5489=CARTESIAN_POINT ( 'NONE',  ( -16.33590634957226229, 99.50000000000000000, 16.80570853669505382 ) ) ;
#5492=ORIENTED_EDGE ( 'NONE', *, *, #4682, .F. ) ;
#5493=CARTESIAN_POINT ( 'NONE',  ( 4.295198626299898237, 99.50000000000001421, -24.68029520312135361 ) ) ;
#5494=CARTESIAN_POINT ( 'NONE',  ( 9.725694684612619767, 100.0000000000000000, 20.03234812723199454 ) ) ;
#5495=CARTESIAN_POINT ( 'NONE',  ( -16.37547766376588854, 99.50000000000000000, 16.41943072543956816 ) ) ;
#5496=ORIENTED_EDGE ( 'NONE', *, *, #4254, .F. ) ;
#5497=CARTESIAN_POINT ( 'NONE',  ( -15.03933290382598820, 99.50000000000000000, 15.19633946010233849 ) ) ;
#5498=CARTESIAN_POINT ( 'NONE',  ( 27.43301270000000258, 5.199999998907525622, -11.36312591709336139 ) ) ;
#5500=CIRCLE ( 'NONE', #8674, 7.500000000000000000 ) ;
#5502=ADVANCED_FACE ( 'NONE', ( #777, #6272 ), #7946, .T. ) ;
#5505=CARTESIAN_POINT ( 'NONE',  ( 3.269123371500344710, 99.50000000000001421, -23.64665713169964434 ) ) ;
#5507=CARTESIAN_POINT ( 'NONE',  ( -16.85368146453285831, 99.49999999999998579, 16.27421966797335529 ) ) ;
#5508=CARTESIAN_POINT ( 'NONE',  ( -27.43301270000000258, 3.949999998907525178, -3.359575119402369376E-15 ) ) ;
#5509=CARTESIAN_POINT ( 'NONE',  ( -15.30604604128650692, 99.50000000000000000, 15.41317891555018349 ) ) ;
#5510=CARTESIAN_POINT ( 'NONE',  ( 3.735769352376668184, 99.99999999999998579, -24.30643046864489420 ) ) ;
#5511=CARTESIAN_POINT ( 'NONE',  ( 2.852289972453743161, 99.50000000000000000, -22.14293542748032451 ) ) ;
#5512=CARTESIAN_POINT ( 'NONE',  ( -22.64023588676181475, 100.0000000000000000, -10.01165679465830927 ) ) ;
#5514=CARTESIAN_POINT ( 'NONE',  ( 4.633286773149219329, 99.50000000000002842, -21.44575434969419447 ) ) ;
#5515=VERTEX_POINT ( 'NONE', #5493 ) ;
#5517=CARTESIAN_POINT ( 'NONE',  ( -11.36312591709337383, 3.999999998907525889, 27.43301269999999548 ) ) ;
#5518=B_SPLINE_CURVE_WITH_KNOTS ( 'NONE', 3,
 ( #8394, #334, #235, #1996, #8237, #5833, #9079, #5195, #6711, #8190, #5141, #2641, #8341, #9025, #5880, #2797, #5783, #2742, #6765 ),
 .UNSPECIFIED., .F., .F.,
 ( 4, 1, 1, 1, 1, 1, 1, 1, 1, 1, 1, 1, 1, 1, 1, 1, 4 ),
 ( 0.000000000000000000, 0.06473908249738200005, 0.1274869542813800993, 0.1888754624962200035, 0.2498352098569301405, 0.3101749858420705941, 0.3718734486855839183, 0.4342313324889700565, 0.4990836447755341299, 0.5639614065304963120, 0.6264045329497629488, 0.6882484937299673255, 0.7493615009078817835, 0.8100377551054726011, 0.8717391907241844873, 0.9348513958286107650, 1.000000000000000000 ),
 .UNSPECIFIED. ) ;
#5520=CARTESIAN_POINT ( 'NONE',  ( 26.99999999999999645, 0.7500000000000001110, 11.18376618407358691 ) ) ;
#5521=CARTESIAN_POINT ( 'NONE',  ( 9.304660012616079001, 99.50000000000000000, 20.07619068507570859 ) ) ;
#5522=PLANE ( 'NONE',  #464 ) ;
#5523=CARTESIAN_POINT ( 'NONE',  ( -15.31787750341841559, 100.0000000000000000, 16.43551622900274722 ) ) ;
#5526=EDGE_LOOP ( 'NONE', ( #6245, #490 ) ) ;
#5527=CARTESIAN_POINT ( 'NONE',  ( 27.43301270000000258, 3.499999998907525445, -11.36312591709336139 ) ) ;
#5528=CARTESIAN_POINT ( 'NONE',  ( 3.824506687597884369, 99.50000000000002842, -24.68145443631992109 ) ) ;
#5529=B_SPLINE_SURFACE_WITH_KNOTS ( 'NONE', 3, 1, ( 
 ( #3040, #461 ),
 ( #9242, #2984 ),
 ( #1406, #5389 ),
 ( #4597, #4434 ),
 ( #2869, #5270 ),
 ( #7001, #6838 ),
 ( #2247, #1295 ) ),
 .UNSPECIFIED., .F., .F., .F.,
 ( 4, 1, 1, 1, 4 ),
 ( 2, 2 ),
 ( 0.000000000000000000, 0.2687002788711734813, 0.5225003893189538173, 0.7676814173175746658, 1.000000000000000000 ),
 ( 0.000000000000000000, 1.000000000000000000 ),
 .UNSPECIFIED. ) ;
#5532=CARTESIAN_POINT ( 'NONE',  ( -16.56313167360273297, 100.0000000000000284, 16.06491815633068398 ) ) ;
#5533=DIRECTION ( 'NONE',  ( -0.9985534407235125975, 0.000000000000000000, 0.05376826219280737146 ) ) ;
#5535=ORIENTED_EDGE ( 'NONE', *, *, #9672, .F. ) ;
#5538=CARTESIAN_POINT ( 'NONE',  ( 4.820889542125314620, 99.99999999999998579, -21.76289454767624676 ) ) ;
#5539=CARTESIAN_POINT ( 'NONE',  ( -15.15193744131588183, 100.0000000000000142, 16.74589488344418697 ) ) ;
#5540=CARTESIAN_POINT ( 'NONE',  ( 8.644881627383616873, 99.49999999999995737, 19.60534525227960145 ) ) ;
#5543=CARTESIAN_POINT ( 'NONE',  ( -22.12191435419165941, 100.0000000000000142, -9.834338183724410598 ) ) ;
#5546=CARTESIAN_POINT ( 'NONE',  ( -16.36254897777739004, 99.50000000000001421, 15.39785597259249350 ) ) ;
#5547=CARTESIAN_POINT ( 'NONE',  ( -19.39806930854667755, 3.849999998907525089, -19.39806930854668110 ) ) ;
#5548=ORIENTED_EDGE ( 'NONE', *, *, #2500, .F. ) ;
#5550=CARTESIAN_POINT ( 'NONE',  ( -21.07742585509981126, 99.99999999999998579, -10.85999754779651383 ) ) ;
#5552=CARTESIAN_POINT ( 'NONE',  ( -20.52076770522338833, 99.50000000000000000, -10.69798695537560462 ) ) ;
#5553=CARTESIAN_POINT ( 'NONE',  ( 19.39806930854668110, 5.249999998907525445, -19.39806930854668110 ) ) ;
#5554=CARTESIAN_POINT ( 'NONE',  ( -15.15623813234777018, 99.99999999999997158, 16.19783826294960249 ) ) ;
#5555=CARTESIAN_POINT ( 'NONE',  ( 19.09188309203678102, 3.699999997815051067, 19.09188309203678813 ) ) ;
#5556=CARTESIAN_POINT ( 'NONE',  ( 2.955068081869620666, 99.49999999999998579, -21.57801138750623338 ) ) ;
#5557=EDGE_CURVE ( 'NONE', #4730, #7160, #8832, .T. ) ;
#5558=CARTESIAN_POINT ( 'NONE',  ( 19.09188309203678813, 4.100000000000000533, -19.09188309203678813 ) ) ;
#5560=CARTESIAN_POINT ( 'NONE',  ( 3.681717055787076642, 99.50000000000000000, -21.09125273517263111 ) ) ;
#5561=ORIENTED_EDGE ( 'NONE', *, *, #699, .T. ) ;
#5563=CARTESIAN_POINT ( 'NONE',  ( -19.39806930854668465, 0.8499999989075252005, 19.39806930854667755 ) ) ;
#5567=CARTESIAN_POINT ( 'NONE',  ( -27.00000000000000355, 3.600000000000000533, -3.306546357697854128E-15 ) ) ;
#5568=CARTESIAN_POINT ( 'NONE',  ( 3.373335371007685435, 100.0000000000000000, -22.75111425220066863 ) ) ;
#5569=EDGE_LOOP ( 'NONE', ( #8389, #4629, #6457, #6430 ) ) ;
#5570=EDGE_LOOP ( 'NONE', ( #3719, #4114, #5496, #1432 ) ) ;
#5572=CARTESIAN_POINT ( 'NONE',  ( -15.49014769301379069, 99.49999999999997158, 16.56834637662448273 ) ) ;
#5573=ORIENTED_EDGE ( 'NONE', *, *, #6738, .F. ) ;
#5575=ORIENTED_EDGE ( 'NONE', *, *, #8116, .T. ) ;
#5577=CARTESIAN_POINT ( 'NONE',  ( -27.43301270000000969, 1.499999998907525445, 11.36312591709335784 ) ) ;
#5578=CARTESIAN_POINT ( 'NONE',  ( 1.653273178848927064E-15, 1.800000000000000266, -27.00000000000000355 ) ) ;
#5579=CARTESIAN_POINT ( 'NONE',  ( -21.84904385032055174, 99.49999999999998579, -11.42736543092427404 ) ) ;
#5581=FACE_OUTER_BOUND ( 'NONE', #5388, .T. ) ;
#5582=CARTESIAN_POINT ( 'NONE',  ( -16.85368146453285831, 99.49999999999998579, 16.27421966797335529 ) ) ;
#5583=CARTESIAN_POINT ( 'NONE',  ( 8.117007248954752896, 100.0000000000000142, 20.40979824468519155 ) ) ;
#5584=EDGE_CURVE ( 'NONE', #6241, #3123, #6184, .T. ) ;
#5586=EDGE_CURVE ( 'NONE', #6302, #533, #3213, .T. ) ;
#5589=CARTESIAN_POINT ( 'NONE',  ( 4.311343222282856047, 100.0000000000000142, -24.33387958695581688 ) ) ;
#5590=DIRECTION ( 'NONE',  ( 0.000000000000000000, 1.000000000000000000, 0.000000000000000000 ) ) ;
#5591=CARTESIAN_POINT ( 'NONE',  ( -14.78677372028383097, 99.99999999999998579, 15.63810349997947569 ) ) ;
#5593=CARTESIAN_POINT ( 'NONE',  ( 2.936358689207804851, 99.50000000000000000, -23.74786164940363875 ) ) ;
#5595=CARTESIAN_POINT ( 'NONE',  ( -22.17094027205346052, 99.50000000000001421, -9.884352203306939089 ) ) ;
#5596=DIRECTION ( 'NONE',  ( -0.2149789550291109352, 0.000000000000000000, -0.9766186814179788067 ) ) ;
#5597=CARTESIAN_POINT ( 'NONE',  ( 11.36312591709336850, 4.199999998907525622, 27.43301269999999903 ) ) ;
#5601=CARTESIAN_POINT ( 'NONE',  ( 3.328702480760086235, 99.49999999999997158, -23.35145716610488975 ) ) ;
#5603=CARTESIAN_POINT ( 'NONE',  ( -20.96129225301843135, 99.50000000000001421, -10.68089388303413934 ) ) ;
#5604=CARTESIAN_POINT ( 'NONE',  ( -11.36312591709335962, 4.599999998907525978, -27.43301270000000258 ) ) ;
#5605=CARTESIAN_POINT ( 'NONE',  ( -15.30066472929571653, 99.49999999999998579, 16.41738810589640707 ) ) ;
#5606=PLANE ( 'NONE',  #9815 ) ;
#5607=CARTESIAN_POINT ( 'NONE',  ( -15.42956291708403782, 99.49999999999998579, 16.53061251458192515 ) ) ;
#5608=B_SPLINE_SURFACE_WITH_KNOTS ( 'NONE', 3, 1, ( 
 ( #1146, #3447 ),
 ( #4337, #6636 ),
 ( #9832, #6588 ),
 ( #3499, #2570 ),
 ( #5810, #2615 ),
 ( #2772, #5169 ),
 ( #5064, #6685 ),
 ( #9779, #7521 ),
 ( #9938, #2664 ),
 ( #8953, #5856 ),
 ( #9001, #362 ) ),
 .UNSPECIFIED., .F., .F., .F.,
 ( 4, 1, 1, 1, 1, 1, 1, 1, 4 ),
 ( 2, 2 ),
 ( 0.000000000000000000, 0.1307887167449866828, 0.2576322083635017579, 0.3824781763252146916, 0.5056045358258490774, 0.6278910088851102911, 0.7502354365656509483, 0.8735741898580190457, 1.000000000000000000 ),
 ( 0.000000000000000000, 1.000000000000000000 ),
 .UNSPECIFIED. ) ;
#5609=CARTESIAN_POINT ( 'NONE',  ( -22.43208371148383762, 100.0000000000000000, -9.654966607469265938 ) ) ;
#5611=CARTESIAN_POINT ( 'NONE',  ( 4.358720771404392735, 100.0000000000000000, -21.20742720589606378 ) ) ;
#5615=CARTESIAN_POINT ( 'NONE',  ( 11.36312591709336850, 0.9999999989075254447, 27.43301269999999903 ) ) ;
#5616=CARTESIAN_POINT ( 'NONE',  ( -16.49882833452567965, 99.50000000000000000, 15.05677840364783115 ) ) ;
#5618=CARTESIAN_POINT ( 'NONE',  ( 19.39806930854668110, 0.3499999989075252560, -19.39806930854668110 ) ) ;
#5620=AXIS2_PLACEMENT_3D ( 'NONE', #2998, #5403, #528 ) ;
#5622=CARTESIAN_POINT ( 'NONE',  ( 19.09188309203678102, 2.099999997815050090, 19.09188309203678813 ) ) ;
#5623=AXIS2_PLACEMENT_3D ( 'NONE', #6202, #1496, #7934 ) ;
#5625=CARTESIAN_POINT ( 'NONE',  ( 27.43301269999999548, 2.599999998907525089, 11.36312591709337916 ) ) ;
#5626=CARTESIAN_POINT ( 'NONE',  ( 4.295198626299898237, 100.0000000000000142, -24.68029520312135361 ) ) ;
#5627=DIRECTION ( 'NONE',  ( 0.9197781680807419757, 0.000000000000000000, -0.3924386850477849520 ) ) ;
#5629=DIRECTION ( 'NONE',  ( -0.000000000000000000, -1.000000000000000000, -0.000000000000000000 ) ) ;
#5630=EDGE_CURVE ( 'NONE', #834, #1366, #7374, .T. ) ;
#5631=CARTESIAN_POINT ( 'NONE',  ( -16.90689012439429462, 99.99999999999998579, 16.08742389234230785 ) ) ;
#5632=CARTESIAN_POINT ( 'NONE',  ( 5.243816414761435674, 100.0000000000000000, -23.48558366465980995 ) ) ;
#5633=EDGE_CURVE ( 'NONE', #4987, #717, #6450, .T. ) ;
#5636=CARTESIAN_POINT ( 'NONE',  ( 4.232798786556307036, 100.0000000000000142, -24.34936571594186105 ) ) ;
#5638=EDGE_CURVE ( 'NONE', #2588, #9675, #9735, .T. ) ;
#5639=CARTESIAN_POINT ( 'NONE',  ( -15.03933290382598820, 100.0000000000000000, 15.19633946010233849 ) ) ;
#5641=EDGE_CURVE ( 'NONE', #647, #7160, #5859, .T. ) ;
#5645=VECTOR ( 'NONE', #4307, 1000.000000000000000 ) ;
#5646=EDGE_CURVE ( 'NONE', #1777, #7350, #7331, .T. ) ;
#5647=CARTESIAN_POINT ( 'NONE',  ( -22.06741020400400188, 99.50000000000004263, -9.788922322134999021 ) ) ;
#5649=CARTESIAN_POINT ( 'NONE',  ( 9.114876806416853938, 99.99999999999998579, 19.97295714941878231 ) ) ;
#5650=VERTEX_POINT ( 'NONE', #6745 ) ;
#5651=CARTESIAN_POINT ( 'NONE',  ( 4.405197143102897783, 99.49999999999995737, -21.72932741277565682 ) ) ;
#5653=CARTESIAN_POINT ( 'NONE',  ( 3.659868213429061878, 100.0000000000000000, -22.50687739797974274 ) ) ;
#5655=CARTESIAN_POINT ( 'NONE',  ( 27.00000000000000355, 2.249999997815050445, -11.18376618407356737 ) ) ;
#5657=CARTESIAN_POINT ( 'NONE',  ( 5.725936192474917696, 99.50000000000000000, 21.08018326417248645 ) ) ;
#5658=B_SPLINE_CURVE_WITH_KNOTS ( 'NONE', 3,
 ( #6391, #2415, #8800, #4268, #111, #392, #3303, #288, #1899, #9082, #2000, #9970, #6443, #9180, #6718, #6492, #1072, #7222, #9915 ),
 .UNSPECIFIED., .F., .F.,
 ( 4, 1, 1, 1, 1, 1, 1, 1, 1, 1, 1, 1, 1, 1, 1, 1, 4 ),
 ( 0.000000000000000000, 0.07313710028058939550, 0.1429478298248799129, 0.2105045057187734658, 0.2751999312753631854, 0.3390602298032547868, 0.4018764873508149926, 0.4650016082884899093, 0.5281538368899733049, 0.5906348070863262079, 0.6510495490485337378, 0.7103018853965116230, 0.7674338915725752441, 0.8249350906448947862, 0.8823686014076175255, 0.9405824579944982444, 1.000000000000000000 ),
 .UNSPECIFIED. ) ;
#5659=CARTESIAN_POINT ( 'NONE',  ( 1.653273178848927064E-15, 3.999999997815050889, -27.00000000000000355 ) ) ;
#5660=CARTESIAN_POINT ( 'NONE',  ( -16.30427144417478402, 99.49999999999998579, 16.48895498912494517 ) ) ;
#5662=AXIS2_PLACEMENT_3D ( 'NONE', #999, #9160, #5020 ) ;
#5664=FACE_OUTER_BOUND ( 'NONE', #9163, .T. ) ;
#5667=CARTESIAN_POINT ( 'NONE',  ( -5.039362679103552881E-15, 1.749999998907525223, 27.43301270000000258 ) ) ;
#5670=CARTESIAN_POINT ( 'NONE',  ( 1.653273178848927064E-15, 4.200000000000000178, -27.00000000000000355 ) ) ;
#5672=CARTESIAN_POINT ( 'NONE',  ( -20.97746206809550884, 100.0000000000000000, -11.22189255051946688 ) ) ;
#5674=CARTESIAN_POINT ( 'NONE',  ( -16.40919047799676989, 99.99999999999995737, 16.38364531277195013 ) ) ;
#5675=CARTESIAN_POINT ( 'NONE',  ( 11.18376618407357093, 2.349999997815050090, -27.00000000000000355 ) ) ;
#5677=CARTESIAN_POINT ( 'NONE',  ( 27.43301269999999548, 1.799999998907525045, 11.36312591709337916 ) ) ;
#5678=CARTESIAN_POINT ( 'NONE',  ( 3.238942592553923472, 99.50000000000001421, -24.36085717291697250 ) ) ;
#5680=CARTESIAN_POINT ( 'NONE',  ( -11.18376618407358336, 1.149999997815050357, 26.99999999999999645 ) ) ;
#5682=CARTESIAN_POINT ( 'NONE',  ( 8.132491713109025966, 100.0000000000000000, 21.08089001807756091 ) ) ;
#5683=CARTESIAN_POINT ( 'NONE',  ( -16.74216497804568604, 100.0000000000000142, 15.31795814478965312 ) ) ;
#5685=VERTEX_POINT ( 'NONE', #315 ) ;
#5687=ORIENTED_EDGE ( 'NONE', *, *, #2754, .T. ) ;
#5689=CARTESIAN_POINT ( 'NONE',  ( 4.259295290443009918, 100.0000000000000426, -24.34414156132068996 ) ) ;
#5691=LINE ( 'NONE', #925, #10238 ) ;
#5696=CARTESIAN_POINT ( 'NONE',  ( -15.18657300206754179, 99.50000000000000000, 16.26161032743331347 ) ) ;
#5699=CARTESIAN_POINT ( 'NONE',  ( 11.36312591709336139, 5.299999998907526155, -27.43301270000000258 ) ) ;
#5700=ORIENTED_EDGE ( 'NONE', *, *, #7539, .T. ) ;
#5701=FACE_OUTER_BOUND ( 'NONE', #1638, .T. ) ;
#5702=CARTESIAN_POINT ( 'NONE',  ( -21.12798922145720582, 100.0000000000000142, -10.90888695829967325 ) ) ;
#5704=ORIENTED_EDGE ( 'NONE', *, *, #4973, .T. ) ;
#5705=CARTESIAN_POINT ( 'NONE',  ( 4.061806280070601183, 100.0000000000000426, -22.51960061163626392 ) ) ;
#5706=CARTESIAN_POINT ( 'NONE',  ( -4.959819536546781389E-15, 1.199999997815050401, 27.00000000000000355 ) ) ;
#5709=CARTESIAN_POINT ( 'NONE',  ( 3.428794695218988053, 99.50000000000001421, -24.07607503615978572 ) ) ;
#5710=CARTESIAN_POINT ( 'NONE',  ( 3.254133136943549776, 100.0000000000000000, -21.76036676155726823 ) ) ;
#5712=DIRECTION ( 'NONE',  ( -0.000000000000000000, 1.000000000000000000, -0.000000000000000000 ) ) ;
#5714=CARTESIAN_POINT ( 'NONE',  ( 9.358681735871565266, 99.99999999999998579, 21.55373624431538815 ) ) ;
#5718=CARTESIAN_POINT ( 'NONE',  ( -15.84712739808237103, 99.49999999999997158, 14.83079670662049310 ) ) ;
#5719=( BOUNDED_SURFACE ( )  B_SPLINE_SURFACE ( 1, 2, ( 
 ( #321, #8176, #4197, #373, #3509, #6751, #9950, #8380, #1209, #4403, #9743, #5233, #1265, #9209, #2210, #4508, #3624, #5412, #7701, #10171, #3731, #481, #2039, #3057, #6804, #6857, #10053, #2890, #3008, #7021, #6238, #6075, #6129, #7759, #8433, #642, #9265, #9440, #5466, #4674, #4562, #2267, #7642, #10003, #4454, #6970, #3676, #2099, #1428, #6183, #5292, #9382, #8605, #9324, #4618, #8489, #5356, #1318, #6021, #7811, #7864, #1479, #3784, #8656, #538, #2838, #3837, #2948, #6913, #10112, #2155, #8545, #1369, #590, #10225, #5517, #7277, #3941, #3259, #7914, #6448, #748, #3994, #900, #3886, #853, #4722, #10330, #3306, #1684, #6347, #3163, #2649, #7179, #4042, #4825, #6496, #6295, #9033, #1633, #9813 ),
 ( #7126, #9542, #2366, #9637, #8709, #9493, #5839, #9586, #1850, #2418, #5563, #4091, #7073, #5615, #8754, #7226, #115, #6396, #2317, #5046, #1528, #2473, #1578, #8021, #10281, #4772, #7968, #802, #5667, #8, #694, #8856, #3211, #61, #8803, #4877, #8069, #3114, #8248, #1127, #4319, #7504, #4425, #1286, #505, #343, #396, #2003, #3484, #5258, #3533, #3699, #10078, #9290, #9184, #7668, #1903, #1075, #2701, #1232, #6668, #9864, #6042, #448, #5890, #3646, #10022, #3590, #6825, #5097, #9973, #2752, #292, #7611, #2123, #6097, #8402, #6881, #9085, #7451, #2857, #7557, #2914, #6722, #8348, #6775, #2807, #4271, #8457, #8297, #4476, #9919, #9232, #5945, #2064, #9136, #1180, #1956, #5151, #4370, #5992 ) ),
 .UNSPECIFIED., .F., .F., .T. ) 
 B_SPLINE_SURFACE_WITH_KNOTS ( ( 2, 2 ),
 ( 3, 2, 2, 2, 2, 2, 2, 2, 2, 2, 2, 2, 2, 2, 2, 2, 2, 2, 2, 2, 2, 2, 2, 2, 2, 2, 2, 2, 2, 2, 2, 2, 2, 2, 2, 2, 2, 2, 2, 2, 2, 2, 2, 2, 2, 2, 2, 2, 2, 2, 3 ),
 ( 0.000000000000000000, 1.000000000000000000 ),
 ( 0.000000000000000000, 0.01785714285714285615, 0.03571428571428571230, 0.05357142857142856845, 0.07142857142857142461, 0.08928571428571428770, 0.1071428571428571369, 0.1250000000000000000, 0.1428571428571428492, 0.1607142857142857262, 0.1785714285714285754, 0.1964285714285714246, 0.2142857142857142738, 0.2321428571428571508, 0.2500000000000000000, 0.2678571428571428492, 0.2857142857142856984, 0.3035714285714285476, 0.3214285714285714524, 0.3392857142857143016, 0.3571428571428571508, 0.3750000000000000000, 0.3928571428571428492, 0.4107142857142856984, 0.4285714285714285476, 0.4464285714285714524, 0.4642857142857143016, 0.4821428571428571508, 0.5000000000000000000, 0.5178571428571429047, 0.5357142857142856984, 0.5535714285714286031, 0.5714285714285713969, 0.5892857142857143016, 0.6071428571428570953, 0.6250000000000000000, 0.6428571428571429047, 0.6607142857142856984, 0.6785714285714286031, 0.6964285714285713969, 0.7142857142857143016, 0.7321428571428570953, 0.7500000000000000000, 0.7678571428571429047, 0.7857142857142856984, 0.8035714285714286031, 0.8214285714285713969, 0.8392857142857143016, 0.8571428571428570953, 0.8750000000000000000, 0.8928571428571429047 ),
 .UNSPECIFIED. ) 
 GEOMETRIC_REPRESENTATION_ITEM ( )  RATIONAL_B_SPLINE_SURFACE ( (
 ( 1.000000000000000000, 0.9238795325112867385, 1.000000000000000000, 0.9238795325112867385, 1.000000000000000000, 0.9238795325112867385, 1.000000000000000000, 0.9238795325112867385, 1.000000000000000000, 0.9238795325112867385, 1.000000000000000000, 0.9238795325112867385, 1.000000000000000000, 0.9238795325112867385, 1.000000000000000000, 0.9238795325112867385, 1.000000000000000000, 0.9238795325112867385, 1.000000000000000000, 0.9238795325112867385, 1.000000000000000000, 0.9238795325112867385, 1.000000000000000000, 0.9238795325112867385, 1.000000000000000000, 0.9238795325112867385, 1.000000000000000000, 0.9238795325112867385, 1.000000000000000000, 0.9238795325112867385, 1.000000000000000000, 0.9238795325112867385, 1.000000000000000000, 0.9238795325112867385, 1.000000000000000000, 0.9238795325112867385, 1.000000000000000000, 0.9238795325112867385, 1.000000000000000000, 0.9238795325112867385, 1.000000000000000000, 0.9238795325112867385, 1.000000000000000000, 0.9238795325112867385, 1.000000000000000000, 0.9238795325112867385, 1.000000000000000000, 0.9238795325112867385, 1.000000000000000000, 0.9238795325112867385, 1.000000000000000000, 0.9238795325112867385, 1.000000000000000000, 0.9238795325112867385, 1.000000000000000000, 0.9238795325112867385, 1.000000000000000000, 0.9238795325112867385, 1.000000000000000000, 0.9238795325112867385, 1.000000000000000000, 0.9238795325112867385, 1.000000000000000000, 0.9238795325112867385, 1.000000000000000000, 0.9238795325112867385, 1.000000000000000000, 0.9238795325112867385, 1.000000000000000000, 0.9238795325112867385, 1.000000000000000000, 0.9238795325112867385, 1.000000000000000000, 0.9238795325112867385, 1.000000000000000000, 0.9238795325112867385, 1.000000000000000000, 0.9238795325112867385, 1.000000000000000000, 0.9238795325112867385, 1.000000000000000000, 0.9238795325112867385, 1.000000000000000000, 0.9238795325112867385, 1.000000000000000000, 0.9238795325112867385, 1.000000000000000000, 0.9238795325112867385, 1.000000000000000000, 0.9238795325112867385, 1.000000000000000000, 0.9238795325112867385, 1.000000000000000000, 0.9238795325112867385, 1.000000000000000000, 0.9238795325112867385, 1.000000000000000000, 0.9238795325112867385, 1.000000000000000000, 0.9238795325112867385, 1.000000000000000000),
 ( 1.000000000000000000, 0.9238795325112867385, 1.000000000000000000, 0.9238795325112867385, 1.000000000000000000, 0.9238795325112867385, 1.000000000000000000, 0.9238795325112867385, 1.000000000000000000, 0.9238795325112867385, 1.000000000000000000, 0.9238795325112867385, 1.000000000000000000, 0.9238795325112867385, 1.000000000000000000, 0.9238795325112867385, 1.000000000000000000, 0.9238795325112867385, 1.000000000000000000, 0.9238795325112867385, 1.000000000000000000, 0.9238795325112867385, 1.000000000000000000, 0.9238795325112867385, 1.000000000000000000, 0.9238795325112867385, 1.000000000000000000, 0.9238795325112867385, 1.000000000000000000, 0.9238795325112867385, 1.000000000000000000, 0.9238795325112867385, 1.000000000000000000, 0.9238795325112867385, 1.000000000000000000, 0.9238795325112867385, 1.000000000000000000, 0.9238795325112867385, 1.000000000000000000, 0.9238795325112867385, 1.000000000000000000, 0.9238795325112867385, 1.000000000000000000, 0.9238795325112867385, 1.000000000000000000, 0.9238795325112867385, 1.000000000000000000, 0.9238795325112867385, 1.000000000000000000, 0.9238795325112867385, 1.000000000000000000, 0.9238795325112867385, 1.000000000000000000, 0.9238795325112867385, 1.000000000000000000, 0.9238795325112867385, 1.000000000000000000, 0.9238795325112867385, 1.000000000000000000, 0.9238795325112867385, 1.000000000000000000, 0.9238795325112867385, 1.000000000000000000, 0.9238795325112867385, 1.000000000000000000, 0.9238795325112867385, 1.000000000000000000, 0.9238795325112867385, 1.000000000000000000, 0.9238795325112867385, 1.000000000000000000, 0.9238795325112867385, 1.000000000000000000, 0.9238795325112867385, 1.000000000000000000, 0.9238795325112867385, 1.000000000000000000, 0.9238795325112867385, 1.000000000000000000, 0.9238795325112867385, 1.000000000000000000, 0.9238795325112867385, 1.000000000000000000, 0.9238795325112867385, 1.000000000000000000, 0.9238795325112867385, 1.000000000000000000, 0.9238795325112867385, 1.000000000000000000, 0.9238795325112867385, 1.000000000000000000, 0.9238795325112867385, 1.000000000000000000, 0.9238795325112867385, 1.000000000000000000, 0.9238795325112867385, 1.000000000000000000, 0.9238795325112867385, 1.000000000000000000, 0.9238795325112867385, 1.000000000000000000) ) ) 
 REPRESENTATION_ITEM ( '' )  SURFACE ( )  );
#5720=CARTESIAN_POINT ( 'NONE',  ( -4.959819536546781389E-15, 3.000000000000000000, 27.00000000000000355 ) ) ;
#5721=CARTESIAN_POINT ( 'NONE',  ( 2.964854786877021642, 99.50000000000000000, -22.43901021186594846 ) ) ;
#5724=CARTESIAN_POINT ( 'NONE',  ( -20.93486371557392545, 99.99999999999995737, -10.61231311368802466 ) ) ;
#5727=CARTESIAN_POINT ( 'NONE',  ( 2.940631318607589417, 100.0000000000000000, -23.77584808773673331 ) ) ;
#5729=VECTOR ( 'NONE', #8266, 1000.000000000000000 ) ;
#5732=CARTESIAN_POINT ( 'NONE',  ( 11.18376618407357093, 1.750000000000000000, -27.00000000000000355 ) ) ;
#5733=CARTESIAN_POINT ( 'NONE',  ( 11.18376618407357093, 5.549999997815051600, -27.00000000000000355 ) ) ;
#5736=CARTESIAN_POINT ( 'NONE',  ( -21.98271324694694329, 100.0000000000000000, -11.39207625356720222 ) ) ;
#5738=CARTESIAN_POINT ( 'NONE',  ( -22.16320288552370243, 99.50000000000001421, -10.86869938533413915 ) ) ;
#5741=ADVANCED_FACE ( 'NONE', ( #5067 ), #9942, .F. ) ;
#5742=ORIENTED_EDGE ( 'NONE', *, *, #6076, .F. ) ;
#5744=CARTESIAN_POINT ( 'NONE',  ( -20.42657152723830905, 99.50000000000000000, -10.54129411626120216 ) ) ;
#5745=CARTESIAN_POINT ( 'NONE',  ( -21.79668695291220715, 100.0000000000000000, -11.08213026643738353 ) ) ;
#5747=ORIENTED_EDGE ( 'NONE', *, *, #5317, .F. ) ;
#5748=CARTESIAN_POINT ( 'NONE',  ( 3.845216150098881513, 99.50000000000000000, -21.40922359334548020 ) ) ;
#5749=CARTESIAN_POINT ( 'NONE',  ( 3.973150561375555334, 99.50000000000000000, -22.87236500961342855 ) ) ;
#5751=ADVANCED_FACE ( 'NONE', ( #366 ), #6546, .T. ) ;
#5752=CARTESIAN_POINT ( 'NONE',  ( 3.873456569393397331, 100.0000000000000568, -22.53291374702356364 ) ) ;
#5753=CARTESIAN_POINT ( 'NONE',  ( 19.09188309203678102, 4.499999997815050001, 19.09188309203678813 ) ) ;
#5754=CARTESIAN_POINT ( 'NONE',  ( -20.45905772418405988, 99.50000000000000000, -10.59533404166311321 ) ) ;
#5755=CARTESIAN_POINT ( 'NONE',  ( -21.18972881998075763, 99.49999999999998579, -9.781869222470191971 ) ) ;
#5756=CARTESIAN_POINT ( 'NONE',  ( -15.07178375341841381, 99.50000000000000000, 16.66969090848992607 ) ) ;
#5757=CARTESIAN_POINT ( 'NONE',  ( -21.79668695291220715, 99.50000000000000000, -11.08213026643738353 ) ) ;
#5759=CARTESIAN_POINT ( 'NONE',  ( 2.940631318607589417, 99.50000000000000000, -23.77584808773673331 ) ) ;
#5763=CARTESIAN_POINT ( 'NONE',  ( -15.07178375341841381, 99.50000000000000000, 15.16157792772069790 ) ) ;
#5765=EDGE_CURVE ( 'NONE', #8029, #5243, #1328, .T. ) ;
#5766=CARTESIAN_POINT ( 'NONE',  ( -27.00000000000001421, 3.650000000000000799, 11.18376618407356382 ) ) ;
#5768=DIRECTION ( 'NONE',  ( 0.000000000000000000, 1.000000000000000000, 0.000000000000000000 ) ) ;
#5769=CARTESIAN_POINT ( 'NONE',  ( -20.91430522584054330, 99.99999999999998579, -10.19152558580213608 ) ) ;
#5770=ORIENTED_EDGE ( 'NONE', *, *, #2927, .F. ) ;
#5771=ORIENTED_EDGE ( 'NONE', *, *, #8962, .F. ) ;
#5772=CARTESIAN_POINT ( 'NONE',  ( -27.43301270000000969, 4.699999998907524734, 11.36312591709335784 ) ) ;
#5773=CARTESIAN_POINT ( 'NONE',  ( -15.91768310440539658, 99.50000000000002842, 15.18344740530786652 ) ) ;
#5775=CARTESIAN_POINT ( 'NONE',  ( -16.49816537377288128, 100.0000000000000000, 16.70951083495554101 ) ) ;
#5780=CARTESIAN_POINT ( 'NONE',  ( -22.33529725360453000, 99.49999999999997158, -10.20112572733487255 ) ) ;
#5781=CARTESIAN_POINT ( 'NONE',  ( 3.198738776810544415, 99.50000000000001421, -22.02447230026614022 ) ) ;
#5782=CARTESIAN_POINT ( 'NONE',  ( -17.94007301623892658, 100.0000000000000000, 17.49000340848992607 ) ) ;
#5783=CARTESIAN_POINT ( 'NONE',  ( -15.27171031718473770, 100.0000000000000284, 15.44886715306589764 ) ) ;
#5785=VECTOR ( 'NONE', #9803, 1000.000000000000114 ) ;
#5786=CARTESIAN_POINT ( 'NONE',  ( -4.959819536546781389E-15, 3.599999997815050534, 27.00000000000000355 ) ) ;
#5787=EDGE_CURVE ( 'NONE', #6736, #6706, #3952, .T. ) ;
#5788=CARTESIAN_POINT ( 'NONE',  ( -21.44539290152690114, 100.0000000000000000, -11.08070480119962298 ) ) ;
#5789=ORIENTED_EDGE ( 'NONE', *, *, #8577, .T. ) ;
#5790=ADVANCED_FACE ( 'NONE', ( #579 ), #6065, .T. ) ;
#5791=CARTESIAN_POINT ( 'NONE',  ( 0.000000000000000000, 100.0000000000000000, 0.000000000000000000 ) ) ;
#5794=CARTESIAN_POINT ( 'NONE',  ( 3.024867170474271116, 99.49999999999995737, -24.05477125543085748 ) ) ;
#5795=CARTESIAN_POINT ( 'NONE',  ( 7.812290123947159159, 99.49999999999998579, 21.17203503082402349 ) ) ;
#5796=ORIENTED_EDGE ( 'NONE', *, *, #5633, .T. ) ;
#5798=CARTESIAN_POINT ( 'NONE',  ( -11.18376618407358336, 4.349999997815050534, 26.99999999999999645 ) ) ;
#5800=CARTESIAN_POINT ( 'NONE',  ( -21.13452028402337035, 99.50000000000000000, -9.824917503107416294 ) ) ;
#5801=DIRECTION ( 'NONE',  ( -0.000000000000000000, -1.000000000000000000, -0.000000000000000000 ) ) ;
#5802=CARTESIAN_POINT ( 'NONE',  ( -21.93524539549613550, 99.49999999999998579, -11.03420246938663318 ) ) ;
#5803=CARTESIAN_POINT ( 'NONE',  ( 2.864934851235464208, 100.0000000000000000, -21.80148171563692827 ) ) ;
#5804=CARTESIAN_POINT ( 'NONE',  ( 0.000000000000000000, 100.0000000000000000, 0.000000000000000000 ) ) ;
#5805=EDGE_CURVE ( 'NONE', #9070, #3821, #5313, .T. ) ;
#5810=CARTESIAN_POINT ( 'NONE',  ( 2.958578797724396026, 99.50000000000000000, -23.36432507653281121 ) ) ;
#5811=CARTESIAN_POINT ( 'NONE',  ( 27.43301270000000258, 3.449999998907525178, 0.000000000000000000 ) ) ;
#5812=CARTESIAN_POINT ( 'NONE',  ( -27.00000000000000355, 0.3499999999999999778, -11.18376618407357270 ) ) ;
#5815=CARTESIAN_POINT ( 'NONE',  ( 0.000000000000000000, 100.0000000000000000, 0.000000000000000000 ) ) ;
#5816=CARTESIAN_POINT ( 'NONE',  ( -20.91264567078791714, 99.49999999999997158, -10.54226115003387676 ) ) ;
#5817=ORIENTED_EDGE ( 'NONE', *, *, #7794, .F. ) ;
#5818=CARTESIAN_POINT ( 'NONE',  ( -20.95972469638759250, 99.99999999999994316, -9.536167108072199028 ) ) ;
#5819=CARTESIAN_POINT ( 'NONE',  ( 1.679787559701184688E-15, 5.249999998907525445, -27.43301270000000258 ) ) ;
#5820=CARTESIAN_POINT ( 'NONE',  ( -15.37731512048643268, 99.50000000000000000, 15.34394520743122214 ) ) ;
#5821=VECTOR ( 'NONE', #10133, 1000.000000000000000 ) ;
#5822=CARTESIAN_POINT ( 'NONE',  ( 3.949943451936506644, 100.0000000000000000, -21.41482314084395711 ) ) ;
#5823=CARTESIAN_POINT ( 'NONE',  ( 9.482997300390421103, 99.50000000000000000, 20.28643943712827991 ) ) ;
#5825=FACE_OUTER_BOUND ( 'NONE', #9786, .T. ) ;
#5826=EDGE_LOOP ( 'NONE', ( #7838, #977, #6271, #1512 ) ) ;
#5828=ORIENTED_EDGE ( 'NONE', *, *, #69, .F. ) ;
#5830=CARTESIAN_POINT ( 'NONE',  ( 3.771794781161601939, 99.99999999999998579, -21.07813736596861176 ) ) ;
#5831=CARTESIAN_POINT ( 'NONE',  ( 3.356341388373609291, 99.99999999999998579, -21.61643044175963979 ) ) ;
#5832=CARTESIAN_POINT ( 'NONE',  ( 3.891852272358404807, 99.50000000000001421, -22.89765557720719968 ) ) ;
#5833=CARTESIAN_POINT ( 'NONE',  ( -15.15623813234777018, 100.0000000000000000, 16.19783826294960249 ) ) ;
#5834=CARTESIAN_POINT ( 'NONE',  ( 8.067960508813904141, 99.50000000000000000, 20.80952186068213905 ) ) ;
#5836=CARTESIAN_POINT ( 'NONE',  ( -21.65488089977124275, 99.99999999999997158, -11.10326233039539723 ) ) ;
#5837=ORIENTED_EDGE ( 'NONE', *, *, #6677, .T. ) ;
#5838=LINE ( 'NONE', #5045, #10077 ) ;
#5839=CARTESIAN_POINT ( 'NONE',  ( -19.39806930854667755, 0.6499999989075252449, -19.39806930854668110 ) ) ;
#5841=CARTESIAN_POINT ( 'NONE',  ( 4.122675185292913547, 99.49999999999997158, -22.83451320417363561 ) ) ;
#5842=CARTESIAN_POINT ( 'NONE',  ( 3.775125937424839151, 99.99999999999997158, -21.41825520325024712 ) ) ;
#5843=CARTESIAN_POINT ( 'NONE',  ( 2.859712287474666770, 99.50000000000000000, -22.17872625191749236 ) ) ;
#5844=CARTESIAN_POINT ( 'NONE',  ( -19.09188309203678813, 5.099999997815051422, 19.09188309203678457 ) ) ;
#5846=CARTESIAN_POINT ( 'NONE',  ( -21.52330660073277002, 100.0000000000000142, -9.647028226243550719 ) ) ;
#5847=CARTESIAN_POINT ( 'NONE',  ( 4.061354557346970040, 99.99999999999997158, -22.84864678426182039 ) ) ;
#5848=CARTESIAN_POINT ( 'NONE',  ( -21.79668695291220715, 100.0000000000000000, -11.08213026643738353 ) ) ;
#5849=PLANE ( 'NONE',  #1627 ) ;
#5856=CARTESIAN_POINT ( 'NONE',  ( 2.936358689207804851, 100.0000000000000000, -23.74786164940363875 ) ) ;
#5857=CARTESIAN_POINT ( 'NONE',  ( -11.36312591709335962, 3.699999998907525622, -27.43301270000000258 ) ) ;
#5858=ADVANCED_FACE ( 'NONE', ( #3104 ), #8701, .T. ) ;
#5859=LINE ( 'NONE', #1874, #6100 ) ;
#5861=CARTESIAN_POINT ( 'NONE',  ( 4.640952353770416927, 100.0000000000000000, -24.17064508475253604 ) ) ;
#5863=ORIENTED_EDGE ( 'NONE', *, *, #8659, .T. ) ;
#5864=CARTESIAN_POINT ( 'NONE',  ( -21.89277277937676303, 99.99999999999992895, -9.329958722595300458 ) ) ;
#5865=CARTESIAN_POINT ( 'NONE',  ( 9.676361905416719367, 99.50000000000000000, 21.63547735782115211 ) ) ;
#5866=CARTESIAN_POINT ( 'NONE',  ( 9.358681735871565266, 99.49999999999998579, 21.55373624431538815 ) ) ;
#5868=CARTESIAN_POINT ( 'NONE',  ( -16.35834224700816009, 100.0000000000000142, 16.43761959438736397 ) ) ;
#5869=CARTESIAN_POINT ( 'NONE',  ( 3.403200340195960738, 99.49999999999998579, -22.39827506699316118 ) ) ;
#5871=CARTESIAN_POINT ( 'NONE',  ( 0.000000000000000000, 100.0000000000000000, 0.000000000000000000 ) ) ;
#5873=CARTESIAN_POINT ( 'NONE',  ( 0.000000000000000000, 100.0000000000000000, -27.00000000000000355 ) ) ;
#5876=VERTEX_POINT ( 'NONE', #9485 ) ;
#5877=CARTESIAN_POINT ( 'NONE',  ( -22.33391032228853490, 100.0000000000000000, -10.55243757774135993 ) ) ;
#5878=CARTESIAN_POINT ( 'NONE',  ( 3.399971579580567393, 99.99999999999997158, -21.57509867787664248 ) ) ;
#5880=CARTESIAN_POINT ( 'NONE',  ( -15.19031985176477662, 99.99999999999998579, 15.56880617076518547 ) ) ;
#5881=EDGE_CURVE ( 'NONE', #5950, #3778, #3420, .T. ) ;
#5882=AXIS2_PLACEMENT_3D ( 'NONE', #4737, #6509, #8769 ) ;
#5883=EDGE_CURVE ( 'NONE', #3601, #519, #3931, .T. ) ;
#5884=ORIENTED_EDGE ( 'NONE', *, *, #9664, .T. ) ;
#5885=CARTESIAN_POINT ( 'NONE',  ( 8.122452352567329115, 99.50000000000000000, 21.04970292111833530 ) ) ;
#5886=LINE ( 'NONE', #8291, #7482 ) ;
#5889=VERTEX_POINT ( 'NONE', #10318 ) ;
#5890=CARTESIAN_POINT ( 'NONE',  ( 27.43301270000000258, 3.549999998907525267, 0.000000000000000000 ) ) ;
#5891=LINE ( 'NONE', #7505, #2223 ) ;
#5892=CARTESIAN_POINT ( 'NONE',  ( 3.750007936853901658, 99.50000000000001421, -22.95001988029826734 ) ) ;
#5893=CARTESIAN_POINT ( 'NONE',  ( 8.051038018032482313, 99.49999999999998579, 19.92675698219059299 ) ) ;
#5894=VERTEX_POINT ( 'NONE', #5657 ) ;
#5895=DIRECTION ( 'NONE',  ( -0.8547548816071318667, 0.000000000000000000, 0.5190318799156541374 ) ) ;
#5896=CARTESIAN_POINT ( 'NONE',  ( 27.00000000000000355, 4.599999997815050534, 0.000000000000000000 ) ) ;
#5897=CARTESIAN_POINT ( 'NONE',  ( -20.61566945723384592, 99.50000000000000000, -10.83949095114527594 ) ) ;
#5898=CARTESIAN_POINT ( 'NONE',  ( -21.08523985030068459, 100.0000000000000000, -9.874866134143449159 ) ) ;
#5899=CARTESIAN_POINT ( 'NONE',  ( 3.328702480760086235, 99.99999999999997158, -23.35145716610488975 ) ) ;
#5900=CARTESIAN_POINT ( 'NONE',  ( -21.30928386698190025, 99.50000000000000000, -11.02857376369709996 ) ) ;
#5901=CARTESIAN_POINT ( 'NONE',  ( 4.909381318607588973, 100.0000000000000000, -23.54377677363417121 ) ) ;
#5904=CARTESIAN_POINT ( 'NONE',  ( -14.83363727892122519, 100.0000000000000000, 15.50654517199034466 ) ) ;
#5906=CARTESIAN_POINT ( 'NONE',  ( -11.36312591709337383, 1.599999998907525534, 27.43301269999999548 ) ) ;
#5909=CARTESIAN_POINT ( 'NONE',  ( 21.82251602564102910, 99.50000000000000000, -0.5181290064102563875 ) ) ;
#5910=CARTESIAN_POINT ( 'NONE',  ( -11.18376618407356737, 4.049999997815050712, -27.00000000000000355 ) ) ;
#5913=CARTESIAN_POINT ( 'NONE',  ( 7.729958523985794194, 99.50000000000001421, 20.63140804260154937 ) ) ;
#5916=EDGE_CURVE ( 'NONE', #9964, #3939, #1571, .T. ) ;
#5917=CARTESIAN_POINT ( 'NONE',  ( -21.43094455402013310, 100.0000000000000000, -11.42705968398779426 ) ) ;
#5918=CARTESIAN_POINT ( 'NONE',  ( 4.446585460023182890, 100.0000000000000284, -21.79057454014859019 ) ) ;
#5919=CARTESIAN_POINT ( 'NONE',  ( -22.59920249870969045, 99.99999999999998579, -10.80326527670058567 ) ) ;
#5920=CARTESIAN_POINT ( 'NONE',  ( -20.97771390646102319, 100.0000000000000284, -10.03345247102482674 ) ) ;
#5921=ORIENTED_EDGE ( 'NONE', *, *, #9652, .F. ) ;
#5922=CARTESIAN_POINT ( 'NONE',  ( 4.887668416326221177, 100.0000000000000142, -23.70513093767710089 ) ) ;
#5924=ORIENTED_EDGE ( 'NONE', *, *, #3496, .F. ) ;
#5925=CARTESIAN_POINT ( 'NONE',  ( -22.28244091826395135, 99.50000000000000000, -10.68852969318427881 ) ) ;
#5926=CARTESIAN_POINT ( 'NONE',  ( 3.231466532446834350, 99.49999999999997158, -21.81145066552309686 ) ) ;
#5928=ADVANCED_FACE ( 'NONE', ( #9533 ), #4590, .T. ) ;
#5929=CARTESIAN_POINT ( 'NONE',  ( 3.269123371500344710, 99.50000000000001421, -23.64665713169964434 ) ) ;
#5930=CARTESIAN_POINT ( 'NONE',  ( 4.295198626299897349, 99.50000000000000000, -24.68029520312135006 ) ) ;
#5931=ORIENTED_EDGE ( 'NONE', *, *, #2318, .T. ) ;
#5932=B_SPLINE_CURVE_WITH_KNOTS ( 'NONE', 3,
 ( #301, #5003, #3490, #6533, #1033, #4179, #9721, #5897, #1858, #5754, #2655 ),
 .UNSPECIFIED., .F., .F.,
 ( 4, 1, 1, 1, 1, 1, 1, 1, 4 ),
 ( 0.000000000000000000, 0.09767211715481777246, 0.1989896052561311024, 0.3043518128873296535, 0.4150874769980872347, 0.5363819683935961979, 0.6738601886791220075, 0.8283091006677448798, 1.000000000000000000 ),
 .UNSPECIFIED. ) ;
#5936=CARTESIAN_POINT ( 'NONE',  ( -16.49092618789450526, 99.99999999999995737, 16.26472549871478179 ) ) ;
#5939=CARTESIAN_POINT ( 'NONE',  ( -21.51485068221570174, 100.0000000000000000, -11.09552232883975087 ) ) ;
#5940=AXIS2_PLACEMENT_3D ( 'NONE', #6258, #3180, #9458 ) ;
#5941=CARTESIAN_POINT ( 'NONE',  ( 9.834295043520187463, 100.0000000000000284, 21.14079655679390513 ) ) ;
#5942=ORIENTED_EDGE ( 'NONE', *, *, #5305, .T. ) ;
#5944=DIRECTION ( 'NONE',  ( 0.000000000000000000, 0.000000000000000000, 1.000000000000000000 ) ) ;
#5945=CARTESIAN_POINT ( 'NONE',  ( 11.36312591709336850, 4.999999998907526333, 27.43301269999999903 ) ) ;
#5946=CARTESIAN_POINT ( 'NONE',  ( 5.825495487346713297, 99.50000000000000000, 20.69456627699299744 ) ) ;
#5947=CARTESIAN_POINT ( 'NONE',  ( 3.293272160652527258, 99.49999999999997158, -24.41359064397622802 ) ) ;
#5948=CARTESIAN_POINT ( 'NONE',  ( 8.223467485077383898, 99.49999999999997158, 19.78581333328655134 ) ) ;
#5949=ADVANCED_FACE ( 'NONE', ( #8203 ), #8158, .T. ) ;
#5950=VERTEX_POINT ( 'NONE', #349 ) ;
#5951=CARTESIAN_POINT ( 'NONE',  ( 9.910564025336874749, 99.50000000000001421, 20.75459158945058036 ) ) ;
#5952=CARTESIAN_POINT ( 'NONE',  ( -19.09188309203678457, 2.499999997815050445, -19.09188309203678813 ) ) ;
#5953=CARTESIAN_POINT ( 'NONE',  ( -21.31369174262763622, 99.49999999999997158, -9.710155485040722567 ) ) ;
#5956=CARTESIAN_POINT ( 'NONE',  ( 4.901590909071964042, 100.0000000000000000, -23.62641080846013608 ) ) ;
#5959=EDGE_CURVE ( 'NONE', #2588, #9964, #5932, .T. ) ;
#5962=FACE_OUTER_BOUND ( 'NONE', #1040, .T. ) ;
#5963=CARTESIAN_POINT ( 'NONE',  ( -27.43301270000000258, 1.449999998907525178, -3.359575119402369376E-15 ) ) ;
#5964=LINE ( 'NONE', #8421, #1852 ) ;
#5967=LINE ( 'NONE', #4242, #4820 ) ;
#5968=CARTESIAN_POINT ( 'NONE',  ( 1.653273178848927064E-15, 1.000000000000000000, -27.00000000000000355 ) ) ;
#5969=CARTESIAN_POINT ( 'NONE',  ( 7.734522023158566739, 99.50000000000002842, 20.86022014488863618 ) ) ;
#5970=CARTESIAN_POINT ( 'NONE',  ( -22.10910773081910818, 99.50000000000001421, -11.33820747227609793 ) ) ;
#5974=CARTESIAN_POINT ( 'NONE',  ( -16.60513711880303234, 99.50000000000001421, 15.15667007515659748 ) ) ;
#5976=CARTESIAN_POINT ( 'NONE',  ( -21.80427673524616239, 100.0000000000000000, -9.663674634844889866 ) ) ;
#5977=ADVANCED_FACE ( 'NONE', ( #8303 ), #5054, .T. ) ;
#5978=PLANE ( 'NONE',  #4213 ) ;
#5980=EDGE_LOOP ( 'NONE', ( #6218, #10233, #6919, #10256 ) ) ;
#5981=CARTESIAN_POINT ( 'NONE',  ( -22.25406130147340633, 99.50000000000002842, -9.998337329044998611 ) ) ;
#5982=CARTESIAN_POINT ( 'NONE',  ( -5.039362679103552881E-15, 0.8499999989075253115, 27.43301270000000258 ) ) ;
#5983=CARTESIAN_POINT ( 'NONE',  ( 21.47055288461538325, 100.0000000000000000, -0.7081330128205128860 ) ) ;
#5984=CARTESIAN_POINT ( 'NONE',  ( -19.09188309203678813, 3.499999997815050445, 19.09188309203678457 ) ) ;
#5986=CARTESIAN_POINT ( 'NONE',  ( 4.835062408351179286, 99.50000000000000000, -21.79588013901878440 ) ) ;
#5989=VERTEX_POINT ( 'NONE', #8942 ) ;
#5990=B_SPLINE_CURVE_WITH_KNOTS ( 'NONE', 3,
 ( #6047, #5441, #9412, #5265, #6887, #9236, #8576, #4483, #8633, #10028, #2864, #7730, #6215, #8407, #2187, #2128, #1291, #9295, #7674 ),
 .UNSPECIFIED., .F., .F.,
 ( 4, 1, 1, 1, 1, 1, 1, 1, 1, 1, 1, 1, 1, 1, 1, 1, 4 ),
 ( 0.000000000000000000, 0.06533929434940796699, 0.1284421010879715219, 0.1894557237235162950, 0.2487158350925330053, 0.3070727012892665031, 0.3650088636856013702, 0.4229902474982629723, 0.4815891416229265420, 0.5404453987529589387, 0.6002338948610608238, 0.6608164219703346332, 0.7232441343194829786, 0.7881366429682739039, 0.8556965829275263724, 0.9259544997225339635, 1.000000000000000000 ),
 .UNSPECIFIED. ) ;
#5992=CARTESIAN_POINT ( 'NONE',  ( 1.679787559701184688E-15, 5.349999998907525089, -27.43301270000000258 ) ) ;
#5993=LINE ( 'NONE', #449, #6558 ) ;
#5995=CARTESIAN_POINT ( 'NONE',  ( 9.802580223201115217, 99.49999999999997158, 21.25247094773282086 ) ) ;
#5996=ORIENTED_EDGE ( 'NONE', *, *, #5048, .F. ) ;
#5997=CARTESIAN_POINT ( 'NONE',  ( -20.77412980915959650, 99.99999999999997158, -9.759484723497815040 ) ) ;
#5999=FACE_BOUND ( 'NONE', #7018, .T. ) ;
#6000=CARTESIAN_POINT ( 'NONE',  ( 4.154273145530666511, 100.0000000000000000, -22.82723029927519676 ) ) ;
#6001=ORIENTED_EDGE ( 'NONE', *, *, #9143, .T. ) ;
#6002=CARTESIAN_POINT ( 'NONE',  ( -16.35834224700816009, 100.0000000000000142, 16.43761959438736397 ) ) ;
#6003=CARTESIAN_POINT ( 'NONE',  ( -27.43301270000000969, 2.399999998907525356, 11.36312591709335784 ) ) ;
#6004=ORIENTED_EDGE ( 'NONE', *, *, #322, .T. ) ;
#6006=CARTESIAN_POINT ( 'NONE',  ( 3.311778287470797721, 99.50000000000000000, -21.22295334266859967 ) ) ;
#6009=CARTESIAN_POINT ( 'NONE',  ( 1.679787559701184688E-15, 3.649999998907525356, -27.43301270000000258 ) ) ;
#6010=DIRECTION ( 'NONE',  ( 0.000000000000000000, 0.000000000000000000, 1.000000000000000000 ) ) ;
#6013=CARTESIAN_POINT ( 'NONE',  ( 8.961048541867139505, 100.0000000000000142, 19.57961630251783092 ) ) ;
#6015=CARTESIAN_POINT ( 'NONE',  ( 8.051038018032482313, 99.99999999999998579, 19.92675698219059299 ) ) ;
#6016=CARTESIAN_POINT ( 'NONE',  ( -15.43596444985078975, 100.0000000000000284, 15.30036492734783593 ) ) ;
#6018=CARTESIAN_POINT ( 'NONE',  ( 2.852289972453743161, 100.0000000000000000, -22.14293542748032451 ) ) ;
#6021=CARTESIAN_POINT ( 'NONE',  ( -19.39806930854668465, 3.149999998907525356, 19.39806930854667755 ) ) ;
#6024=CARTESIAN_POINT ( 'NONE',  ( 4.232447118646125439, 99.99999999999998579, -21.54138831197867887 ) ) ;
#6025=CARTESIAN_POINT ( 'NONE',  ( 3.282077632710153292, 99.50000000000000000, -23.74569985055724786 ) ) ;
#6026=FACE_OUTER_BOUND ( 'NONE', #3290, .T. ) ;
#6031=CARTESIAN_POINT ( 'NONE',  ( -21.96365545856212265, 99.50000000000001421, -9.726658277667754149 ) ) ;
#6032=CARTESIAN_POINT ( 'NONE',  ( -15.07178375341841559, 99.50000000000001421, 15.16157792772069968 ) ) ;
#6033=CARTESIAN_POINT ( 'NONE',  ( 5.243816414761435674, 99.50000000000000000, -23.48558366465980995 ) ) ;
#6034=( BOUNDED_CURVE ( )  B_SPLINE_CURVE ( 2, ( #8268, #1924, #1096, #5812, #9003, #1975, #9103, #314, #5171 ),
 .UNSPECIFIED., .F., .T. ) 
 B_SPLINE_CURVE_WITH_KNOTS ( ( 3, 2, 2, 2, 3 ),
 ( 0.03571428571428571230, 0.05357142857142856845, 0.07142857142857142461, 0.08928571428571428770, 0.1071428571428571369 ),
 .UNSPECIFIED. ) 
 CURVE ( )  GEOMETRIC_REPRESENTATION_ITEM ( )  RATIONAL_B_SPLINE_CURVE ( ( 1.000000000000000000, 0.9238795325112867385, 1.000000000000000000, 0.9238795325112867385, 1.000000000000000000, 0.9238795325112867385, 1.000000000000000000, 0.9238795325112867385, 1.000000000000000000 ) ) 
 REPRESENTATION_ITEM ( '' )  );
#6038=CARTESIAN_POINT ( 'NONE',  ( -16.65546786808457469, 99.99999999999998579, 16.57295196178722918 ) ) ;
#6041=CARTESIAN_POINT ( 'NONE',  ( 11.18376618407357626, 1.249999997815050445, 27.00000000000000000 ) ) ;
#6042=CARTESIAN_POINT ( 'NONE',  ( 19.39806930854667399, 3.449999998907525622, 19.39806930854668465 ) ) ;
#6044=EDGE_CURVE ( 'NONE', #8336, #4987, #7407, .T. ) ;
#6045=CARTESIAN_POINT ( 'NONE',  ( 9.838488147574068421, 99.50000000000000000, 20.25735696016189280 ) ) ;
#6046=CARTESIAN_POINT ( 'NONE',  ( 7.486453019397995234, 99.50000000000000000, 23.81666162955709964 ) ) ;
#6047=CARTESIAN_POINT ( 'NONE',  ( 4.295198626299898237, 99.50000000000001421, -24.68029520312135361 ) ) ;
#6049=CARTESIAN_POINT ( 'NONE',  ( -16.37951318544778445, 99.49999999999997158, 15.41600550949200077 ) ) ;
#6051=ORIENTED_EDGE ( 'NONE', *, *, #9851, .F. ) ;
#6053=CARTESIAN_POINT ( 'NONE',  ( -19.39806930854668465, 1.649999998907525356, 19.39806930854667755 ) ) ;
#6056=EDGE_CURVE ( 'NONE', #4212, #6063, #3063, .T. ) ;
#6057=CARTESIAN_POINT ( 'NONE',  ( 9.357295078982289738, 99.50000000000004263, 20.12145687760884627 ) ) ;
#6058=CARTESIAN_POINT ( 'NONE',  ( 3.023131990384279710, 99.50000000000002842, -21.47496011329876708 ) ) ;
#6060=CARTESIAN_POINT ( 'NONE',  ( -11.36312591709335962, 4.499999998907525445, -27.43301270000000258 ) ) ;
#6061=CARTESIAN_POINT ( 'NONE',  ( -19.39806930854667755, 2.249999998907525001, -19.39806930854668110 ) ) ;
#6062=COLOUR_RGB ( '',0.8941176470588234615, 0.8941176470588234615, 0.8941176470588234615 ) ;
#6063=VERTEX_POINT ( 'NONE', #6162 ) ;
#6064=ORIENTED_EDGE ( 'NONE', *, *, #5142, .F. ) ;
#6065=PLANE ( 'NONE',  #5620 ) ;
#6067=CARTESIAN_POINT ( 'NONE',  ( 7.812290123947159159, 99.99999999999998579, 21.17203503082402349 ) ) ;
#6068=CARTESIAN_POINT ( 'NONE',  ( 3.664124300404482337, 100.0000000000000284, -24.27219056640880623 ) ) ;
#6069=VERTEX_POINT ( 'NONE', #3598 ) ;
#6072=EDGE_CURVE ( 'NONE', #369, #6174, #2010, .T. ) ;
#6075=CARTESIAN_POINT ( 'NONE',  ( 27.43301269999999548, 1.799999998907525267, 11.36312591709337738 ) ) ;
#6076=EDGE_CURVE ( 'NONE', #6802, #2896, #1187, .T. ) ;
#6077=CARTESIAN_POINT ( 'NONE',  ( -15.98658610793439117, 99.99999999999997158, 14.83943845084690949 ) ) ;
#6078=CARTESIAN_POINT ( 'NONE',  ( 27.00000000000000355, 0.8000000000000000444, 0.000000000000000000 ) ) ;
#6079=CARTESIAN_POINT ( 'NONE',  ( 2.859712287474666770, 99.50000000000000000, -22.17872625191749236 ) ) ;
#6081=EDGE_LOOP ( 'NONE', ( #9325, #9322, #2994, #8019 ) ) ;
#6083=CARTESIAN_POINT ( 'NONE',  ( -16.05266356869597644, 99.50000000000000000, 16.62382211633880047 ) ) ;
#6086=CARTESIAN_POINT ( 'NONE',  ( -22.28738277804067636, 99.99999999999994316, -10.06255608345902886 ) ) ;
#6090=CARTESIAN_POINT ( 'NONE',  ( 3.375079225685456041, 100.0000000000000000, -22.79123997459842954 ) ) ;
#6091=VECTOR ( 'NONE', #989, 1000.000000000000227 ) ;
#6092=VERTEX_POINT ( 'NONE', #9360 ) ;
#6093=CARTESIAN_POINT ( 'NONE',  ( 4.280752963211088336, 99.49999999999997158, -21.16602454745684270 ) ) ;
#6095=CARTESIAN_POINT ( 'NONE',  ( 24.91446314102564230, 99.50000000000000000, -1.581029647435897578 ) ) ;
#6097=CARTESIAN_POINT ( 'NONE',  ( -11.36312591709337383, 4.099999998907525089, 27.43301269999999548 ) ) ;
#6099=FACE_OUTER_BOUND ( 'NONE', #5382, .T. ) ;
#6100=VECTOR ( 'NONE', #214, 1000.000000000000000 ) ;
#6102=CARTESIAN_POINT ( 'NONE',  ( -21.49703851962343037, 99.99999999999997158, -9.300281078773625865 ) ) ;
#6103=CARTESIAN_POINT ( 'NONE',  ( 0.000000000000000000, 97.50000000000000000, 0.000000000000000000 ) ) ;
#6107=ORIENTED_EDGE ( 'NONE', *, *, #2496, .T. ) ;
#6108=CARTESIAN_POINT ( 'NONE',  ( -15.84348323231452049, 100.0000000000000000, 15.18005498687102772 ) ) ;
#6109=CARTESIAN_POINT ( 'NONE',  ( -27.43301270000000258, 1.499999998907525223, -11.36312591709336317 ) ) ;
#6113=CARTESIAN_POINT ( 'NONE',  ( 8.973011566395204142, 99.49999999999997158, 19.93291184930431115 ) ) ;
#6116=CARTESIAN_POINT ( 'NONE',  ( 4.773458297025112707, 99.50000000000001421, -24.02094923175124208 ) ) ;
#6117=CARTESIAN_POINT ( 'NONE',  ( 19.39806930854668110, 2.849999998907525089, -19.39806930854668110 ) ) ;
#6118=ORIENTED_EDGE ( 'NONE', *, *, #7406, .F. ) ;
#6119=CARTESIAN_POINT ( 'NONE',  ( 9.725694684612619767, 100.0000000000000000, 20.03234812723199454 ) ) ;
#6120=CARTESIAN_POINT ( 'NONE',  ( 3.023131990384279710, 99.50000000000002842, -21.47496011329876708 ) ) ;
#6122=CARTESIAN_POINT ( 'NONE',  ( -16.36254897777739004, 100.0000000000000142, 15.39785597259249350 ) ) ;
#6124=ORIENTED_EDGE ( 'NONE', *, *, #2448, .T. ) ;
#6126=CARTESIAN_POINT ( 'NONE',  ( -21.84904385032055174, 99.49999999999998579, -11.42736543092427404 ) ) ;
#6127=ORIENTED_EDGE ( 'NONE', *, *, #5166, .T. ) ;
#6129=CARTESIAN_POINT ( 'NONE',  ( 27.43301270000000258, 1.849999998907525312, 0.000000000000000000 ) ) ;
#6130=B_SPLINE_CURVE_WITH_KNOTS ( 'NONE', 3,
 ( #7774, #6090, #8448, #1278, #8619, #4579, #5310 ),
 .UNSPECIFIED., .F., .F.,
 ( 4, 1, 1, 1, 4 ),
 ( 0.000000000000000000, 0.2581490702850675056, 0.5078756004687992043, 0.7540928115589713432, 1.000000000000000000 ),
 .UNSPECIFIED. ) ;
#6131=ORIENTED_EDGE ( 'NONE', *, *, #2179, .F. ) ;
#6132=DIRECTION ( 'NONE',  ( -0.000000000000000000, 1.000000000000000000, -0.000000000000000000 ) ) ;
#6133=CARTESIAN_POINT ( 'NONE',  ( -4.959819536546781389E-15, 0.6000000000000000888, 27.00000000000000355 ) ) ;
#6134=AXIS2_PLACEMENT_3D ( 'NONE', #96, #882, #7950 ) ;
#6135=CARTESIAN_POINT ( 'NONE',  ( 9.446088657802272692, 100.0000000000000711, 20.22669104216016578 ) ) ;
#6137=CARTESIAN_POINT ( 'NONE',  ( -16.49419651247312046, 99.99999999999994316, 15.57134447358898477 ) ) ;
#6138=CARTESIAN_POINT ( 'NONE',  ( 8.067960508813904141, 99.50000000000000000, 20.80952186068213905 ) ) ;
#6140=ORIENTED_EDGE ( 'NONE', *, *, #780, .F. ) ;
#6142=CARTESIAN_POINT ( 'NONE',  ( -27.43301270000000258, 0.5999999989075253115, -11.36312591709336317 ) ) ;
#6144=CARTESIAN_POINT ( 'NONE',  ( -22.28244091826395135, 99.50000000000000000, -10.68852969318427881 ) ) ;
#6146=CARTESIAN_POINT ( 'NONE',  ( 5.207032889226773875, 100.0000000000000284, -23.83708953234284778 ) ) ;
#6147=LINE ( 'NONE', #2175, #6945 ) ;
#6148=EDGE_CURVE ( 'NONE', #6813, #3209, #9377, .T. ) ;
#6149=VECTOR ( 'NONE', #1875, 1000.000000000000000 ) ;
#6150=LINE ( 'NONE', #7551, #8329 ) ;
#6151=CARTESIAN_POINT ( 'NONE',  ( -16.92301558088953328, 100.0000000000000142, 15.88693424423437683 ) ) ;
#6158=CARTESIAN_POINT ( 'NONE',  ( 9.676361905416721143, 99.50000000000001421, 21.63547735782115566 ) ) ;
#6161=CARTESIAN_POINT ( 'NONE',  ( 8.857094148306096315, 100.0000000000000142, 19.57755665027156766 ) ) ;
#6162=CARTESIAN_POINT ( 'NONE',  ( 1.653273178848927064E-15, 3.400000000000000355, -27.00000000000000355 ) ) ;
#6163=CARTESIAN_POINT ( 'NONE',  ( -16.45635306197508996, 99.50000000000000000, 15.51056558312563105 ) ) ;
#6164=ORIENTED_EDGE ( 'NONE', *, *, #3035, .F. ) ;
#6166=CARTESIAN_POINT ( 'NONE',  ( -5.039362679103552881E-15, 2.549999998907525267, 27.43301270000000258 ) ) ;
#6167=ORIENTED_EDGE ( 'NONE', *, *, #5557, .T. ) ;
#6172=CARTESIAN_POINT ( 'NONE',  ( -16.81182640597031508, 99.50000000000000000, 16.36129326314865295 ) ) ;
#6173=CARTESIAN_POINT ( 'NONE',  ( 27.43301270000000258, 3.549999998907525267, 0.000000000000000000 ) ) ;
#6174=VERTEX_POINT ( 'NONE', #7731 ) ;
#6175=CARTESIAN_POINT ( 'NONE',  ( 8.857094148306096315, 100.0000000000000142, 19.57755665027156766 ) ) ;
#6176=LINE ( 'NONE', #685, #7831 ) ;
#6177=CARTESIAN_POINT ( 'NONE',  ( 3.311778287470797721, 99.50000000000000000, -21.22295334266859967 ) ) ;
#6178=B_SPLINE_SURFACE_WITH_KNOTS ( 'NONE', 3, 1, ( 
 ( #1757, #9817 ),
 ( #9139, #5842 ),
 ( #9717, #1030 ),
 ( #4999, #2704 ),
 ( #8199, #9037 ),
 ( #1131, #1854 ),
 ( #5050, #4323 ),
 ( #937, #4954 ),
 ( #8155, #983 ),
 ( #7357, #399 ),
 ( #2388, #6365 ),
 ( #3905, #7144 ),
 ( #8725, #1388 ),
 ( #4739, #606 ),
 ( #4581, #7092 ) ),
 .UNSPECIFIED., .F., .F., .F.,
 ( 4, 1, 1, 1, 1, 1, 1, 1, 1, 1, 1, 1, 4 ),
 ( 2, 2 ),
 ( 0.000000000000000000, 0.1166921615859537187, 0.2277195327244859735, 0.3361971884410420164, 0.4453256767247914527, 0.5018483577356800396, 0.5617326728321133666, 0.6243107931132723110, 0.6909729641497043273, 0.7615676753376537933, 0.8363829297815326136, 0.9156607463298391814, 0.9999999999999998890 ),
 ( 0.000000000000000000, 1.000000000000000000 ),
 .UNSPECIFIED. ) ;
#6179=CARTESIAN_POINT ( 'NONE',  ( -20.96643530928959365, 99.99999999999997158, -10.05541671241504886 ) ) ;
#6181=CARTESIAN_POINT ( 'NONE',  ( 4.633286773149219329, 100.0000000000000284, -21.44575434969419447 ) ) ;
#6183=CARTESIAN_POINT ( 'NONE',  ( 27.43301270000000258, 2.699999998907525178, -11.36312591709336139 ) ) ;
#6184=B_SPLINE_CURVE_WITH_KNOTS ( 'NONE', 3,
 ( #8734, #3237, #35, #3969, #3190, #6372, #3285, #4069, #4700, #7252, #2344, #6424, #3917, #9615, #5543, #723, #2399, #3087, #2449 ),
 .UNSPECIFIED., .F., .F.,
 ( 4, 1, 1, 1, 1, 1, 1, 1, 1, 1, 1, 1, 1, 1, 1, 1, 4 ),
 ( 0.000000000000000000, 0.06441145199513656494, 0.1272798026707614161, 0.1891796676955485867, 0.2501048626594916668, 0.3106574229659737063, 0.3727353219478334867, 0.4357106927796215445, 0.5001540812204312569, 0.5646670943021733224, 0.6273118991093056263, 0.6892359343283066542, 0.7500873997029591234, 0.8110709007071082999, 0.8723115105649058565, 0.9354174373376444862, 1.000000000000000000 ),
 .UNSPECIFIED. ) ;
#6185=ORIENTED_EDGE ( 'NONE', *, *, #3430, .T. ) ;
#6186=CARTESIAN_POINT ( 'NONE',  ( -15.70584307919286893, 99.50000000000000000, 14.84247401567675162 ) ) ;
#6188=CARTESIAN_POINT ( 'NONE',  ( -11.18376618407358336, 1.350000000000000089, 26.99999999999999645 ) ) ;
#6189=CARTESIAN_POINT ( 'NONE',  ( 2.852289972453743161, 100.0000000000000000, -22.14293542748032451 ) ) ;
#6190=ORIENTED_EDGE ( 'NONE', *, *, #9667, .T. ) ;
#6192=CARTESIAN_POINT ( 'NONE',  ( -15.49014769301379069, 99.99999999999997158, 16.56834637662448273 ) ) ;
#6195=ORIENTED_EDGE ( 'NONE', *, *, #2683, .F. ) ;
#6196=ORIENTED_EDGE ( 'NONE', *, *, #8045, .F. ) ;
#6198=DIRECTION ( 'NONE',  ( -0.9804671828129908340, 0.000000000000000000, 0.1966827481675937905 ) ) ;
#6201=CARTESIAN_POINT ( 'NONE',  ( 5.240996349771887886, 99.50000000000001421, -23.60769396873743631 ) ) ;
#6202=CARTESIAN_POINT ( 'NONE',  ( 0.000000000000000000, 100.0000000000000000, 0.000000000000000000 ) ) ;
#6203=APPLICATION_CONTEXT ( 'automotive_design' ) ;
#6206=CARTESIAN_POINT ( 'NONE',  ( -16.63177974700816009, 100.0000000000000000, 16.59747536361813403 ) ) ;
#6213=ORIENTED_EDGE ( 'NONE', *, *, #8716, .F. ) ;
#6215=CARTESIAN_POINT ( 'NONE',  ( 5.142436925601051811, 99.49999999999995737, -24.04117066426968563 ) ) ;
#6216=CARTESIAN_POINT ( 'NONE',  ( 3.282077632710153292, 100.0000000000000000, -23.74569985055724786 ) ) ;
#6217=CARTESIAN_POINT ( 'NONE',  ( -16.54512803120131181, 99.50000000000000000, 16.13427955854364626 ) ) ;
#6218=ORIENTED_EDGE ( 'NONE', *, *, #7457, .F. ) ;
#6219=CARTESIAN_POINT ( 'NONE',  ( -15.37731512048643268, 100.0000000000000000, 15.34394520743122214 ) ) ;
#6221=CARTESIAN_POINT ( 'NONE',  ( -27.43301270000000969, 0.7999999989075252671, 11.36312591709335784 ) ) ;
#6224=FACE_OUTER_BOUND ( 'NONE', #3706, .T. ) ;
#6226=CARTESIAN_POINT ( 'NONE',  ( 1.679787559701184688E-15, 5.249999998907525445, -27.43301270000000258 ) ) ;
#6227=CARTESIAN_POINT ( 'NONE',  ( 27.43301270000000258, 2.799999998907525267, -11.36312591709336139 ) ) ;
#6228=ORIENTED_EDGE ( 'NONE', *, *, #184, .T. ) ;
#6229=VECTOR ( 'NONE', #8281, 1000.000000000000000 ) ;
#6230=CARTESIAN_POINT ( 'NONE',  ( -15.55395551812965671, 100.0000000000000284, 16.59868653893595791 ) ) ;
#6232=CARTESIAN_POINT ( 'NONE',  ( 3.356341388373609291, 99.50000000000001421, -21.61643044175963979 ) ) ;
#6233=CARTESIAN_POINT ( 'NONE',  ( 3.286905236079108672, 100.0000000000000426, -23.77014634954566574 ) ) ;
#6235=CARTESIAN_POINT ( 'NONE',  ( -21.49703851962343037, 99.49999999999997158, -9.300281078773625865 ) ) ;
#6238=CARTESIAN_POINT ( 'NONE',  ( 19.39806930854667399, 1.749999998907525223, 19.39806930854668465 ) ) ;
#6241=VERTEX_POINT ( 'NONE', #5443 ) ;
#6243=CARTESIAN_POINT ( 'NONE',  ( -27.00000000000001421, 2.049999999999999822, 11.18376618407356382 ) ) ;
#6244=CARTESIAN_POINT ( 'NONE',  ( 9.114876806416853938, 100.0000000000000142, 19.97295714941878231 ) ) ;
#6245=ORIENTED_EDGE ( 'NONE', *, *, #5881, .F. ) ;
#6246=CARTESIAN_POINT ( 'NONE',  ( -16.41302370085497131, 99.99999999999994316, 15.45185748370271206 ) ) ;
#6247=CARTESIAN_POINT ( 'NONE',  ( 8.337740814200648387, 99.50000000000002842, 20.10843643765939248 ) ) ;
#6249=ORIENTED_EDGE ( 'NONE', *, *, #7410, .T. ) ;
#6251=ORIENTED_EDGE ( 'NONE', *, *, #1973, .T. ) ;
#6252=EDGE_LOOP ( 'NONE', ( #1382, #10087, #8181, #7130 ) ) ;
#6254=CARTESIAN_POINT ( 'NONE',  ( 1.679787559701184688E-15, 2.049999998907525711, -27.43301270000000258 ) ) ;
#6255=CARTESIAN_POINT ( 'NONE',  ( -21.94169572595625795, 99.50000000000000000, -9.715372641902229489 ) ) ;
#6257=CARTESIAN_POINT ( 'NONE',  ( -19.09188309203678457, 3.500000000000000000, -19.09188309203678813 ) ) ;
#6258=CARTESIAN_POINT ( 'NONE',  ( 0.000000000000000000, 100.0000000000000000, 0.000000000000000000 ) ) ;
#6260=VECTOR ( 'NONE', #6764, 1000.000000000000000 ) ;
#6262=EDGE_CURVE ( 'NONE', #2471, #8902, #10306, .T. ) ;
#6263=CARTESIAN_POINT ( 'NONE',  ( 4.259295290443009918, 99.50000000000002842, -24.34414156132068996 ) ) ;
#6264=CARTESIAN_POINT ( 'NONE',  ( 11.18376618407357626, 0.6500000000000001332, 27.00000000000000000 ) ) ;
#6266=EDGE_LOOP ( 'NONE', ( #8434, #7945, #5263, #6393 ) ) ;
#6267=CARTESIAN_POINT ( 'NONE',  ( 9.063633472794011325, 99.49999999999998579, 19.59517414759687526 ) ) ;
#6270=B_SPLINE_SURFACE_WITH_KNOTS ( 'NONE', 3, 1, ( 
 ( #4603, #7795 ),
 ( #626, #3663 ),
 ( #4493, #10038 ),
 ( #2197, #2874 ),
 ( #6006, #1249 ),
 ( #3825, #4439 ),
 ( #9199, #3714 ),
 ( #6058, #9425 ),
 ( #467, #6897 ),
 ( #9307, #2139 ),
 ( #7741, #574 ),
 ( #3768, #734 ),
 ( #9673, #8053 ),
 ( #6335, #8889 ),
 ( #6432, #7211 ) ),
 .UNSPECIFIED., .F., .F., .F.,
 ( 4, 1, 1, 1, 1, 1, 1, 1, 1, 1, 1, 1, 4 ),
 ( 2, 2 ),
 ( 0.000000000000000000, 0.08963690308348271074, 0.1775767702671464110, 0.2649576542713044658, 0.3533131777157214604, 0.4402865524342069459, 0.5245518675747646853, 0.6066224975438009315, 0.6889424263984335051, 0.7698335385027974542, 0.8475882324521423206, 0.9236428641877653112, 1.000000000000000000 ),
 ( 0.000000000000000000, 1.000000000000000000 ),
 .UNSPECIFIED. ) ;
#6271=ORIENTED_EDGE ( 'NONE', *, *, #8965, .T. ) ;
#6272=FACE_OUTER_BOUND ( 'NONE', #3230, .T. ) ;
#6273=CARTESIAN_POINT ( 'NONE',  ( 9.778118981323553172, 99.49999999999998579, 20.11889122584574352 ) ) ;
#6276=ORIENTED_EDGE ( 'NONE', *, *, #911, .T. ) ;
#6277=CARTESIAN_POINT ( 'NONE',  ( -14.76042637754942177, 99.50000000000000000, 16.05242888258284140 ) ) ;
#6278=CARTESIAN_POINT ( 'NONE',  ( -27.43301270000000258, 3.099999998907525089, -11.36312591709336317 ) ) ;
#6279=VERTEX_POINT ( 'NONE', #6216 ) ;
#6284=CARTESIAN_POINT ( 'NONE',  ( -16.91659681606879317, 99.50000000000000000, 15.78485274883190392 ) ) ;
#6285=CARTESIAN_POINT ( 'NONE',  ( -11.36312591709335962, 3.799999998907525711, -27.43301270000000258 ) ) ;
#6286=CARTESIAN_POINT ( 'NONE',  ( -15.19031985176477662, 99.99999999999995737, 15.56880617076518547 ) ) ;
#6287=CARTESIAN_POINT ( 'NONE',  ( 26.99999999999999645, 3.749999997815050445, 11.18376618407358691 ) ) ;
#6288=CARTESIAN_POINT ( 'NONE',  ( 2.901827748664965068, 99.49999999999998579, -21.68759887446373469 ) ) ;
#6290=CARTESIAN_POINT ( 'NONE',  ( -4.959819536546781389E-15, 3.799999999999999822, 27.00000000000000355 ) ) ;
#6292=CARTESIAN_POINT ( 'NONE',  ( 4.118246196500586542, 99.49999999999998579, -21.10643963665684453 ) ) ;
#6293=ORIENTED_EDGE ( 'NONE', *, *, #385, .T. ) ;
#6295=CARTESIAN_POINT ( 'NONE',  ( 27.43301270000000258, 5.099999998907525978, -11.36312591709336139 ) ) ;
#6297=CARTESIAN_POINT ( 'NONE',  ( -15.56505537928961047, 99.99999999999998579, 14.87309967080592088 ) ) ;
#6299=CARTESIAN_POINT ( 'NONE',  ( -19.09188309203678457, 2.700000000000000178, -19.09188309203678813 ) ) ;
#6300=CARTESIAN_POINT ( 'NONE',  ( 8.829292973371666520, 99.49999999999998579, 19.92220432019063736 ) ) ;
#6302=VERTEX_POINT ( 'NONE', #9521 ) ;
#6304=CARTESIAN_POINT ( 'NONE',  ( -15.30604604128650692, 99.50000000000000000, 15.41317891555018349 ) ) ;
#6305=CARTESIAN_POINT ( 'NONE',  ( 8.081885929396888102, 99.50000000000001421, 20.89785832093561169 ) ) ;
#6309=CARTESIAN_POINT ( 'NONE',  ( -27.43301270000000969, 3.099999998907525089, 11.36312591709335784 ) ) ;
#6310=CARTESIAN_POINT ( 'NONE',  ( -21.13452028402337035, 99.50000000000000000, -9.824917503107416294 ) ) ;
#6311=B_SPLINE_CURVE_WITH_KNOTS ( 'NONE', 3,
 ( #6483, #7058, #10314, #3151, #9529, #3245, #101, #2511, #2353, #9573, #837, #2305, #4078, #5550, #5702, #1714, #8107, #8005, #4910 ),
 .UNSPECIFIED., .F., .F.,
 ( 4, 1, 1, 1, 1, 1, 1, 1, 1, 1, 1, 1, 1, 1, 1, 1, 4 ),
 ( 0.000000000000000000, 0.06455295689170470474, 0.1273249605695649933, 0.1891299628201091876, 0.2499617887110622549, 0.3104215510145779122, 0.3717966107350694216, 0.4346754705585744727, 0.4991966429079077727, 0.5636107885140392293, 0.6264421791528413941, 0.6882713145562978641, 0.7491215306807221808, 0.8100115732567139126, 0.8716292230916812267, 0.9349778748807419104, 1.000000000000000000 ),
 .UNSPECIFIED. ) ;
#6312=AXIS2_PLACEMENT_3D ( 'NONE', #1349, #1243, #675 ) ;
#6313=VECTOR ( 'NONE', #188, 1000.000000000000000 ) ;
#6315=DIRECTION ( 'NONE',  ( 0.3918949146621865109, 0.000000000000000000, 0.9200099868272720860 ) ) ;
#6316=ORIENTED_EDGE ( 'NONE', *, *, #8891, .T. ) ;
#6321=CARTESIAN_POINT ( 'NONE',  ( -16.07368679829020763, 99.50000000000000000, 17.11560437002838952 ) ) ;
#6322=DIRECTION ( 'NONE',  ( -0.000000000000000000, 1.000000000000000000, -0.000000000000000000 ) ) ;
#6324=ADVANCED_FACE ( 'NONE', ( #1559 ), #10360, .F. ) ;
#6325=CARTESIAN_POINT ( 'NONE',  ( -16.49187002848391970, 99.50000000000001421, 16.71294888518108124 ) ) ;
#6327=( BOUNDED_CURVE ( )  B_SPLINE_CURVE ( 2, ( #7926, #7188, #3358, #4102, #9739 ),
 .UNSPECIFIED., .F., .T. ) 
 B_SPLINE_CURVE_WITH_KNOTS ( ( 3, 2, 3 ),
 ( 0.000000000000000000, 0.01785714285714285615, 0.03571428571428571230 ),
 .UNSPECIFIED. ) 
 CURVE ( )  GEOMETRIC_REPRESENTATION_ITEM ( )  RATIONAL_B_SPLINE_CURVE ( ( 1.000000000000000000, 0.9238795325112867385, 1.000000000000000000, 0.9238795325112867385, 1.000000000000000000 ) ) 
 REPRESENTATION_ITEM ( '' )  );
#6328=CARTESIAN_POINT ( 'NONE',  ( -22.29247428061501779, 99.50000000000000000, -10.66603791136541624 ) ) ;
#6329=CARTESIAN_POINT ( 'NONE',  ( -16.36254897777739004, 100.0000000000000142, 15.39785597259249350 ) ) ;
#6330=CARTESIAN_POINT ( 'NONE',  ( 11.36312591709336139, 3.699999998907525622, -27.43301270000000258 ) ) ;
#6333=B_SPLINE_CURVE_WITH_KNOTS ( 'NONE', 3,
 ( #8375, #7426, #1981, #9060, #5969, #8961, #5913, #9946, #5071, #5023, #1053, #4245, #8273, #422, #318, #1779, #1205, #3562, #5125 ),
 .UNSPECIFIED., .F., .F.,
 ( 4, 1, 1, 1, 1, 1, 1, 1, 1, 1, 1, 1, 1, 1, 1, 1, 4 ),
 ( 0.000000000000000000, 0.06839333837245492598, 0.1346519561570838353, 0.1985335841112251809, 0.2613354512981445610, 0.3228799447584090876, 0.3842093944964607433, 0.4462111754260434937, 0.5089246482083435996, 0.5715029624870164859, 0.6324491702983550123, 0.6923675070709934820, 0.7521785462597534444, 0.8119602890481165680, 0.8728645645504365946, 0.9355733815441056311, 1.000000000000000000 ),
 .UNSPECIFIED. ) ;
#6335=CARTESIAN_POINT ( 'NONE',  ( 2.847408871211157155, 99.50000000000001421, -22.10537533382872510 ) ) ;
#6337=CARTESIAN_POINT ( 'NONE',  ( -21.18296228862668329, 99.50000000000002842, -10.95406920104765724 ) ) ;
#6338=CARTESIAN_POINT ( 'NONE',  ( -19.09188309203678813, 1.899999997815050579, 19.09188309203678457 ) ) ;
#6339=DIRECTION ( 'NONE',  ( 0.5074415416931677969, 0.000000000000000000, 0.8616861851997287269 ) ) ;
#6340=CARTESIAN_POINT ( 'NONE',  ( 3.320270046935387853, 99.99999999999998579, -23.88810568987970484 ) ) ;
#6341=CARTESIAN_POINT ( 'NONE',  ( 3.552835461024879127, 99.50000000000000000, -21.47801279722421697 ) ) ;
#6342=CARTESIAN_POINT ( 'NONE',  ( 19.09188309203678102, 3.900000000000000355, 19.09188309203678813 ) ) ;
#6344=CARTESIAN_POINT ( 'NONE',  ( 3.861186820804014097, 99.50000000000004263, -21.07288982789904708 ) ) ;
#6345=ORIENTED_EDGE ( 'NONE', *, *, #4146, .T. ) ;
#6347=CARTESIAN_POINT ( 'NONE',  ( -19.39806930854668465, 4.749999998907525445, 19.39806930854667755 ) ) ;
#6348=EDGE_CURVE ( 'NONE', #4897, #9070, #8098, .T. ) ;
#6350=EDGE_CURVE ( 'NONE', #393, #4830, #3421, .T. ) ;
#6351=CARTESIAN_POINT ( 'NONE',  ( 26.99999999999999645, 3.950000000000000178, 11.18376618407358691 ) ) ;
#6355=CARTESIAN_POINT ( 'NONE',  ( -15.76250887235353737, 99.49999999999998579, 16.65066592061022277 ) ) ;
#6357=CARTESIAN_POINT ( 'NONE',  ( -20.74358258379034936, 99.99999999999992895, -9.818556592845180120 ) ) ;
#6358=CARTESIAN_POINT ( 'NONE',  ( 1.679787559701184688E-15, 3.649999998907525356, -27.43301270000000258 ) ) ;
#6359=CARTESIAN_POINT ( 'NONE',  ( 3.097283534322414766, 99.50000000000002842, -24.18405864774921454 ) ) ;
#6360=B_SPLINE_SURFACE_WITH_KNOTS ( 'NONE', 3, 1, ( 
 ( #3012, #6189 ),
 ( #6079, #5298 ),
 ( #4829, #8906 ),
 ( #2529, #1733 ),
 ( #5721, #805 ),
 ( #1636, #9545 ),
 ( #997, #4969 ),
 ( #2572, #2369 ),
 ( #3999, #7182 ),
 ( #165, #5568 ),
 ( #6452, #6500 ) ),
 .UNSPECIFIED., .F., .F., .F.,
 ( 4, 1, 1, 1, 1, 1, 1, 1, 4 ),
 ( 2, 2 ),
 ( 0.000000000000000000, 0.1243175037779491315, 0.2437391319546453605, 0.3610119291759345539, 0.4796059399169178006, 0.5994854737745749507, 0.7252340722053824962, 0.8585022233306516259, 1.000000000000000000 ),
 ( 0.000000000000000000, 1.000000000000000000 ),
 .UNSPECIFIED. ) ;
#6363=CARTESIAN_POINT ( 'NONE',  ( 1.653273178848927064E-15, 1.599999997815050312, -27.00000000000000355 ) ) ;
#6364=CARTESIAN_POINT ( 'NONE',  ( -16.76168403648438243, 100.0000000000000284, 16.44483764528499847 ) ) ;
#6365=CARTESIAN_POINT ( 'NONE',  ( 4.363164797760430424, 100.0000000000000000, -21.67376679147534446 ) ) ;
#6368=LINE ( 'NONE', #9562, #1280 ) ;
#6372=CARTESIAN_POINT ( 'NONE',  ( -22.35673484330673944, 100.0000000000000142, -10.41320610523044721 ) ) ;
#6373=LINE ( 'NONE', #2346, #7654 ) ;
#6374=DIRECTION ( 'NONE',  ( -0.9985315370676780544, 0.000000000000000000, 0.05417351272771728232 ) ) ;
#6375=CARTESIAN_POINT ( 'NONE',  ( 1.679787559701184688E-15, 3.749999998907525445, -27.43301270000000258 ) ) ;
#6377=EDGE_CURVE ( 'NONE', #1366, #4987, #9807, .T. ) ;
#6380=CARTESIAN_POINT ( 'NONE',  ( 3.275092494823534928, 99.50000000000000000, -23.54688978826290580 ) ) ;
#6382=CARTESIAN_POINT ( 'NONE',  ( -21.07003209069497984, 99.99999999999998579, -11.28505157174820361 ) ) ;
#6383=CARTESIAN_POINT ( 'NONE',  ( -4.959819536546781389E-15, 1.999999997815050445, 27.00000000000000355 ) ) ;
#6384=( BOUNDED_CURVE ( )  B_SPLINE_CURVE ( 2, ( #6696, #5130, #9791, #8382, #5074, #3626, #9211, #2043, #1934 ),
 .UNSPECIFIED., .F., .T. ) 
 B_SPLINE_CURVE_WITH_KNOTS ( ( 3, 2, 2, 2, 3 ),
 ( 0.8214285714285713969, 0.8392857142857143016, 0.8571428571428570953, 0.8750000000000000000, 0.8928571428571429047 ),
 .UNSPECIFIED. ) 
 CURVE ( )  GEOMETRIC_REPRESENTATION_ITEM ( )  RATIONAL_B_SPLINE_CURVE ( ( 1.000000000000000000, 0.9238795325112867385, 1.000000000000000000, 0.9238795325112867385, 1.000000000000000000, 0.9238795325112867385, 1.000000000000000000, 0.9238795325112867385, 1.000000000000000000 ) ) 
 REPRESENTATION_ITEM ( '' )  );
#6385=CARTESIAN_POINT ( 'NONE',  ( -15.18657300206754179, 99.99999999999997158, 16.26161032743331347 ) ) ;
#6386=CARTESIAN_POINT ( 'NONE',  ( 9.342627931057743140, 100.0000000000000000, 21.59831790269294771 ) ) ;
#6387=CARTESIAN_POINT ( 'NONE',  ( 3.317038232150706367, 99.99999999999998579, -21.66195598387956878 ) ) ;
#6391=CARTESIAN_POINT ( 'NONE',  ( 4.232798786556307036, 99.50000000000000000, -24.34936571594186105 ) ) ;
#6393=ORIENTED_EDGE ( 'NONE', *, *, #2486, .T. ) ;
#6395=EDGE_CURVE ( 'NONE', #6501, #6993, #4486, .T. ) ;
#6396=CARTESIAN_POINT ( 'NONE',  ( 27.43301270000000258, 1.199999998907525178, -11.36312591709336139 ) ) ;
#6398=CARTESIAN_POINT ( 'NONE',  ( -15.34367147589386349, 99.50000000000004263, 16.87599331055909602 ) ) ;
#6399=CARTESIAN_POINT ( 'NONE',  ( -19.39806930854668465, 0.7499999989075252227, 19.39806930854667755 ) ) ;
#6400=CARTESIAN_POINT ( 'NONE',  ( 3.079986699855593473E-15, 85.00000000000000000, 25.15000000000000213 ) ) ;
#6402=CARTESIAN_POINT ( 'NONE',  ( -20.89884294283097432, 99.50000000000001421, -10.47119744953613640 ) ) ;
#6403=EDGE_CURVE ( 'NONE', #9797, #2280, #978, .T. ) ;
#6407=ADVANCED_FACE ( 'NONE', ( #1069, #3374 ), #9026, .T. ) ;
#6408=CARTESIAN_POINT ( 'NONE',  ( 27.43301270000000258, 1.099999998907525312, -11.36312591709336139 ) ) ;
#6409=CARTESIAN_POINT ( 'NONE',  ( 3.350143586568126164, 100.0000000000000142, -24.46212657588250394 ) ) ;
#6410=CARTESIAN_POINT ( 'NONE',  ( -11.18376618407356737, 0.8499999978150503122, -27.00000000000000355 ) ) ;
#6412=CARTESIAN_POINT ( 'NONE',  ( -16.45635306197508996, 100.0000000000000000, 15.51056558312563105 ) ) ;
#6414=CARTESIAN_POINT ( 'NONE',  ( -22.58826642033182353, 99.49999999999998579, -9.883148377786627137 ) ) ;
#6416=B_SPLINE_CURVE_WITH_KNOTS ( 'NONE', 3,
 ( #3874, #7629, #526, #2199, #8532, #8477, #10268, #1468, #6116, #3100, #5454 ),
 .UNSPECIFIED., .F., .F.,
 ( 4, 1, 1, 1, 1, 1, 1, 1, 4 ),
 ( 0.000000000000000000, 0.1514666391271576040, 0.2940212016997327260, 0.4289076436562640482, 0.5568069201790899481, 0.6759213874835566793, 0.7888117551744765477, 0.8972989960681465593, 1.000000000000000000 ),
 .UNSPECIFIED. ) ;
#6419=CARTESIAN_POINT ( 'NONE',  ( 4.523042264738025509, 99.50000000000001421, -24.25177047807976294 ) ) ;
#6420=CARTESIAN_POINT ( 'NONE',  ( 0.000000000000000000, 0.000000000000000000, 0.000000000000000000 ) ) ;
#6421=CARTESIAN_POINT ( 'NONE',  ( 9.445361748092775400, 99.50000000000001421, 19.75398588445988324 ) ) ;
#6424=CARTESIAN_POINT ( 'NONE',  ( -22.25406130147340633, 100.0000000000000284, -9.998337329044998611 ) ) ;
#6425=EDGE_LOOP ( 'NONE', ( #9031, #4626, #8374, #5837 ) ) ;
#6428=CARTESIAN_POINT ( 'NONE',  ( -16.34436021381890924, 100.0000000000000000, 15.38072013554846151 ) ) ;
#6429=CARTESIAN_POINT ( 'NONE',  ( 11.36312591709336850, 4.999999998907526333, 27.43301269999999903 ) ) ;
#6430=ORIENTED_EDGE ( 'NONE', *, *, #9006, .T. ) ;
#6431=CARTESIAN_POINT ( 'NONE',  ( 3.207968951880266761, 99.49999999999998579, -22.92616835434091627 ) ) ;
#6432=CARTESIAN_POINT ( 'NONE',  ( 2.852289972453743161, 99.50000000000000000, -22.14293542748032451 ) ) ;
#6434=CARTESIAN_POINT ( 'NONE',  ( -21.07003209069497984, 99.49999999999998579, -11.28505157174820361 ) ) ;
#6435=CARTESIAN_POINT ( 'NONE',  ( -27.00000000000000355, 1.799999997815050490, -3.306546357697854128E-15 ) ) ;
#6437=DIRECTION ( 'NONE',  ( 0.000000000000000000, 0.000000000000000000, 1.000000000000000000 ) ) ;
#6438=CARTESIAN_POINT ( 'NONE',  ( 3.296462644833695776, 100.0000000000000142, -23.81854410834942115 ) ) ;
#6439=DIRECTION ( 'NONE',  ( 0.3368601548094422582, 0.000000000000000000, -0.9415546909775122097 ) ) ;
#6443=CARTESIAN_POINT ( 'NONE',  ( 3.428794695218988053, 99.50000000000001421, -24.07607503615978572 ) ) ;
#6445=VECTOR ( 'NONE', #9731, 1000.000000000000000 ) ;
#6446=EDGE_LOOP ( 'NONE', ( #8823, #5161, #2845, #335 ) ) ;
#6448=CARTESIAN_POINT ( 'NONE',  ( 27.43301270000000258, 4.249999998907525445, 0.000000000000000000 ) ) ;
#6449=CARTESIAN_POINT ( 'NONE',  ( -15.45548338988150938, 99.49999999999997158, 16.93306818456458984 ) ) ;
#6450=B_SPLINE_CURVE_WITH_KNOTS ( 'NONE', 3,
 ( #3502, #9884, #264, #6688, #1773, #9835, #2618 ),
 .UNSPECIFIED., .F., .F.,
 ( 4, 1, 1, 1, 4 ),
 ( 0.000000000000000000, 0.2676680225848128147, 0.5230972062070123885, 0.7658030722156558001, 1.000000000000000000 ),
 .UNSPECIFIED. ) ;
#6451=CARTESIAN_POINT ( 'NONE',  ( 11.18376618407356915, 3.350000000000000089, -27.00000000000000355 ) ) ;
#6452=CARTESIAN_POINT ( 'NONE',  ( 3.411785164761435674, 99.50000000000000000, -22.76693382491622231 ) ) ;
#6455=CARTESIAN_POINT ( 'NONE',  ( -21.12798922145720582, 99.50000000000001421, -10.90888695829967325 ) ) ;
#6457=ORIENTED_EDGE ( 'NONE', *, *, #6715, .T. ) ;
#6458=CARTESIAN_POINT ( 'NONE',  ( 8.429066232339796017, 99.50000000000000000, 19.67794530653910101 ) ) ;
#6459=ORIENTED_EDGE ( 'NONE', *, *, #8191, .T. ) ;
#6460=CARTESIAN_POINT ( 'NONE',  ( -11.36312591709335962, 2.099999998907525089, -27.43301270000000258 ) ) ;
#6461=CARTESIAN_POINT ( 'NONE',  ( 2.950788281418828429, 100.0000000000000142, -23.82341910423825837 ) ) ;
#6465=CARTESIAN_POINT ( 'NONE',  ( -22.43208371148383762, 99.50000000000000000, -9.654966607469265938 ) ) ;
#6466=CARTESIAN_POINT ( 'NONE',  ( 4.772556553149396308, 99.99999999999997158, -24.49721679606612312 ) ) ;
#6469=VECTOR ( 'NONE', #1629, 1000.000000000000000 ) ;
#6471=CARTESIAN_POINT ( 'NONE',  ( -20.63200021313574695, 99.50000000000000000, -10.19493994959453431 ) ) ;
#6472=FACE_OUTER_BOUND ( 'NONE', #7703, .T. ) ;
#6476=EDGE_CURVE ( 'NONE', #1992, #9410, #10362, .T. ) ;
#6478=CARTESIAN_POINT ( 'NONE',  ( -18.01369080470046313, 99.50000000000000000, 17.15556831233607937 ) ) ;
#6480=CARTESIAN_POINT ( 'NONE',  ( -11.36312591709337561, 3.299999998907525267, 27.43301269999999548 ) ) ;
#6481=ORIENTED_EDGE ( 'NONE', *, *, #3915, .F. ) ;
#6482=CARTESIAN_POINT ( 'NONE',  ( 3.949943451936506644, 99.50000000000000000, -21.41482314084395711 ) ) ;
#6483=CARTESIAN_POINT ( 'NONE',  ( -20.96643530928959365, 99.99999999999997158, -10.05541671241504886 ) ) ;
#6485=CARTESIAN_POINT ( 'NONE',  ( 0.000000000000000000, 0.000000000000000000, 0.000000000000000000 ) ) ;
#6486=CARTESIAN_POINT ( 'NONE',  ( -27.43301270000000258, 4.749999998907525445, -3.359575119402369376E-15 ) ) ;
#6487=CARTESIAN_POINT ( 'NONE',  ( -15.11611088805441661, 99.50000000000000000, 16.06180012866831319 ) ) ;
#6488=CARTESIAN_POINT ( 'NONE',  ( 3.286905236079108672, 99.50000000000004263, -23.77014634954566574 ) ) ;
#6492=CARTESIAN_POINT ( 'NONE',  ( 3.320270046935387853, 99.49999999999998579, -23.88810568987970484 ) ) ;
#6496=CARTESIAN_POINT ( 'NONE',  ( 27.43301270000000258, 5.049999998907525267, 0.000000000000000000 ) ) ;
#6498=CARTESIAN_POINT ( 'NONE',  ( 5.825495487346713297, 100.0000000000000000, 20.69456627699299744 ) ) ;
#6499=CARTESIAN_POINT ( 'NONE',  ( 27.43301270000000258, 0.2499999989075252504, 0.000000000000000000 ) ) ;
#6500=CARTESIAN_POINT ( 'NONE',  ( 3.411785164761435674, 100.0000000000000000, -22.76693382491622231 ) ) ;
#6501=VERTEX_POINT ( 'NONE', #2162 ) ;
#6503=EDGE_LOOP ( 'NONE', ( #4719, #9007, #8399, #9849 ) ) ;
#6504=CARTESIAN_POINT ( 'NONE',  ( 27.43301270000000258, 5.099999998907525089, -11.36312591709336139 ) ) ;
#6506=EDGE_CURVE ( 'NONE', #6069, #7989, #3064, .T. ) ;
#6507=CARTESIAN_POINT ( 'NONE',  ( -21.71039561923405969, 99.50000000000004263, -11.44438725057713313 ) ) ;
#6509=DIRECTION ( 'NONE',  ( 0.2901787468363226652, 0.000000000000000000, 0.9569724629708534769 ) ) ;
#6510=MECHANICAL_DESIGN_GEOMETRIC_PRESENTATION_REPRESENTATION('',(#663),#1647);
#6511=CARTESIAN_POINT ( 'NONE',  ( -22.59920249870969045, 99.49999999999998579, -10.80326527670058567 ) ) ;
#6512=CARTESIAN_POINT ( 'NONE',  ( 8.149445629999579666, 100.0000000000000284, 20.33980848884064230 ) ) ;
#6514=ORIENTED_EDGE ( 'NONE', *, *, #4043, .F. ) ;
#6516=CARTESIAN_POINT ( 'NONE',  ( -20.69312081029678296, 99.49999999999997158, -9.926742041671966277 ) ) ;
#6517=EDGE_CURVE ( 'NONE', #9173, #4212, #2644, .T. ) ;
#6518=DIRECTION ( 'NONE',  ( -0.000000000000000000, -1.000000000000000000, -0.000000000000000000 ) ) ;
#6520=ORIENTED_EDGE ( 'NONE', *, *, #4909, .F. ) ;
#6523=ADVANCED_FACE ( 'NONE', ( #5145 ), #8617, .T. ) ;
#6524=CARTESIAN_POINT ( 'NONE',  ( -22.27115127098604574, 100.0000000000000000, -10.71048520281369676 ) ) ;
#6525=CARTESIAN_POINT ( 'NONE',  ( 8.564701892180647036, 100.0000000000000000, 19.97971282122689018 ) ) ;
#6529=CARTESIAN_POINT ( 'NONE',  ( 2.971063225226878046, 99.50000000000000000, -23.91837856253154015 ) ) ;
#6530=CARTESIAN_POINT ( 'NONE',  ( 8.051038018032482313, 99.99999999999994316, 19.92675698219059299 ) ) ;
#6531=CARTESIAN_POINT ( 'NONE',  ( -20.52076770522338833, 100.0000000000000000, -10.69798695537560462 ) ) ;
#6532=CARTESIAN_POINT ( 'NONE',  ( 11.18376618407356915, 0.7499999978150503344, -27.00000000000000355 ) ) ;
#6533=CARTESIAN_POINT ( 'NONE',  ( -20.97746206809550884, 99.50000000000000000, -11.22189255051946688 ) ) ;
#6536=CARTESIAN_POINT ( 'NONE',  ( -16.11976138926855739, 99.49999999999997158, 16.60078749809536447 ) ) ;
#6537=CARTESIAN_POINT ( 'NONE',  ( -21.44539290152690114, 99.50000000000000000, -11.08070480119962298 ) ) ;
#6543=MANIFOLD_SOLID_BREP ( 'Thread1', #4135 ) ;
#6544=CARTESIAN_POINT ( 'NONE',  ( 19.09188309203678102, 3.100000000000000533, 19.09188309203678813 ) ) ;
#6545=DIRECTION ( 'NONE',  ( -0.000000000000000000, -1.000000000000000000, -0.000000000000000000 ) ) ;
#6546=CYLINDRICAL_SURFACE ( 'NONE', #2940, 27.00000000000000355 ) ;
#6547=CARTESIAN_POINT ( 'NONE',  ( 21.82251602564102910, 99.50000000000000000, -0.5181290064102563875 ) ) ;
#6548=CARTESIAN_POINT ( 'NONE',  ( -20.89145576992255116, 99.49999999999997158, -10.33073932272468198 ) ) ;
#6550=ORIENTED_EDGE ( 'NONE', *, *, #3753, .F. ) ;
#6552=CARTESIAN_POINT ( 'NONE',  ( 9.547662139763570366, 99.49999999999997158, 20.94662037603165672 ) ) ;
#6555=CARTESIAN_POINT ( 'NONE',  ( -22.59920249870969045, 99.49999999999998579, -10.80326527670058567 ) ) ;
#6556=CARTESIAN_POINT ( 'NONE',  ( -22.69331084068295112, 99.99999999999998579, -10.43328931840349050 ) ) ;
#6557=CARTESIAN_POINT ( 'NONE',  ( -4.959819536546781389E-15, 5.199999997815050179, 27.00000000000000355 ) ) ;
#6558=VECTOR ( 'NONE', #9974, 1000.000000000000000 ) ;
#6559=EDGE_CURVE ( 'NONE', #7809, #4244, #3947, .T. ) ;
#6561=ORIENTED_EDGE ( 'NONE', *, *, #8169, .T. ) ;
#6562=CARTESIAN_POINT ( 'NONE',  ( -22.35642768247353729, 99.99999999999994316, -10.34293228154892752 ) ) ;
#6563=CARTESIAN_POINT ( 'NONE',  ( 3.673732336774000018, 99.50000000000000000, -21.43557726391590279 ) ) ;
#6573=ORIENTED_EDGE ( 'NONE', *, *, #8246, .T. ) ;
#6574=CARTESIAN_POINT ( 'NONE',  ( 3.817429849879703241, 99.99999999999995737, -22.92346308580664171 ) ) ;
#6575=CARTESIAN_POINT ( 'NONE',  ( 8.429066232339796017, 99.50000000000000000, 19.67794530653910101 ) ) ;
#6576=CARTESIAN_POINT ( 'NONE',  ( 9.723125805078051798, 99.50000000000000000, 21.50134635983626907 ) ) ;
#6577=CARTESIAN_POINT ( 'NONE',  ( -19.09188309203678457, 4.899999997815050357, -19.09188309203678813 ) ) ;
#6578=DIRECTION ( 'NONE',  ( 0.9682498375925071565, 0.000000000000000000, 0.2499845035238856816 ) ) ;
#6579=CARTESIAN_POINT ( 'NONE',  ( -21.24882413972086681, 99.50000000000002842, -9.742484589929601313 ) ) ;
#6581=CARTESIAN_POINT ( 'NONE',  ( -21.51485068221570174, 100.0000000000000000, -11.09552232883975087 ) ) ;
#6584=VERTEX_POINT ( 'NONE', #67 ) ;
#6586=( BOUNDED_CURVE ( )  B_SPLINE_CURVE ( 2, ( #2177, #8452, #1282, #7607, #3642, #4471, #5376, #501, #2119 ),
 .UNSPECIFIED., .F., .F. ) 
 B_SPLINE_CURVE_WITH_KNOTS ( ( 3, 2, 2, 2, 3 ),
 ( 0.1785714285714285754, 0.1964285714285714246, 0.2142857142857142738, 0.2321428571428571508, 0.2500000000000000000 ),
 .UNSPECIFIED. ) 
 CURVE ( )  GEOMETRIC_REPRESENTATION_ITEM ( )  RATIONAL_B_SPLINE_CURVE ( ( 1.000000000000000000, 0.9238795325112867385, 1.000000000000000000, 0.9238795325112867385, 1.000000000000000000, 0.9238795325112867385, 1.000000000000000000, 0.9238795325112867385, 1.000000000000000000 ) ) 
 REPRESENTATION_ITEM ( '' )  );
#6587=CARTESIAN_POINT ( 'NONE',  ( -14.83571502646304197, 100.0000000000000284, 16.32397075880403392 ) ) ;
#6588=CARTESIAN_POINT ( 'NONE',  ( 3.016803124593948393, 100.0000000000000142, -23.20507807535735978 ) ) ;
#6589=CARTESIAN_POINT ( 'NONE',  ( 1.679787559701184688E-15, 1.249999998907525223, -27.43301270000000258 ) ) ;
#6593=CARTESIAN_POINT ( 'NONE',  ( 0.000000000000000000, 5.000000000000004441, -27.00000000000000355 ) ) ;
#6594=CARTESIAN_POINT ( 'NONE',  ( -20.99557965837879081, 99.99999999999994316, -10.74478602187354959 ) ) ;
#6595=VECTOR ( 'NONE', #7613, 1000.000000000000000 ) ;
#6597=CARTESIAN_POINT ( 'NONE',  ( -21.79396932678589849, 99.99999999999994316, -9.306975108219608828 ) ) ;
#6598=CARTESIAN_POINT ( 'NONE',  ( 2.950788281418828429, 100.0000000000000142, -23.82341910423825837 ) ) ;
#6599=DIRECTION ( 'NONE',  ( -0.9572638942369904314, 0.000000000000000000, 0.2892158999609669712 ) ) ;
#6600=CARTESIAN_POINT ( 'NONE',  ( -21.56977948371741505, 99.99999999999995737, -11.44450812306045329 ) ) ;
#6601=CARTESIAN_POINT ( 'NONE',  ( 4.049441352997683374, 100.0000000000000000, -21.43849541167161732 ) ) ;
#6602=CARTESIAN_POINT ( 'NONE',  ( -16.61132721736409934, 100.0000000000000142, 16.61681399495993716 ) ) ;
#6605=CARTESIAN_POINT ( 'NONE',  ( 5.098880966732203035, 100.0000000000000000, -24.13374913903897223 ) ) ;
#6607=ORIENTED_EDGE ( 'NONE', *, *, #5305, .F. ) ;
#6609=CARTESIAN_POINT ( 'NONE',  ( -22.34867803760930727, 99.49999999999998579, -10.48295844864103721 ) ) ;
#6610=CARTESIAN_POINT ( 'NONE',  ( 3.198738776810544415, 99.99999999999998579, -22.02447230026614022 ) ) ;
#6611=CARTESIAN_POINT ( 'NONE',  ( -22.05902956123343017, 99.50000000000000000, -10.96257574645357558 ) ) ;
#6612=FACE_OUTER_BOUND ( 'NONE', #8876, .T. ) ;
#6613=CARTESIAN_POINT ( 'NONE',  ( 8.337740814200648387, 99.50000000000002842, 20.10843643765939248 ) ) ;
#6614=VECTOR ( 'NONE', #1781, 1000.000000000000114 ) ;
#6616=CARTESIAN_POINT ( 'NONE',  ( -19.09188309203678813, 2.699999997815051067, 19.09188309203678457 ) ) ;
#6617=ORIENTED_EDGE ( 'NONE', *, *, #7012, .T. ) ;
#6620=ADVANCED_FACE ( 'NONE', ( #8810 ), #5522, .T. ) ;
#6621=VECTOR ( 'NONE', #4170, 1000.000000000000000 ) ;
#6622=CARTESIAN_POINT ( 'NONE',  ( 4.061354557346970040, 99.49999999999997158, -22.84864678426182039 ) ) ;
#6623=CARTESIAN_POINT ( 'NONE',  ( 7.978247738654171251, 99.50000000000000000, 20.00924965157036794 ) ) ;
#6625=CARTESIAN_POINT ( 'NONE',  ( 9.766630880609509902, 99.50000000000002842, 21.37293705761699059 ) ) ;
#6626=CARTESIAN_POINT ( 'NONE',  ( 26.99999999999999645, 4.549999997815051600, 11.18376618407358691 ) ) ;
#6627=DIRECTION ( 'NONE',  ( -0.3923379498508065000, 0.000000000000000000, -0.9198211419112228837 ) ) ;
#6628=CARTESIAN_POINT ( 'NONE',  ( 0.000000000000000000, 87.00000000000001421, 0.000000000000000000 ) ) ;
#6629=CYLINDRICAL_SURFACE ( 'NONE', #1217, 27.00000000000000355 ) ;
#6630=CARTESIAN_POINT ( 'NONE',  ( -22.28244091826395135, 100.0000000000000000, -10.68852969318427881 ) ) ;
#6631=CARTESIAN_POINT ( 'NONE',  ( 4.773458297025112707, 99.50000000000001421, -24.02094923175124208 ) ) ;
#6633=CARTESIAN_POINT ( 'NONE',  ( -16.07368679829020763, 99.50000000000000000, 17.11560437002838952 ) ) ;
#6636=CARTESIAN_POINT ( 'NONE',  ( 3.044406660298407452, 100.0000000000000000, -23.15442635585071685 ) ) ;
#6638=CARTESIAN_POINT ( 'NONE',  ( -19.39806930854668465, 2.349999998907525534, 19.39806930854667755 ) ) ;
#6641=VECTOR ( 'NONE', #4884, 1000.000000000000000 ) ;
#6642=CYLINDRICAL_SURFACE ( 'NONE', #1129, 27.00000000000000355 ) ;
#6644=ORIENTED_EDGE ( 'NONE', *, *, #8582, .T. ) ;
#6646=CARTESIAN_POINT ( 'NONE',  ( -21.20585021321354802, 99.50000000000005684, -9.381045134209834657 ) ) ;
#6648=CARTESIAN_POINT ( 'NONE',  ( 1.679787559701184688E-15, 4.449999998907525622, -27.43301270000000258 ) ) ;
#6649=CARTESIAN_POINT ( 'NONE',  ( 9.468852706215191262, 99.50000000000000000, 21.22967007823213237 ) ) ;
#6651=VECTOR ( 'NONE', #4702, 1000.000000000000000 ) ;
#6652=CARTESIAN_POINT ( 'NONE',  ( 4.295198626299898237, 100.0000000000000142, -24.68029520312135361 ) ) ;
#6653=CARTESIAN_POINT ( 'NONE',  ( 8.540544597724410991, 99.50000000000000000, 19.98924338346217766 ) ) ;
#6654=CARTESIAN_POINT ( 'NONE',  ( 9.526533506306627430, 99.50000000000000000, 21.03094362668609207 ) ) ;
#6655=CARTESIAN_POINT ( 'NONE',  ( -21.66466628782423243, 100.0000000000000142, -9.640935998098070669 ) ) ;
#6656=VERTEX_POINT ( 'NONE', #6547 ) ;
#6659=CARTESIAN_POINT ( 'NONE',  ( -21.43094455402013310, 100.0000000000000000, -11.42705968398779426 ) ) ;
#6660=DIRECTION ( 'NONE',  ( -0.000000000000000000, 1.000000000000000000, -0.000000000000000000 ) ) ;
#6662=CARTESIAN_POINT ( 'NONE',  ( 4.401614252286283779, 100.0000000000000568, -24.65974366035752396 ) ) ;
#6663=CARTESIAN_POINT ( 'NONE',  ( 8.540544597724410991, 99.50000000000000000, 19.98924338346217766 ) ) ;
#6664=LINE ( 'NONE', #9859, #4828 ) ;
#6665=PLANE ( 'NONE',  #797 ) ;
#6666=CARTESIAN_POINT ( 'NONE',  ( 9.766630880609509902, 100.0000000000000284, 21.37293705761699059 ) ) ;
#6668=CARTESIAN_POINT ( 'NONE',  ( -5.039362679103552881E-15, 3.349999998907525534, 27.43301270000000258 ) ) ;
#6669=DIRECTION ( 'NONE',  ( 0.9569724629708533659, 0.000000000000000000, -0.2901787468363226097 ) ) ;
#6670=CARTESIAN_POINT ( 'NONE',  ( 3.434779879277784609, 99.50000000000001421, -23.17575050830969374 ) ) ;
#6671=CARTESIAN_POINT ( 'NONE',  ( 7.726884419709978857, 99.99999999999994316, 20.74516479202295471 ) ) ;
#6673=CARTESIAN_POINT ( 'NONE',  ( 3.403200340195960738, 99.49999999999998579, -22.39827506699316118 ) ) ;
#6674=CARTESIAN_POINT ( 'NONE',  ( 11.18376618407357626, 5.249999997815050889, 27.00000000000000000 ) ) ;
#6676=FACE_OUTER_BOUND ( 'NONE', #4564, .T. ) ;
#6677=EDGE_CURVE ( 'NONE', #834, #8336, #755, .T. ) ;
#6678=CARTESIAN_POINT ( 'NONE',  ( -22.16320288552370243, 99.50000000000001421, -10.86869938533413915 ) ) ;
#6680=PLANE ( 'NONE',  #958 ) ;
#6685=CARTESIAN_POINT ( 'NONE',  ( 2.928963527206765338, 99.99999999999997158, -23.52685633767685758 ) ) ;
#6686=CARTESIAN_POINT ( 'NONE',  ( -19.39806930854668465, 3.149999998907525356, 19.39806930854667755 ) ) ;
#6687=CARTESIAN_POINT ( 'NONE',  ( 11.36312591709336139, 0.4999999989075251672, -27.43301270000000258 ) ) ;
#6688=CARTESIAN_POINT ( 'NONE',  ( -20.66709314808276332, 100.0000000000000284, -10.01107456535036455 ) ) ;
#6689=CARTESIAN_POINT ( 'NONE',  ( 0.000000000000000000, 87.00000000000001421, 0.000000000000000000 ) ) ;
#6691=EDGE_CURVE ( 'NONE', #2647, #2426, #4155, .T. ) ;
#6692=DIRECTION ( 'NONE',  ( -0.2910078965507976179, 0.000000000000000000, -0.9567206510497618943 ) ) ;
#6694=CARTESIAN_POINT ( 'NONE',  ( 27.43301270000000258, 5.049999998907525267, 0.000000000000000000 ) ) ;
#6695=DIRECTION ( 'NONE',  ( -0.000000000000000000, -1.000000000000000000, -0.000000000000000000 ) ) ;
#6696=CARTESIAN_POINT ( 'NONE',  ( -4.959819536546781389E-15, 4.599999999999999645, 27.00000000000000355 ) ) ;
#6697=DIRECTION ( 'NONE',  ( -0.000000000000000000, 1.000000000000000000, -0.000000000000000000 ) ) ;
#6698=DIRECTION ( 'NONE',  ( -0.000000000000000000, 1.000000000000000000, -0.000000000000000000 ) ) ;
#6699=DIRECTION ( 'NONE',  ( 0.000000000000000000, 0.000000000000000000, 1.000000000000000000 ) ) ;
#6700=EDGE_LOOP ( 'NONE', ( #8924, #1351, #10136, #3003 ) ) ;
#6701=EDGE_CURVE ( 'NONE', #341, #2896, #5967, .T. ) ;
#6702=( BOUNDED_SURFACE ( )  B_SPLINE_SURFACE ( 1, 2, ( 
 ( #5018, #9781, #4190, #6687, #8214, #9880, #5119, #8317, #1149, #8478, #3718, #5400, #4442, #10042, #7688, #4496, #7798, #4662, #3875, #6900, #3771, #8592, #682, #1306, #7010, #3101, #1469, #2142, #1414, #470, #8533, #10096, #5279, #9428, #2878, #6846, #2254, #3828, #6061, #10213, #3047, #6957, #9371, #527, #9252, #2085, #629, #10160, #2935, #6227, #6117, #7745, #2200, #3666, #9310, #5343, #1358, #5455, #4550, #1252, #8645, #578, #7852, #2993, #6173, #4606, #7061, #7630, #10269, #6285, #9482, #2308, #5508, #939, #790, #841, #2460, #8110, #8745, #4081, #154, #8894, #9576, #8846, #7904, #5604, #3982, #2356, #6486, #7117, #3930, #9677, #891, #10317, #7263, #105, #4032, #3295, #5553, #48, #3201 ),
 ( #7316, #3341, #2515, #6532, #1620, #1719, #1569, #4133, #4913, #7168, #2408, #4759, #5706, #3463, #9719, #2561, #8697, #3155, #7214, #1518, #3248, #7957, #1672, #4711, #6435, #737, #6338, #9532, #6383, #8794, #4814, #8009, #9628, #5655, #4867, #8057, #1961, #1133, #5952, #5157, #9039, #9768, #1032, #7460, #6729, #2607, #5002, #8302, #200, #985, #1186, #4277, #402, #300, #4227, #9142, #8941, #3489, #3433, #9092, #8355, #1082, #4177, #7563, #3383, #7359, #1810, #8989, #1910, #4377, #3597, #8202, #8254, #9870, #6780, #5798, #4326, #9979, #5753, #6626, #5896, #4956, #2654, #7405, #248, #3540, #6577, #9819, #9925, #7510, #5844, #348, #2760, #6674, #1759, #1857, #2706, #5053, #8157, #5102, #7050 ) ),
 .UNSPECIFIED., .F., .F., .T. ) 
 B_SPLINE_SURFACE_WITH_KNOTS ( ( 2, 2 ),
 ( 3, 2, 2, 2, 2, 2, 2, 2, 2, 2, 2, 2, 2, 2, 2, 2, 2, 2, 2, 2, 2, 2, 2, 2, 2, 2, 2, 2, 2, 2, 2, 2, 2, 2, 2, 2, 2, 2, 2, 2, 2, 2, 2, 2, 2, 2, 2, 2, 2, 2, 3 ),
 ( 0.000000000000000000, 1.000000000000000000 ),
 ( 0.000000000000000000, 0.01785714285714285615, 0.03571428571428571230, 0.05357142857142856845, 0.07142857142857142461, 0.08928571428571428770, 0.1071428571428571369, 0.1250000000000000000, 0.1428571428571428492, 0.1607142857142857262, 0.1785714285714285754, 0.1964285714285714246, 0.2142857142857142738, 0.2321428571428571508, 0.2500000000000000000, 0.2678571428571428492, 0.2857142857142856984, 0.3035714285714285476, 0.3214285714285714524, 0.3392857142857143016, 0.3571428571428571508, 0.3750000000000000000, 0.3928571428571428492, 0.4107142857142856984, 0.4285714285714285476, 0.4464285714285714524, 0.4642857142857143016, 0.4821428571428571508, 0.5000000000000000000, 0.5178571428571429047, 0.5357142857142856984, 0.5535714285714286031, 0.5714285714285713969, 0.5892857142857143016, 0.6071428571428570953, 0.6250000000000000000, 0.6428571428571429047, 0.6607142857142856984, 0.6785714285714286031, 0.6964285714285713969, 0.7142857142857143016, 0.7321428571428570953, 0.7500000000000000000, 0.7678571428571429047, 0.7857142857142856984, 0.8035714285714286031, 0.8214285714285713969, 0.8392857142857143016, 0.8571428571428570953, 0.8750000000000000000, 0.8928571428571429047 ),
 .UNSPECIFIED. ) 
 GEOMETRIC_REPRESENTATION_ITEM ( )  RATIONAL_B_SPLINE_SURFACE ( (
 ( 1.000000000000000000, 0.9238795325112867385, 1.000000000000000000, 0.9238795325112867385, 1.000000000000000000, 0.9238795325112867385, 1.000000000000000000, 0.9238795325112867385, 1.000000000000000000, 0.9238795325112867385, 1.000000000000000000, 0.9238795325112867385, 1.000000000000000000, 0.9238795325112867385, 1.000000000000000000, 0.9238795325112867385, 1.000000000000000000, 0.9238795325112867385, 1.000000000000000000, 0.9238795325112867385, 1.000000000000000000, 0.9238795325112867385, 1.000000000000000000, 0.9238795325112867385, 1.000000000000000000, 0.9238795325112867385, 1.000000000000000000, 0.9238795325112867385, 1.000000000000000000, 0.9238795325112867385, 1.000000000000000000, 0.9238795325112867385, 1.000000000000000000, 0.9238795325112867385, 1.000000000000000000, 0.9238795325112867385, 1.000000000000000000, 0.9238795325112867385, 1.000000000000000000, 0.9238795325112867385, 1.000000000000000000, 0.9238795325112867385, 1.000000000000000000, 0.9238795325112867385, 1.000000000000000000, 0.9238795325112867385, 1.000000000000000000, 0.9238795325112867385, 1.000000000000000000, 0.9238795325112867385, 1.000000000000000000, 0.9238795325112867385, 1.000000000000000000, 0.9238795325112867385, 1.000000000000000000, 0.9238795325112867385, 1.000000000000000000, 0.9238795325112867385, 1.000000000000000000, 0.9238795325112867385, 1.000000000000000000, 0.9238795325112867385, 1.000000000000000000, 0.9238795325112867385, 1.000000000000000000, 0.9238795325112867385, 1.000000000000000000, 0.9238795325112867385, 1.000000000000000000, 0.9238795325112867385, 1.000000000000000000, 0.9238795325112867385, 1.000000000000000000, 0.9238795325112867385, 1.000000000000000000, 0.9238795325112867385, 1.000000000000000000, 0.9238795325112867385, 1.000000000000000000, 0.9238795325112867385, 1.000000000000000000, 0.9238795325112867385, 1.000000000000000000, 0.9238795325112867385, 1.000000000000000000, 0.9238795325112867385, 1.000000000000000000, 0.9238795325112867385, 1.000000000000000000, 0.9238795325112867385, 1.000000000000000000, 0.9238795325112867385, 1.000000000000000000, 0.9238795325112867385, 1.000000000000000000, 0.9238795325112867385, 1.000000000000000000, 0.9238795325112867385, 1.000000000000000000, 0.9238795325112867385, 1.000000000000000000),
 ( 1.000000000000000000, 0.9238795325112867385, 1.000000000000000000, 0.9238795325112867385, 1.000000000000000000, 0.9238795325112867385, 1.000000000000000000, 0.9238795325112867385, 1.000000000000000000, 0.9238795325112867385, 1.000000000000000000, 0.9238795325112867385, 1.000000000000000000, 0.9238795325112867385, 1.000000000000000000, 0.9238795325112867385, 1.000000000000000000, 0.9238795325112867385, 1.000000000000000000, 0.9238795325112867385, 1.000000000000000000, 0.9238795325112867385, 1.000000000000000000, 0.9238795325112867385, 1.000000000000000000, 0.9238795325112867385, 1.000000000000000000, 0.9238795325112867385, 1.000000000000000000, 0.9238795325112867385, 1.000000000000000000, 0.9238795325112867385, 1.000000000000000000, 0.9238795325112867385, 1.000000000000000000, 0.9238795325112867385, 1.000000000000000000, 0.9238795325112867385, 1.000000000000000000, 0.9238795325112867385, 1.000000000000000000, 0.9238795325112867385, 1.000000000000000000, 0.9238795325112867385, 1.000000000000000000, 0.9238795325112867385, 1.000000000000000000, 0.9238795325112867385, 1.000000000000000000, 0.9238795325112867385, 1.000000000000000000, 0.9238795325112867385, 1.000000000000000000, 0.9238795325112867385, 1.000000000000000000, 0.9238795325112867385, 1.000000000000000000, 0.9238795325112867385, 1.000000000000000000, 0.9238795325112867385, 1.000000000000000000, 0.9238795325112867385, 1.000000000000000000, 0.9238795325112867385, 1.000000000000000000, 0.9238795325112867385, 1.000000000000000000, 0.9238795325112867385, 1.000000000000000000, 0.9238795325112867385, 1.000000000000000000, 0.9238795325112867385, 1.000000000000000000, 0.9238795325112867385, 1.000000000000000000, 0.9238795325112867385, 1.000000000000000000, 0.9238795325112867385, 1.000000000000000000, 0.9238795325112867385, 1.000000000000000000, 0.9238795325112867385, 1.000000000000000000, 0.9238795325112867385, 1.000000000000000000, 0.9238795325112867385, 1.000000000000000000, 0.9238795325112867385, 1.000000000000000000, 0.9238795325112867385, 1.000000000000000000, 0.9238795325112867385, 1.000000000000000000, 0.9238795325112867385, 1.000000000000000000, 0.9238795325112867385, 1.000000000000000000, 0.9238795325112867385, 1.000000000000000000, 0.9238795325112867385, 1.000000000000000000) ) ) 
 REPRESENTATION_ITEM ( '' )  SURFACE ( )  );
#6703=CARTESIAN_POINT ( 'NONE',  ( 0.000000000000000000, 99.50000000000000000, 0.000000000000000000 ) ) ;
#6704=ADVANCED_FACE ( 'NONE', ( #1775, #316 ), #8372, .F. ) ;
#6706=VERTEX_POINT ( 'NONE', #7476 ) ;
#6707=CARTESIAN_POINT ( 'NONE',  ( -21.16695614262292580, 100.0000000000000000, -11.33496398805607441 ) ) ;
#6708=CARTESIAN_POINT ( 'NONE',  ( 3.411785164761435674, 99.50000000000000000, -22.76693382491622231 ) ) ;
#6710=CARTESIAN_POINT ( 'NONE',  ( -11.18376618407356737, 4.849999997815050534, -27.00000000000000355 ) ) ;
#6711=CARTESIAN_POINT ( 'NONE',  ( -15.10617644529808423, 100.0000000000000284, 15.98944417891004477 ) ) ;
#6712=VECTOR ( 'NONE', #10008, 1000.000000000000000 ) ;
#6713=ORIENTED_EDGE ( 'NONE', *, *, #3961, .F. ) ;
#6714=CARTESIAN_POINT ( 'NONE',  ( -16.36254897777738648, 99.50000000000000000, 15.39785597259249172 ) ) ;
#6715=EDGE_CURVE ( 'NONE', #6656, #4720, #3503, .T. ) ;
#6716=CARTESIAN_POINT ( 'NONE',  ( 5.825495487346713297, 100.0000000000000000, 20.69456627699299744 ) ) ;
#6717=DIRECTION ( 'NONE',  ( -0.1705044153832351028, 0.000000000000000000, 0.9853569121566161382 ) ) ;
#6718=CARTESIAN_POINT ( 'NONE',  ( 3.349514647153394975, 99.49999999999998579, -23.95461210612682024 ) ) ;
#6720=ORIENTED_EDGE ( 'NONE', *, *, #6350, .F. ) ;
#6721=CARTESIAN_POINT ( 'NONE',  ( 1.653273178848927064E-15, 1.599999997815050312, -27.00000000000000355 ) ) ;
#6722=CARTESIAN_POINT ( 'NONE',  ( 11.36312591709336139, 4.499999998907525445, -27.43301270000000258 ) ) ;
#6725=CARTESIAN_POINT ( 'NONE',  ( 3.635130212803377781, 99.99999999999997158, -23.00575896550913768 ) ) ;
#6726=CARTESIAN_POINT ( 'NONE',  ( 7.809833820264425519, 99.99999999999991473, 20.29999375863051370 ) ) ;
#6727=EDGE_LOOP ( 'NONE', ( #434, #5134 ) ) ;
#6728=CARTESIAN_POINT ( 'NONE',  ( 3.411785164761435674, 99.50000000000000000, -22.76693382491622231 ) ) ;
#6729=CARTESIAN_POINT ( 'NONE',  ( -4.959819536546781389E-15, 2.799999997815050268, 27.00000000000000355 ) ) ;
#6736=VERTEX_POINT ( 'NONE', #215 ) ;
#6738=EDGE_CURVE ( 'NONE', #3772, #4679, #8171, .T. ) ;
#6740=CARTESIAN_POINT ( 'NONE',  ( -14.79004890936967875, 99.49999999999998579, 16.19006955939758541 ) ) ;
#6742=CARTESIAN_POINT ( 'NONE',  ( 27.43301270000000258, 2.699999998907525178, -11.36312591709336139 ) ) ;
#6745=CARTESIAN_POINT ( 'NONE',  ( 3.411785164761435674, 99.50000000000000000, -22.76693382491622231 ) ) ;
#6746=DIRECTION ( 'NONE',  ( -0.000000000000000000, 1.000000000000000000, -0.000000000000000000 ) ) ;
#6749=LINE ( 'NONE', #4400, #8290 ) ;
#6751=CARTESIAN_POINT ( 'NONE',  ( -11.36312591709335962, 0.4999999989075251672, -27.43301270000000258 ) ) ;
#6754=EDGE_CURVE ( 'NONE', #3778, #5950, #5500, .T. ) ;
#6756=DIRECTION ( 'NONE',  ( -0.000000000000000000, 1.000000000000000000, -0.000000000000000000 ) ) ;
#6758=CARTESIAN_POINT ( 'NONE',  ( -16.30427144417478402, 99.99999999999998579, 16.48895498912494517 ) ) ;
#6761=CARTESIAN_POINT ( 'NONE',  ( 7.156925775808251622, 100.0000000000000000, 23.91622092442889524 ) ) ;
#6762=CARTESIAN_POINT ( 'NONE',  ( 27.43301270000000258, 0.2499999989075252504, 0.000000000000000000 ) ) ;
#6763=CIRCLE ( 'NONE', #8947, 27.00000000000000355 ) ;
#6764=DIRECTION ( 'NONE',  ( -0.000000000000000000, 1.000000000000000000, -0.000000000000000000 ) ) ;
#6765=CARTESIAN_POINT ( 'NONE',  ( -15.32348647777738826, 100.0000000000000000, 15.39505148541300450 ) ) ;
#6766=( BOUNDED_CURVE ( )  B_SPLINE_CURVE ( 2, ( #7060, #4605, #628, #2934, #7797 ),
 .UNSPECIFIED., .F., .F. ) 
 B_SPLINE_CURVE_WITH_KNOTS ( ( 3, 2, 3 ),
 ( 0.000000000000000000, 0.01785714285714285615, 0.03571428571428571230 ),
 .UNSPECIFIED. ) 
 CURVE ( )  GEOMETRIC_REPRESENTATION_ITEM ( )  RATIONAL_B_SPLINE_CURVE ( ( 1.000000000000000000, 0.9238795325112867385, 1.000000000000000000, 0.9238795325112867385, 1.000000000000000000 ) ) 
 REPRESENTATION_ITEM ( '' )  );
#6767=VERTEX_POINT ( 'NONE', #6593 ) ;
#6768=CARTESIAN_POINT ( 'NONE',  ( -11.18376618407358336, 2.949999999999999289, 26.99999999999999645 ) ) ;
#6771=CARTESIAN_POINT ( 'NONE',  ( 9.915951879163557692, 100.0000000000000284, 20.63215000232408158 ) ) ;
#6773=ADVANCED_FACE ( 'NONE', ( #2777 ), #9885, .T. ) ;
#6774=CARTESIAN_POINT ( 'NONE',  ( 21.79306891025641235, 100.0000000000000000, -1.065004006410256387 ) ) ;
#6775=CARTESIAN_POINT ( 'NONE',  ( -11.36312591709335962, 4.599999998907525978, -27.43301270000000258 ) ) ;
#6776=ADVANCED_FACE ( 'NONE', ( #9105 ), #6642, .T. ) ;
#6777=DIRECTION ( 'NONE',  ( -0.000000000000000000, 1.000000000000000000, -0.000000000000000000 ) ) ;
#6779=CARTESIAN_POINT ( 'NONE',  ( 5.825495487346713297, 99.50000000000000000, 20.69456627699299744 ) ) ;
#6780=CARTESIAN_POINT ( 'NONE',  ( -19.09188309203678813, 4.299999997815050712, 19.09188309203678457 ) ) ;
#6781=CARTESIAN_POINT ( 'NONE',  ( -22.57971655928959365, 99.50000000000000000, -10.84768434062017839 ) ) ;
#6782=FACE_BOUND ( 'NONE', #336, .T. ) ;
#6783=CARTESIAN_POINT ( 'NONE',  ( 0.000000000000000000, 85.00000000000000000, 0.000000000000000000 ) ) ;
#6785=CARTESIAN_POINT ( 'NONE',  ( 4.803433990161294354, 100.0000000000000142, -23.96838578116891583 ) ) ;
#6786=CARTESIAN_POINT ( 'NONE',  ( -19.39806930854667755, 2.249999998907525001, -19.39806930854668110 ) ) ;
#6791=DIRECTION ( 'NONE',  ( 0.000000000000000000, -0.000000000000000000, 1.000000000000000000 ) ) ;
#6793=CARTESIAN_POINT ( 'NONE',  ( 19.39806930854667399, 3.349999998907525534, 19.39806930854668465 ) ) ;
#6795=ORIENTED_EDGE ( 'NONE', *, *, #4869, .F. ) ;
#6796=CARTESIAN_POINT ( 'NONE',  ( 9.600410285814406919, 99.99999999999998579, 19.87914582625927196 ) ) ;
#6797=CARTESIAN_POINT ( 'NONE',  ( 4.386516977709190357, 100.0000000000000426, -24.31220192127581825 ) ) ;
#6799=CARTESIAN_POINT ( 'NONE',  ( 4.054941747578200584, 99.99999999999998579, -24.36678493958047298 ) ) ;
#6800=CARTESIAN_POINT ( 'NONE',  ( 5.725936192474917696, 99.50000000000000000, 21.08018326417248645 ) ) ;
#6801=CARTESIAN_POINT ( 'NONE',  ( -21.16695614262292580, 99.50000000000000000, -11.33496398805607441 ) ) ;
#6802=VERTEX_POINT ( 'NONE', #7581 ) ;
#6803=DIRECTION ( 'NONE',  ( 0.000000000000000000, 1.000000000000000000, 0.000000000000000000 ) ) ;
#6804=CARTESIAN_POINT ( 'NONE',  ( -27.43301270000000258, 1.449999998907525178, -3.359575119402369376E-15 ) ) ;
#6806=CARTESIAN_POINT ( 'NONE',  ( 4.128176300878408256, 100.0000000000000142, -21.47174600747824869 ) ) ;
#6807=CARTESIAN_POINT ( 'NONE',  ( 3.222930479149370253, 99.49999999999995737, -22.15251218086615381 ) ) ;
#6808=CARTESIAN_POINT ( 'NONE',  ( -15.07178375341841381, 99.50000000000000000, 16.66969090848992607 ) ) ;
#6809=EDGE_LOOP ( 'NONE', ( #7912, #2636, #8092, #1928 ) ) ;
#6813=VERTEX_POINT ( 'NONE', #1825 ) ;
#6814=ADVANCED_FACE ( 'NONE', ( #8270 ), #3454, .T. ) ;
#6816=DIRECTION ( 'NONE',  ( 0.000000000000000000, 0.000000000000000000, -1.000000000000000000 ) ) ;
#6817=CARTESIAN_POINT ( 'NONE',  ( -11.36312591709335962, 0.4999999989075252782, -27.43301270000000258 ) ) ;
#6818=CARTESIAN_POINT ( 'NONE',  ( -19.46743691185369585, 99.50000000000000000, -8.912588186774021537 ) ) ;
#6819=CARTESIAN_POINT ( 'NONE',  ( 4.401614252286283779, 99.50000000000002842, -24.65974366035752396 ) ) ;
#6820=DIRECTION ( 'NONE',  ( -0.000000000000000000, -1.000000000000000000, -0.000000000000000000 ) ) ;
#6821=CARTESIAN_POINT ( 'NONE',  ( -16.91659681606879317, 100.0000000000000000, 15.78485274883190392 ) ) ;
#6822=CARTESIAN_POINT ( 'NONE',  ( -4.959819536546781389E-15, 0.6000000000000000888, 27.00000000000000355 ) ) ;
#6823=ORIENTED_EDGE ( 'NONE', *, *, #9480, .T. ) ;
#6825=CARTESIAN_POINT ( 'NONE',  ( 1.679787559701184688E-15, 3.749999998907525445, -27.43301270000000258 ) ) ;
#6828=ORIENTED_EDGE ( 'NONE', *, *, #2801, .F. ) ;
#6831=DIRECTION ( 'NONE',  ( 0.000000000000000000, 1.000000000000000000, 0.000000000000000000 ) ) ;
#6835=CARTESIAN_POINT ( 'NONE',  ( 3.504547665631520648, 99.99999999999997158, -23.10026541809159184 ) ) ;
#6836=EDGE_CURVE ( 'NONE', #7711, #2107, #7235, .T. ) ;
#6837=ORIENTED_EDGE ( 'NONE', *, *, #7813, .T. ) ;
#6838=CARTESIAN_POINT ( 'NONE',  ( -16.61132721736409934, 100.0000000000000142, 16.61681399495993716 ) ) ;
#6839=CARTESIAN_POINT ( 'NONE',  ( 19.39806930854668110, 2.049999998907525711, -19.39806930854668110 ) ) ;
#6840=ORIENTED_EDGE ( 'NONE', *, *, #1716, .F. ) ;
#6845=DIRECTION ( 'NONE',  ( -0.000000000000000000, -1.000000000000000000, -0.000000000000000000 ) ) ;
#6846=CARTESIAN_POINT ( 'NONE',  ( 11.36312591709336139, 2.099999998907525089, -27.43301270000000258 ) ) ;
#6848=CARTESIAN_POINT ( 'NONE',  ( -16.38049141020750099, 100.0000000000000426, 14.97568473612765416 ) ) ;
#6850=DIRECTION ( 'NONE',  ( 0.000000000000000000, 0.000000000000000000, 1.000000000000000000 ) ) ;
#6851=CARTESIAN_POINT ( 'NONE',  ( -15.91768310440539658, 100.0000000000000284, 15.18344740530786652 ) ) ;
#6852=AXIS2_PLACEMENT_3D ( 'NONE', #8990, #6627, #4327 ) ;
#6855=ORIENTED_EDGE ( 'NONE', *, *, #7681, .F. ) ;
#6856=CARTESIAN_POINT ( 'NONE',  ( 0.000000000000000000, 97.50000000000000000, 0.000000000000000000 ) ) ;
#6857=CARTESIAN_POINT ( 'NONE',  ( -27.43301270000000969, 1.499999998907525223, 11.36312591709335429 ) ) ;
#6860=CARTESIAN_POINT ( 'NONE',  ( -15.29853103387017121, 99.99999999999997158, 14.98378122532347057 ) ) ;
#6861=CARTESIAN_POINT ( 'NONE',  ( 9.554054106072296548, 99.99999999999994316, 20.45778517829714360 ) ) ;
#6862=CYLINDRICAL_SURFACE ( 'NONE', #4119, 27.00000000000000355 ) ;
#6863=VERTEX_POINT ( 'NONE', #7525 ) ;
#6864=ORIENTED_EDGE ( 'NONE', *, *, #3903, .T. ) ;
#6865=CARTESIAN_POINT ( 'NONE',  ( -16.11976138926855739, 99.49999999999997158, 16.60078749809536447 ) ) ;
#6866=B_SPLINE_CURVE_WITH_KNOTS ( 'NONE', 3,
 ( #432, #3573, #7594, #5922, #9217, #4514, #7709, #8440, #544, #9170, #2898 ),
 .UNSPECIFIED., .F., .F.,
 ( 4, 1, 1, 1, 1, 1, 1, 1, 4 ),
 ( 0.000000000000000000, 0.1514666391271576040, 0.2940212016997327260, 0.4289076436562640482, 0.5568069201790899481, 0.6759213874835566793, 0.7888117551744765477, 0.8972989960681465593, 1.000000000000000000 ),
 .UNSPECIFIED. ) ;
#6868=ORIENTED_EDGE ( 'NONE', *, *, #2074, .T. ) ;
#6869=CARTESIAN_POINT ( 'NONE',  ( -22.31427554260534052, 99.50000000000002842, -10.13077409178744404 ) ) ;
#6870=CARTESIAN_POINT ( 'NONE',  ( -15.58193289918752278, 100.0000000000000000, 16.98546238400348329 ) ) ;
#6871=CARTESIAN_POINT ( 'NONE',  ( 3.306546357697854128E-15, 100.0000000000000000, 27.00000000000000355 ) ) ;
#6873=CARTESIAN_POINT ( 'NONE',  ( 3.044406660298407452, 100.0000000000000000, -23.15442635585071685 ) ) ;
#6874=EDGE_CURVE ( 'NONE', #3644, #6902, #367, .T. ) ;
#6877=LINE ( 'NONE', #7663, #5821 ) ;
#6881=CARTESIAN_POINT ( 'NONE',  ( 11.36312591709336850, 4.199999998907525622, 27.43301269999999903 ) ) ;
#6883=CARTESIAN_POINT ( 'NONE',  ( 9.915951879163557692, 100.0000000000000142, 20.63215000232408158 ) ) ;
#6884=ADVANCED_FACE ( 'NONE', ( #3774 ), #5226, .F. ) ;
#6885=ORIENTED_EDGE ( 'NONE', *, *, #4220, .F. ) ;
#6886=CARTESIAN_POINT ( 'NONE',  ( -21.03505001771060634, 100.0000000000000000, -9.476849197711761263 ) ) ;
#6887=CARTESIAN_POINT ( 'NONE',  ( 4.599186066243659887, 99.50000000000002842, -24.59301055568561623 ) ) ;
#6888=DIRECTION ( 'NONE',  ( -0.000000000000000000, 1.000000000000000000, -0.000000000000000000 ) ) ;
#6889=CARTESIAN_POINT ( 'NONE',  ( -4.959819536546781389E-15, 5.199999997815050179, 27.00000000000000355 ) ) ;
#6890=ORIENTED_EDGE ( 'NONE', *, *, #6701, .F. ) ;
#6891=CARTESIAN_POINT ( 'NONE',  ( -15.43596444985078975, 100.0000000000000284, 15.30036492734783593 ) ) ;
#6892=CARTESIAN_POINT ( 'NONE',  ( 27.43301270000000258, 1.999999998907525001, -11.36312591709336139 ) ) ;
#6897=CARTESIAN_POINT ( 'NONE',  ( 2.955068081869620666, 99.99999999999995737, -21.57801138750623338 ) ) ;
#6899=CARTESIAN_POINT ( 'NONE',  ( -27.43301270000000258, 4.649999998907525800, -3.359575119402369376E-15 ) ) ;
#6900=CARTESIAN_POINT ( 'NONE',  ( 11.36312591709336139, 1.299999998907525267, -27.43301270000000258 ) ) ;
#6901=AXIS2_PLACEMENT_3D ( 'NONE', #2122, #8400, #1955 ) ;
#6902=VERTEX_POINT ( 'NONE', #2088 ) ;
#6903=EDGE_LOOP ( 'NONE', ( #2255, #2470, #6561, #2151 ) ) ;
#6905=CARTESIAN_POINT ( 'NONE',  ( 4.232798786556307036, 100.0000000000000000, -24.34936571594186105 ) ) ;
#6906=CARTESIAN_POINT ( 'NONE',  ( -16.49816537377288128, 99.50000000000000000, 16.70951083495554101 ) ) ;
#6910=CARTESIAN_POINT ( 'NONE',  ( 2.964854786877021642, 100.0000000000000000, -22.43901021186594846 ) ) ;
#6913=CARTESIAN_POINT ( 'NONE',  ( 1.679787559701184688E-15, 3.649999998907525356, -27.43301270000000258 ) ) ;
#6916=CARTESIAN_POINT ( 'NONE',  ( 0.000000000000000000, 100.0000000000000000, -27.00000000000000355 ) ) ;
#6917=CARTESIAN_POINT ( 'NONE',  ( 8.564701892180647036, 100.0000000000000284, 19.97971282122689018 ) ) ;
#6918=EDGE_LOOP ( 'NONE', ( #5492, #5009, #8294, #6644 ) ) ;
#6919=ORIENTED_EDGE ( 'NONE', *, *, #9527, .T. ) ;
#6924=CARTESIAN_POINT ( 'NONE',  ( 1.679787559701184688E-15, 0.4499999989075252338, -27.43301270000000258 ) ) ;
#6925=CARTESIAN_POINT ( 'NONE',  ( -21.87421819196487505, 99.50000000000000000, -9.684578881761979119 ) ) ;
#6926=B_SPLINE_SURFACE_WITH_KNOTS ( 'NONE', 3, 1, ( 
 ( #4407, #7590 ),
 ( #9953, #9896 ),
 ( #9116, #4300 ),
 ( #375, #1883 ),
 ( #4457, #8226 ),
 ( #1935, #1267 ),
 ( #6654, #1161 ),
 ( #1987, #5077 ),
 ( #3678, #5185 ),
 ( #3466, #7647 ),
 ( #1833, #9067 ),
 ( #5029, #484 ),
 ( #7486, #6861 ),
 ( #10058, #5132 ),
 ( #1059, #8384 ) ),
 .UNSPECIFIED., .F., .F., .F.,
 ( 4, 1, 1, 1, 1, 1, 1, 1, 1, 1, 1, 1, 4 ),
 ( 2, 2 ),
 ( 0.000000000000000000, 0.1101401978779246588, 0.2116695470404897084, 0.3047824012491699430, 0.3893374185178356539, 0.4648567744508144695, 0.5325800579573772842, 0.5913915682020929321, 0.6424829260185016544, 0.7344861914544180692, 0.8232371011010507500, 0.9113455750355911045, 1.000000000000000000 ),
 ( 0.000000000000000000, 1.000000000000000000 ),
 .UNSPECIFIED. ) ;
#6929=LINE ( 'NONE', #6986, #3221 ) ;
#6930=CARTESIAN_POINT ( 'NONE',  ( 19.09188309203678813, 4.699999997815051067, -19.09188309203678813 ) ) ;
#6931=B_SPLINE_CURVE_WITH_KNOTS ( 'NONE', 3,
 ( #665, #1554, #3859, #5540, #10252, #8731, #3083, #6267, #9464, #2292, #2546, #6421, #1658, #4991, #3370, #8042, #4849, #4210, #8880 ),
 .UNSPECIFIED., .F., .F.,
 ( 4, 1, 1, 1, 1, 1, 1, 1, 1, 1, 1, 1, 1, 1, 1, 1, 4 ),
 ( 0.000000000000000000, 0.07024023345195122559, 0.1375772235014411093, 0.2026681864156774648, 0.2655894380381068620, 0.3279415367477454546, 0.3896445486312665740, 0.4521557380645868096, 0.5154465764363311830, 0.5785479733725392704, 0.6397241484143471046, 0.6996998702489094502, 0.7590513234224176564, 0.8180896689983322423, 0.8773873076253557723, 0.9378402036119877216, 1.000000000000000000 ),
 .UNSPECIFIED. ) ;
#6935=CARTESIAN_POINT ( 'NONE',  ( 9.554054106072296548, 100.0000000000000142, 20.45778517829714360 ) ) ;
#6941=EDGE_LOOP ( 'NONE', ( #7678, #9241, #4151, #5011 ) ) ;
#6942=FACE_OUTER_BOUND ( 'NONE', #198, .T. ) ;
#6945=VECTOR ( 'NONE', #3804, 1000.000000000000114 ) ;
#6946=CARTESIAN_POINT ( 'NONE',  ( 0.000000000000000000, 87.00000000000001421, 0.000000000000000000 ) ) ;
#6947=ORIENTED_EDGE ( 'NONE', *, *, #7743, .F. ) ;
#6949=LINE ( 'NONE', #7791, #4289 ) ;
#6950=EDGE_LOOP ( 'NONE', ( #2234, #3067, #3847, #9197 ) ) ;
#6951=EDGE_CURVE ( 'NONE', #1438, #3772, #7751, .T. ) ;
#6954=DIRECTION ( 'NONE',  ( -0.000000000000000000, 1.000000000000000000, -0.000000000000000000 ) ) ;
#6956=CARTESIAN_POINT ( 'NONE',  ( -20.95611194834973645, 99.50000000000000000, -10.07788454426966318 ) ) ;
#6957=CARTESIAN_POINT ( 'NONE',  ( -27.43301270000000969, 2.399999998907525356, 11.36312591709335429 ) ) ;
#6960=CARTESIAN_POINT ( 'NONE',  ( -15.31787750341841559, 100.0000000000000000, 16.43551622900274722 ) ) ;
#6963=CARTESIAN_POINT ( 'NONE',  ( 3.888553205800344248, 99.99999999999995737, -24.35333287445124739 ) ) ;
#6964=VECTOR ( 'NONE', #2097, 1000.000000000000000 ) ;
#6967=CARTESIAN_POINT ( 'NONE',  ( 3.681717055787076642, 100.0000000000000000, -21.09125273517263111 ) ) ;
#6968=ORIENTED_EDGE ( 'NONE', *, *, #1731, .F. ) ;
#6970=CARTESIAN_POINT ( 'NONE',  ( 11.36312591709336850, 2.499999998907525445, 27.43301269999999903 ) ) ;
#6973=CARTESIAN_POINT ( 'NONE',  ( 27.00000000000000355, 1.649999999999999911, -11.18376618407356737 ) ) ;
#6975=DIRECTION ( 'NONE',  ( 0.000000000000000000, 0.000000000000000000, -1.000000000000000000 ) ) ;
#6976=ORIENTED_EDGE ( 'NONE', *, *, #368, .T. ) ;
#6977=CARTESIAN_POINT ( 'NONE',  ( -16.57687742313193269, 99.99999999999998579, 15.91855687263828756 ) ) ;
#6978=CARTESIAN_POINT ( 'NONE',  ( 8.122452352567329115, 100.0000000000000000, 21.04970292111833530 ) ) ;
#6982=ORIENTED_EDGE ( 'NONE', *, *, #4672, .T. ) ;
#6983=EDGE_CURVE ( 'NONE', #10090, #5876, #9374, .T. ) ;
#6986=CARTESIAN_POINT ( 'NONE',  ( 1.653273178848927064E-15, 5.324999998907524734, -27.00000000000000355 ) ) ;
#6988=AXIS2_PLACEMENT_3D ( 'NONE', #6628, #8943, #1135 ) ;
#6989=CARTESIAN_POINT ( 'NONE',  ( 24.93339342948717885, 99.50000000000000000, -1.235376602564102644 ) ) ;
#6990=CARTESIAN_POINT ( 'NONE',  ( 3.207968951880266761, 99.49999999999998579, -22.92616835434091627 ) ) ;
#6991=CARTESIAN_POINT ( 'NONE',  ( 19.09188309203678102, 0.6999999999999999556, 19.09188309203678813 ) ) ;
#6993=VERTEX_POINT ( 'NONE', #3670 ) ;
#6994=CARTESIAN_POINT ( 'NONE',  ( 9.676361905416721143, 99.50000000000001421, 21.63547735782115566 ) ) ;
#6998=CARTESIAN_POINT ( 'NONE',  ( 9.357053078540884528, 100.0000000000000142, 19.70216357796830664 ) ) ;
#7001=CARTESIAN_POINT ( 'NONE',  ( -16.61132721736409934, 99.50000000000001421, 16.61681399495993716 ) ) ;
#7002=CARTESIAN_POINT ( 'NONE',  ( 27.43301269999999548, 1.099999998907525312, 11.36312591709337916 ) ) ;
#7006=PLANE ( 'NONE',  #3416 ) ;
#7009=CARTESIAN_POINT ( 'NONE',  ( -27.43301270000000969, 4.699999998907524734, 11.36312591709335429 ) ) ;
#7010=CARTESIAN_POINT ( 'NONE',  ( -27.43301270000000258, 1.549999998907525267, -3.359575119402369376E-15 ) ) ;
#7012=EDGE_CURVE ( 'NONE', #2877, #6069, #6176, .T. ) ;
#7013=CARTESIAN_POINT ( 'NONE',  ( 9.778118981323553172, 99.99999999999998579, 20.11889122584574352 ) ) ;
#7014=CARTESIAN_POINT ( 'NONE',  ( 5.243816414761435674, 99.50000000000000000, -23.48558366465980995 ) ) ;
#7015=PLANE ( 'NONE',  #1940 ) ;
#7017=CARTESIAN_POINT ( 'NONE',  ( -21.03505001771060634, 99.50000000000000000, -9.476849197711761263 ) ) ;
#7018=EDGE_LOOP ( 'NONE', ( #1080, #9710, #10173, #1200, #5425, #4145, #8973, #7862, #9417, #4357, #6167, #5205 ) ) ;
#7021=CARTESIAN_POINT ( 'NONE',  ( 11.36312591709336850, 1.699999998907525178, 27.43301269999999903 ) ) ;
#7023=VERTEX_POINT ( 'NONE', #4554 ) ;
#7024=CARTESIAN_POINT ( 'NONE',  ( -15.10737684033046335, 99.99999999999995737, 15.12848924955281049 ) ) ;
#7025=CARTESIAN_POINT ( 'NONE',  ( 1.653273178848927064E-15, 2.600000000000000533, -27.00000000000000355 ) ) ;
#7026=CARTESIAN_POINT ( 'NONE',  ( 9.044794778432494908, 99.50000000000001421, 19.94873160813952140 ) ) ;
#7029=CARTESIAN_POINT ( 'NONE',  ( -16.41302370085497131, 99.49999999999998579, 15.45185748370271206 ) ) ;
#7030=CARTESIAN_POINT ( 'NONE',  ( 8.231219904624582639, 99.50000000000000000, 20.21381436664452735 ) ) ;
#7035=CARTESIAN_POINT ( 'NONE',  ( -27.43301270000000258, 1.449999998907525178, -3.359575119402369376E-15 ) ) ;
#7039=CARTESIAN_POINT ( 'NONE',  ( 5.207032889226773875, 99.50000000000000000, -23.83708953234284778 ) ) ;
#7040=ADVANCED_FACE ( 'NONE', ( #3723 ), #7100, .T. ) ;
#7043=CARTESIAN_POINT ( 'NONE',  ( 4.200543313440712190, 100.0000000000000000, -21.13206004899810608 ) ) ;
#7044=LINE ( 'NONE', #5377, #7614 ) ;
#7048=ADVANCED_FACE ( 'NONE', ( #740 ), #5606, .T. ) ;
#7050=CARTESIAN_POINT ( 'NONE',  ( 1.653273178848927064E-15, 5.599999997815050534, -27.00000000000000355 ) ) ;
#7051=( BOUNDED_CURVE ( )  B_SPLINE_CURVE ( 2, ( #3593, #7877, #8352, #1183, #8673, #3959, #6930, #7560, #4692 ),
 .UNSPECIFIED., .F., .F. ) 
 B_SPLINE_CURVE_WITH_KNOTS ( ( 3, 2, 2, 2, 3 ),
 ( 0.6785714285714286031, 0.6964285714285713969, 0.7142857142857143016, 0.7321428571428570953, 0.7500000000000000000 ),
 .UNSPECIFIED. ) 
 CURVE ( )  GEOMETRIC_REPRESENTATION_ITEM ( )  RATIONAL_B_SPLINE_CURVE ( ( 1.000000000000000000, 0.9238795325112867385, 1.000000000000000000, 0.9238795325112867385, 1.000000000000000000, 0.9238795325112867385, 1.000000000000000000, 0.9238795325112867385, 1.000000000000000000 ) ) 
 REPRESENTATION_ITEM ( '' )  );
#7053=EDGE_LOOP ( 'NONE', ( #2295, #7491, #6982, #6573 ) ) ;
#7054=CARTESIAN_POINT ( 'NONE',  ( -15.56095293356939813, 99.50000000000001421, 15.23332223661997453 ) ) ;
#7055=CARTESIAN_POINT ( 'NONE',  ( -27.43301270000000258, 3.149999998907524912, -3.359575119402369376E-15 ) ) ;
#7058=CARTESIAN_POINT ( 'NONE',  ( -20.95611194834973645, 100.0000000000000000, -10.07788454426966318 ) ) ;
#7060=CARTESIAN_POINT ( 'NONE',  ( 27.00000000000000355, 0.5999999978150503122, 0.000000000000000000 ) ) ;
#7061=CARTESIAN_POINT ( 'NONE',  ( 19.39806930854668110, 3.649999998907525356, -19.39806930854668110 ) ) ;
#7063=CIRCLE ( 'NONE', #7548, 25.00000000000000000 ) ;
#7064=CARTESIAN_POINT ( 'NONE',  ( -15.27171031718473770, 99.50000000000002842, 15.44886715306589764 ) ) ;
#7065=B_SPLINE_CURVE_WITH_KNOTS ( 'NONE', 3,
 ( #10164, #7856, #3001, #7120, #6177, #7693, #7067, #6120, #5556, #6288, #9375, #9487, #5405, #8537, #5511 ),
 .UNSPECIFIED., .F., .F.,
 ( 4, 1, 1, 1, 1, 1, 1, 1, 1, 1, 1, 1, 4 ),
 ( 0.000000000000000000, 0.08963690308348271074, 0.1775767702671464110, 0.2649576542713044658, 0.3533131777157214604, 0.4402865524342069459, 0.5245518675747646853, 0.6066224975438009315, 0.6889424263984335051, 0.7698335385027974542, 0.8475882324521423206, 0.9236428641877653112, 1.000000000000000000 ),
 .UNSPECIFIED. ) ;
#7066=CARTESIAN_POINT ( 'NONE',  ( 3.664124300404482337, 99.50000000000002842, -24.27219056640880623 ) ) ;
#7067=CARTESIAN_POINT ( 'NONE',  ( 3.106448761625311139, 99.49999999999998579, -21.38062202216113761 ) ) ;
#7068=DIRECTION ( 'NONE',  ( 0.05409991075415103434, 0.000000000000000000, 0.9985355274883277454 ) ) ;
#7070=CARTESIAN_POINT ( 'NONE',  ( -21.69499712064247277, 99.49999999999998579, -9.295461156691713356 ) ) ;
#7073=CARTESIAN_POINT ( 'NONE',  ( -5.039362679103552881E-15, 0.9499999989075252893, 27.43301270000000258 ) ) ;
#7076=CARTESIAN_POINT ( 'NONE',  ( -15.07178375341841559, 99.99999999999997158, 15.16157792772069968 ) ) ;
#7078=CARTESIAN_POINT ( 'NONE',  ( 19.09188309203678813, 2.500000000000000000, -19.09188309203678813 ) ) ;
#7079=CARTESIAN_POINT ( 'NONE',  ( 9.513000527211589841, 99.50000000000000000, 20.35102222961602436 ) ) ;
#7081=CARTESIAN_POINT ( 'NONE',  ( -16.54770463920453949, 99.50000000000002842, 15.70234036036222847 ) ) ;
#7082=CARTESIAN_POINT ( 'NONE',  ( 8.067960508813904141, 100.0000000000000000, 20.80952186068213905 ) ) ;
#7086=CARTESIAN_POINT ( 'NONE',  ( -11.36312591709337561, 2.399999998907525356, 27.43301269999999548 ) ) ;
#7090=CARTESIAN_POINT ( 'NONE',  ( -16.37951318544778445, 99.99999999999997158, 15.41600550949200077 ) ) ;
#7092=CARTESIAN_POINT ( 'NONE',  ( 4.486604876299897349, 99.99999999999997158, -21.85617661337775885 ) ) ;
#7097=CARTESIAN_POINT ( 'NONE',  ( -15.72775836928289017, 100.0000000000000000, 17.03252426573849476 ) ) ;
#7100=B_SPLINE_SURFACE_WITH_KNOTS ( 'NONE', 3, 1, ( 
 ( #474, #6905 ),
 ( #632, #9432 ),
 ( #3830, #10102 ),
 ( #7634, #2258 ),
 ( #4666, #2938 ),
 ( #8648, #2831 ),
 ( #3878, #9204 ),
 ( #3933, #5510 ),
 ( #7066, #10320 ),
 ( #4817, #3203 ),
 ( #9679, #9534 ),
 ( #1624, #3157 ),
 ( #5709, #9486 ),
 ( #7172, #2518 ),
 ( #7907, #9579 ),
 ( #7217, #6340 ),
 ( #4915, #6438 ),
 ( #6488, #4714 ),
 ( #9630, #7119 ) ),
 .UNSPECIFIED., .F., .F., .F.,
 ( 4, 1, 1, 1, 1, 1, 1, 1, 1, 1, 1, 1, 1, 1, 1, 1, 4 ),
 ( 2, 2 ),
 ( 0.000000000000000000, 0.07313710028058939550, 0.1429478298248799129, 0.2105045057187734658, 0.2751999312753631854, 0.3390602298032547868, 0.4018764873508149926, 0.4650016082884899093, 0.5281538368899733049, 0.5906348070863262079, 0.6510495490485337378, 0.7103018853965116230, 0.7674338915725752441, 0.8249350906448947862, 0.8823686014076175255, 0.9405824579944982444, 1.000000000000000000 ),
 ( 0.000000000000000000, 1.000000000000000000 ),
 .UNSPECIFIED. ) ;
#7101=ORIENTED_EDGE ( 'NONE', *, *, #3786, .T. ) ;
#7103=VECTOR ( 'NONE', #6698, 1000.000000000000000 ) ;
#7107=CARTESIAN_POINT ( 'NONE',  ( -16.30857500771091040, 99.99999999999994316, 15.34700649443169063 ) ) ;
#7109=CARTESIAN_POINT ( 'NONE',  ( 1.679787559701184688E-15, 4.549999998907526155, -27.43301270000000258 ) ) ;
#7110=EDGE_LOOP ( 'NONE', ( #8997, #2447, #1563, #8455 ) ) ;
#7111=EDGE_CURVE ( 'NONE', #7619, #3366, #8684, .T. ) ;
#7114=CARTESIAN_POINT ( 'NONE',  ( 3.374624233514611937, 99.50000000000002842, -23.25900349070959550 ) ) ;
#7116=CARTESIAN_POINT ( 'NONE',  ( -20.97746206809550884, 100.0000000000000000, -11.22189255051946688 ) ) ;
#7117=CARTESIAN_POINT ( 'NONE',  ( -27.43301270000000969, 4.799999998907525267, 11.36312591709335429 ) ) ;
#7118=DIRECTION ( 'NONE',  ( 0.9853569121566161382, 0.000000000000000000, 0.1705044153832351028 ) ) ;
#7119=CARTESIAN_POINT ( 'NONE',  ( 3.282077632710153292, 100.0000000000000000, -23.74569985055724786 ) ) ;
#7120=CARTESIAN_POINT ( 'NONE',  ( 3.428579745388047328, 99.49999999999998579, -21.16399209792802694 ) ) ;
#7123=CARTESIAN_POINT ( 'NONE',  ( -21.59614764830937972, 99.50000000000001421, -9.292069227195950631 ) ) ;
#7124=ORIENTED_EDGE ( 'NONE', *, *, #9346, .F. ) ;
#7126=CARTESIAN_POINT ( 'NONE',  ( 27.43301270000000258, 0.3499999989075252005, 0.000000000000000000 ) ) ;
#7128=CARTESIAN_POINT ( 'NONE',  ( -19.09188309203678813, 1.300000000000000266, 19.09188309203678457 ) ) ;
#7130=ORIENTED_EDGE ( 'NONE', *, *, #3912, .T. ) ;
#7131=AXIS2_PLACEMENT_3D ( 'NONE', #7665, #10135, #10074 ) ;
#7133=CARTESIAN_POINT ( 'NONE',  ( -20.96643530928959365, 99.99999999999997158, -10.05541671241504886 ) ) ;
#7136=DIRECTION ( 'NONE',  ( -0.3923910917372159246, 0.000000000000000000, -0.9197984731044490658 ) ) ;
#7137=CARTESIAN_POINT ( 'NONE',  ( -27.43301270000000258, 2.249999998907525001, -3.359575119402369376E-15 ) ) ;
#7138=CARTESIAN_POINT ( 'NONE',  ( 3.472565890032746960, 99.50000000000002842, -24.54662015932514052 ) ) ;
#7139=CARTESIAN_POINT ( 'NONE',  ( -22.55793349878803156, 99.50000000000000000, -10.88926985104519929 ) ) ;
#7140=VECTOR ( 'NONE', #3707, 1000.000000000000000 ) ;
#7142=CARTESIAN_POINT ( 'NONE',  ( -16.54512803120131181, 100.0000000000000000, 16.13427955854364626 ) ) ;
#7143=CARTESIAN_POINT ( 'NONE',  ( 9.873655262861264603, 99.99999999999998579, 20.34710108723753308 ) ) ;
#7144=CARTESIAN_POINT ( 'NONE',  ( 4.405197143102897783, 99.99999999999994316, -21.72932741277565682 ) ) ;
#7145=EDGE_CURVE ( 'NONE', #463, #4730, #3105, .T. ) ;
#7149=CARTESIAN_POINT ( 'NONE',  ( 4.723706824522782455, 100.0000000000000142, -24.08630974238606370 ) ) ;
#7158=CARTESIAN_POINT ( 'NONE',  ( -22.21584973381871464, 99.50000000000001421, -9.938501092090024969 ) ) ;
#7159=CARTESIAN_POINT ( 'NONE',  ( 9.446088657802272692, 100.0000000000000426, 20.22669104216016578 ) ) ;
#7160=VERTEX_POINT ( 'NONE', #6386 ) ;
#7162=EDGE_CURVE ( 'NONE', #8581, #1470, #976, .T. ) ;
#7166=ADVANCED_FACE ( 'NONE', ( #3250 ), #9355, .T. ) ;
#7167=CARTESIAN_POINT ( 'NONE',  ( -21.30928386698190025, 99.50000000000000000, -11.02857376369709996 ) ) ;
#7168=CARTESIAN_POINT ( 'NONE',  ( -27.00000000000001421, 1.049999997815050490, 11.18376618407356382 ) ) ;
#7169=UNCERTAINTY_MEASURE_WITH_UNIT (LENGTH_MEASURE( 1.000000000000000082E-05 ), #1688, 'distance_accuracy_value', 'NONE');
#7170=CARTESIAN_POINT ( 'NONE',  ( -15.13293277027690209, 99.99999999999997158, 16.13104881108577970 ) ) ;
#7172=CARTESIAN_POINT ( 'NONE',  ( 3.386276725104728769, 99.50000000000001421, -24.01678749451497907 ) ) ;
#7173=CARTESIAN_POINT ( 'NONE',  ( -16.05266356869597644, 99.50000000000000000, 16.62382211633880047 ) ) ;
#7176=CARTESIAN_POINT ( 'NONE',  ( -20.95972469638759250, 99.50000000000000000, -9.536167108072199028 ) ) ;
#7177=VERTEX_POINT ( 'NONE', #4136 ) ;
#7179=CARTESIAN_POINT ( 'NONE',  ( 11.36312591709336850, 4.899999998907526688, 27.43301269999999903 ) ) ;
#7180=DIRECTION ( 'NONE',  ( -0.000000000000000000, 1.000000000000000000, -0.000000000000000000 ) ) ;
#7181=CARTESIAN_POINT ( 'NONE',  ( 1.653273178848927064E-15, 3.400000000000000355, -27.00000000000000355 ) ) ;
#7182=CARTESIAN_POINT ( 'NONE',  ( 3.298672054714395063, 100.0000000000000142, -22.72039518595936869 ) ) ;
#7183=ADVANCED_FACE ( 'NONE', ( #6676 ), #7462, .F. ) ;
#7184=( NAMED_UNIT ( * ) SI_UNIT ( $, .STERADIAN. ) SOLID_ANGLE_UNIT ( ) );
#7188=CARTESIAN_POINT ( 'NONE',  ( 27.00000000000000355, 0.05000000000000000278, -11.18376618407356915 ) ) ;
#7189=CARTESIAN_POINT ( 'NONE',  ( -11.36312591709337561, 1.599999998907525756, 27.43301269999999548 ) ) ;
#7190=CARTESIAN_POINT ( 'NONE',  ( 4.241330131419338123, 99.99999999999998579, -24.68798891778770965 ) ) ;
#7192=CARTESIAN_POINT ( 'NONE',  ( -27.00000000000001421, 1.049999997815050490, 11.18376618407356560 ) ) ;
#7194=DIRECTION ( 'NONE',  ( -0.9197984731044490658, 0.000000000000000000, 0.3923910917372159246 ) ) ;
#7195=CARTESIAN_POINT ( 'NONE',  ( -22.33111803333905243, 99.99999999999997158, -9.558150950182401573 ) ) ;
#7196=CARTESIAN_POINT ( 'NONE',  ( 1.653273178848927064E-15, 5.599999997815050534, -27.00000000000000355 ) ) ;
#7198=VECTOR ( 'NONE', #8784, 1000.000000000000000 ) ;
#7199=CARTESIAN_POINT ( 'NONE',  ( 1.653273178848927064E-15, 4.200000000000000178, -27.00000000000000355 ) ) ;
#7200=CARTESIAN_POINT ( 'NONE',  ( -15.45548338988150938, 99.99999999999997158, 16.93306818456458984 ) ) ;
#7201=DIRECTION ( 'NONE',  ( -0.5137073458062109133, 0.000000000000000000, -0.8579654788304353907 ) ) ;
#7204=DIRECTION ( 'NONE',  ( 0.000000000000000000, 1.000000000000000000, 0.000000000000000000 ) ) ;
#7206=CARTESIAN_POINT ( 'NONE',  ( 26.99999999999999645, 2.949999997815051067, 11.18376618407358691 ) ) ;
#7207=CARTESIAN_POINT ( 'NONE',  ( 27.43301269999999548, 5.099999998907525089, 11.36312591709337916 ) ) ;
#7211=CARTESIAN_POINT ( 'NONE',  ( 2.852289972453743161, 99.99999999999997158, -22.14293542748032451 ) ) ;
#7213=CARTESIAN_POINT ( 'NONE',  ( -20.79740905086423552, 100.0000000000000142, -11.06234285579171051 ) ) ;
#7214=CARTESIAN_POINT ( 'NONE',  ( 19.09188309203678813, 1.499999997815050223, -19.09188309203678813 ) ) ;
#7215=CARTESIAN_POINT ( 'NONE',  ( -15.11611088805441661, 99.99999999999997158, 16.06180012866831319 ) ) ;
#7216=VECTOR ( 'NONE', #5249, 1000.000000000000114 ) ;
#7217=CARTESIAN_POINT ( 'NONE',  ( 3.320270046935387853, 99.49999999999998579, -23.88810568987970484 ) ) ;
#7218=CARTESIAN_POINT ( 'NONE',  ( 3.611424427577684781, 100.0000000000000142, -21.45475674085064099 ) ) ;
#7222=CARTESIAN_POINT ( 'NONE',  ( 3.286905236079108672, 99.50000000000004263, -23.77014634954566574 ) ) ;
#7223=ORIENTED_EDGE ( 'NONE', *, *, #8265, .F. ) ;
#7224=ORIENTED_EDGE ( 'NONE', *, *, #8122, .F. ) ;
#7226=CARTESIAN_POINT ( 'NONE',  ( 27.43301269999999548, 1.099999998907525089, 11.36312591709337738 ) ) ;
#7229=CARTESIAN_POINT ( 'NONE',  ( 27.43301270000000258, 1.049999998907525267, 0.000000000000000000 ) ) ;
#7232=LINE ( 'NONE', #860, #8739 ) ;
#7233=CARTESIAN_POINT ( 'NONE',  ( 4.739008722453744049, 99.50000000000001421, -24.06821587619827696 ) ) ;
#7235=B_SPLINE_CURVE_WITH_KNOTS ( 'NONE', 3,
 ( #1050, #7423, #5123, #5861, #1098, #3615, #4293, #6797, #1926, #4341, #8957 ),
 .UNSPECIFIED., .F., .F.,
 ( 4, 1, 1, 1, 1, 1, 1, 1, 4 ),
 ( 0.000000000000000000, 0.1199228846740813259, 0.2396820999030742083, 0.3587608595380448184, 0.4799620281296770319, 0.6043577515038436321, 0.7314057062717854718, 0.8632643124108332344, 1.000000000000000000 ),
 .UNSPECIFIED. ) ;
#7236=CARTESIAN_POINT ( 'NONE',  ( -5.039362679103552881E-15, 1.649999998907525356, 27.43301270000000258 ) ) ;
#7238=CARTESIAN_POINT ( 'NONE',  ( -27.00000000000000355, 1.950000000000000400, -11.18376618407357270 ) ) ;
#7240=CARTESIAN_POINT ( 'NONE',  ( -22.22752541189434794, 99.99999999999994316, -11.26717589342885084 ) ) ;
#7243=CARTESIAN_POINT ( 'NONE',  ( -22.21668755910108928, 100.0000000000000426, -9.472979539922778969 ) ) ;
#7244=CARTESIAN_POINT ( 'NONE',  ( 27.00000000000000355, 5.449999997815051067, -11.18376618407356915 ) ) ;
#7247=ORIENTED_EDGE ( 'NONE', *, *, #5805, .F. ) ;
#7248=DIRECTION ( 'NONE',  ( -0.000000000000000000, -1.000000000000000000, -0.000000000000000000 ) ) ;
#7249=LINE ( 'NONE', #2339, #3132 ) ;
#7250=CARTESIAN_POINT ( 'NONE',  ( -21.86704275050744073, 99.50000000000001421, -11.06111336656620026 ) ) ;
#7252=CARTESIAN_POINT ( 'NONE',  ( -22.31427554260534052, 100.0000000000000284, -10.13077409178744404 ) ) ;
#7253=CARTESIAN_POINT ( 'NONE',  ( -15.26676860252058887, 99.49999999999998579, 16.38168943497750973 ) ) ;
#7254=CARTESIAN_POINT ( 'NONE',  ( -22.00707282958688182, 99.49999999999997158, -9.748971510896797810 ) ) ;
#7255=CARTESIAN_POINT ( 'NONE',  ( -27.00000000000000355, 2.549999997815050712, -11.18376618407357270 ) ) ;
#7256=CARTESIAN_POINT ( 'NONE',  ( -27.43301270000000969, 3.199999998907525622, 11.36312591709335784 ) ) ;
#7258=CARTESIAN_POINT ( 'NONE',  ( 4.277141017070624329, 99.50000000000002842, -21.57940364907851816 ) ) ;
#7260=CARTESIAN_POINT ( 'NONE',  ( 3.277744210708366079, 99.99999999999998579, -23.71256836663369327 ) ) ;
#7263=CARTESIAN_POINT ( 'NONE',  ( 19.39806930854667399, 5.049999998907525267, 19.39806930854668465 ) ) ;
#7264=CARTESIAN_POINT ( 'NONE',  ( -15.10687288066601930, 99.99999999999995737, 15.84109048427130517 ) ) ;
#7265=AXIS2_PLACEMENT_3D ( 'NONE', #8306, #8114, #4917 ) ;
#7266=DIRECTION ( 'NONE',  ( -0.8799640205556051864, 0.000000000000000000, -0.4750403377899758417 ) ) ;
#7269=PRODUCT ( 'Reservoir Tank', 'Reservoir Tank', '', ( #522 ) ) ;
#7272=CARTESIAN_POINT ( 'NONE',  ( 9.676361905416721143, 100.0000000000000142, 21.63547735782115566 ) ) ;
#7273=ORIENTED_EDGE ( 'NONE', *, *, #4019, .T. ) ;
#7275=VERTEX_POINT ( 'NONE', #5209 ) ;
#7277=CARTESIAN_POINT ( 'NONE',  ( -5.039362679103552881E-15, 4.049999998907525267, 27.43301270000000258 ) ) ;
#7278=CARTESIAN_POINT ( 'NONE',  ( 24.93339342948717885, 100.0000000000000000, -1.235376602564102644 ) ) ;
#7279=B_SPLINE_CURVE_WITH_KNOTS ( 'NONE', 3,
 ( #9339, #2169, #9124, #1943, #5138, #5352, #5970, #2726, #6126, #535, #5177, #2153, #9262, #8542, #6801 ),
 .UNSPECIFIED., .F., .F.,
 ( 4, 1, 1, 1, 1, 1, 1, 1, 1, 1, 1, 1, 4 ),
 ( 0.000000000000000000, 0.08450893420292937552, 0.1670077533940913517, 0.2489527561816328172, 0.3323249201989921797, 0.4152786837838207679, 0.4972150204155297848, 0.5791806016509544186, 0.6636863847498374325, 0.7483757861910059761, 0.8320455266939520422, 0.9153409992114193150, 1.000000000000000000 ),
 .UNSPECIFIED. ) ;
#7280=CARTESIAN_POINT ( 'NONE',  ( 27.00000000000000355, 4.849999999999999645, -11.18376618407356737 ) ) ;
#7281=CARTESIAN_POINT ( 'NONE',  ( -16.33590634957226229, 100.0000000000000000, 16.80570853669505382 ) ) ;
#7282=VERTEX_POINT ( 'NONE', #6889 ) ;
#7284=LINE ( 'NONE', #1776, #9409 ) ;
#7289=CARTESIAN_POINT ( 'NONE',  ( 3.538198506519217190, 99.49999999999998579, -24.58220198924426114 ) ) ;
#7290=CARTESIAN_POINT ( 'NONE',  ( 24.91446314102564230, 100.0000000000000000, -1.581029647435897578 ) ) ;
#7293=CARTESIAN_POINT ( 'NONE',  ( -22.69253165798458127, 99.50000000000001421, -10.28928739654909563 ) ) ;
#7299=ORIENTED_EDGE ( 'NONE', *, *, #8716, .T. ) ;
#7301=CARTESIAN_POINT ( 'NONE',  ( 3.712044765110731337, 99.99999999999998579, -21.08683700305641651 ) ) ;
#7303=CARTESIAN_POINT ( 'NONE',  ( -14.79004890936967875, 99.99999999999998579, 16.19006955939758541 ) ) ;
#7305=EDGE_LOOP ( 'NONE', ( #1235, #2836, #1423, #8219 ) ) ;
#7308=PLANE ( 'NONE',  #3970 ) ;
#7309=CARTESIAN_POINT ( 'NONE',  ( 8.612131858919537919, 99.99999999999998579, 19.96100069886393413 ) ) ;
#7310=EDGE_LOOP ( 'NONE', ( #8470, #3526, #3697, #6228 ) ) ;
#7311=CARTESIAN_POINT ( 'NONE',  ( 4.486604876299897349, 99.50000000000000000, -21.85617661337775885 ) ) ;
#7313=CARTESIAN_POINT ( 'NONE',  ( 3.573144549190039321, 99.49999999999998579, -23.04580706645134214 ) ) ;
#7314=CARTESIAN_POINT ( 'NONE',  ( 5.725936192474917696, 100.0000000000000000, 21.08018326417248645 ) ) ;
#7315=CARTESIAN_POINT ( 'NONE',  ( -20.88772068548257366, 100.0000000000000142, -11.14739719174079546 ) ) ;
#7316=CARTESIAN_POINT ( 'NONE',  ( 27.00000000000000355, 0.5999999978150503122, 0.000000000000000000 ) ) ;
#7317=CARTESIAN_POINT ( 'NONE',  ( 19.09188309203678102, 3.100000000000000533, 19.09188309203678813 ) ) ;
#7319=CARTESIAN_POINT ( 'NONE',  ( -15.49014769301379069, 99.49999999999997158, 16.56834637662448273 ) ) ;
#7321=VECTOR ( 'NONE', #7375, 1000.000000000000114 ) ;
#7327=CARTESIAN_POINT ( 'NONE',  ( 1.679787559701184688E-15, 5.283333332240858660, -27.43301270000000258 ) ) ;
#7328=ADVANCED_FACE ( 'NONE', ( #2130, #9192, #514, #5999, #10203, #1404, #1347, #6782 ), #403, .T. ) ;
#7329=CARTESIAN_POINT ( 'NONE',  ( 19.09188309203678102, 4.700000000000000178, 19.09188309203678813 ) ) ;
#7331=LINE ( 'NONE', #4340, #9624 ) ;
#7333=CARTESIAN_POINT ( 'NONE',  ( -20.89169796687544789, 99.50000000000001421, -10.40078880447404330 ) ) ;
#7335=CARTESIAN_POINT ( 'NONE',  ( 3.606694021351891877, 100.0000000000000000, -24.61315535935035115 ) ) ;
#7336=CARTESIAN_POINT ( 'NONE',  ( 3.701176614148623756, 99.50000000000000000, -24.64875008328975170 ) ) ;
#7340=CARTESIAN_POINT ( 'NONE',  ( -22.13144646319157260, 99.50000000000001421, -9.428651666388001118 ) ) ;
#7341=CARTESIAN_POINT ( 'NONE',  ( 4.988497440555089923, 100.0000000000000000, -24.29977663856455194 ) ) ;
#7342=EDGE_LOOP ( 'NONE', ( #6828, #3468, #1154, #4551 ) ) ;
#7343=ADVANCED_FACE ( 'NONE', ( #566 ), #10030, .F. ) ;
#7345=VERTEX_POINT ( 'NONE', #4485 ) ;
#7347=CARTESIAN_POINT ( 'NONE',  ( 3.446946945638383664, 99.49999999999997158, -21.53774374131874580 ) ) ;
#7348=CARTESIAN_POINT ( 'NONE',  ( -21.65488089977124275, 99.49999999999997158, -11.10326233039539723 ) ) ;
#7350=VERTEX_POINT ( 'NONE', #10147 ) ;
#7351=CARTESIAN_POINT ( 'NONE',  ( 8.231219904624582639, 99.50000000000000000, 20.21381436664452735 ) ) ;
#7353=CARTESIAN_POINT ( 'NONE',  ( -11.18376618407358336, 2.749999997815050445, 26.99999999999999645 ) ) ;
#7354=CARTESIAN_POINT ( 'NONE',  ( 4.363164797760430424, 99.50000000000002842, -21.67376679147534446 ) ) ;
#7355=EDGE_CURVE ( 'NONE', #8654, #9400, #7987, .T. ) ;
#7356=CARTESIAN_POINT ( 'NONE',  ( 3.689266881520847807, 99.99999999999997158, -22.97735580002706968 ) ) ;
#7357=CARTESIAN_POINT ( 'NONE',  ( 4.320351800798612807, 99.49999999999995737, -21.62386382141117736 ) ) ;
#7358=CARTESIAN_POINT ( 'NONE',  ( 3.341734429721257005, 99.50000000000000000, -22.34498040423979148 ) ) ;
#7359=CARTESIAN_POINT ( 'NONE',  ( 27.00000000000000355, 3.849999997815050534, -11.18376618407356737 ) ) ;
#7361=CARTESIAN_POINT ( 'NONE',  ( -21.59424432678268957, 99.49999999999997158, -9.639623801236600897 ) ) ;
#7363=CARTESIAN_POINT ( 'NONE',  ( -21.72555844818415594, 100.0000000000000142, -11.09629251537910655 ) ) ;
#7364=DIRECTION ( 'NONE',  ( 0.000000000000000000, 0.000000000000000000, -1.000000000000000000 ) ) ;
#7371=CARTESIAN_POINT ( 'NONE',  ( -5.039362679103552881E-15, 3.249999998907525001, 27.43301270000000258 ) ) ;
#7372=CARTESIAN_POINT ( 'NONE',  ( -20.61566945723384592, 100.0000000000000000, -10.83949095114527594 ) ) ;
#7374=LINE ( 'NONE', #8269, #3776 ) ;
#7375=DIRECTION ( 'NONE',  ( -0.8799640205556051864, 0.000000000000000000, -0.4750403377899757862 ) ) ;
#7376=CARTESIAN_POINT ( 'NONE',  ( 0.000000000000000000, 0.000000000000000000, -25.15000000000000213 ) ) ;
#7378=ORIENTED_EDGE ( 'NONE', *, *, #3637, .F. ) ;
#7379=( BOUNDED_CURVE ( )  B_SPLINE_CURVE ( 2, ( #4361, #1120, #3640, #4261, #9177, #7547, #5984, #1225, #1893 ),
 .UNSPECIFIED., .F., .T. ) 
 B_SPLINE_CURVE_WITH_KNOTS ( ( 3, 2, 2, 2, 3 ),
 ( 0.4642857142857143016, 0.4821428571428571508, 0.5000000000000000000, 0.5178571428571429047, 0.5357142857142856984 ),
 .UNSPECIFIED. ) 
 CURVE ( )  GEOMETRIC_REPRESENTATION_ITEM ( )  RATIONAL_B_SPLINE_CURVE ( ( 1.000000000000000000, 0.9238795325112867385, 1.000000000000000000, 0.9238795325112867385, 1.000000000000000000, 0.9238795325112867385, 1.000000000000000000, 0.9238795325112867385, 1.000000000000000000 ) ) 
 REPRESENTATION_ITEM ( '' )  );
#7380=CARTESIAN_POINT ( 'NONE',  ( -21.59614764830937972, 99.99999999999994316, -9.292069227195950631 ) ) ;
#7381=CARTESIAN_POINT ( 'NONE',  ( 19.39806930854668110, 4.349999998907525089, -19.39806930854668110 ) ) ;
#7382=CARTESIAN_POINT ( 'NONE',  ( -16.30857500771091040, 99.49999999999994316, 15.34700649443169063 ) ) ;
#7383=DIRECTION ( 'NONE',  ( -0.000000000000000000, 1.000000000000000000, -0.000000000000000000 ) ) ;
#7385=CARTESIAN_POINT ( 'NONE',  ( -16.60513711880302878, 100.0000000000000000, 15.15667007515659570 ) ) ;
#7386=CARTESIAN_POINT ( 'NONE',  ( 4.503533123526070270, 99.99999999999995737, -24.63026223303895890 ) ) ;
#7389=EDGE_LOOP ( 'NONE', ( #5434, #7943, #9288, #2481 ) ) ;
#7391=CARTESIAN_POINT ( 'NONE',  ( 0.000000000000000000, 85.00000000000000000, 0.000000000000000000 ) ) ;
#7392=CARTESIAN_POINT ( 'NONE',  ( 3.446946945638383664, 99.99999999999994316, -21.53774374131874580 ) ) ;
#7393=CARTESIAN_POINT ( 'NONE',  ( -14.97579057656165169, 100.0000000000000142, 16.56690896377573452 ) ) ;
#7394=CARTESIAN_POINT ( 'NONE',  ( 4.772556553149396308, 99.49999999999997158, -24.49721679606612312 ) ) ;
#7395=VECTOR ( 'NONE', #589, 1000.000000000000000 ) ;
#7396=CARTESIAN_POINT ( 'NONE',  ( -15.30066472929571653, 99.49999999999998579, 16.41738810589640707 ) ) ;
#7398=DIRECTION ( 'NONE',  ( -0.000000000000000000, -1.000000000000000000, -0.000000000000000000 ) ) ;
#7400=CARTESIAN_POINT ( 'NONE',  ( 3.080354370726382296, 100.0000000000000426, -23.09295995363041598 ) ) ;
#7402=CARTESIAN_POINT ( 'NONE',  ( 3.504547665631520648, 99.99999999999994316, -23.10026541809159184 ) ) ;
#7403=CARTESIAN_POINT ( 'NONE',  ( 8.393217272293057363, 99.50000000000000000, 19.69436072183531650 ) ) ;
#7405=CARTESIAN_POINT ( 'NONE',  ( 11.18376618407356915, 4.749999997815050001, -27.00000000000000355 ) ) ;
#7406=EDGE_CURVE ( 'NONE', #8654, #1114, #4651, .T. ) ;
#7407=LINE ( 'NONE', #8895, #5010 ) ;
#7408=CARTESIAN_POINT ( 'NONE',  ( -21.13452028402337035, 100.0000000000000000, -9.824917503107416294 ) ) ;
#7410=EDGE_CURVE ( 'NONE', #393, #6584, #6373, .T. ) ;
#7411=FACE_OUTER_BOUND ( 'NONE', #10310, .T. ) ;
#7412=DIRECTION ( 'NONE',  ( 0.05468478504300072068, 0.000000000000000000, 0.9985036676371302766 ) ) ;
#7413=DIRECTION ( 'NONE',  ( -0.000000000000000000, -1.000000000000000000, -0.000000000000000000 ) ) ;
#7414=ORIENTED_EDGE ( 'NONE', *, *, #1752, .T. ) ;
#7415=ORIENTED_EDGE ( 'NONE', *, *, #6350, .T. ) ;
#7418=CARTESIAN_POINT ( 'NONE',  ( -15.03963071504896121, 99.50000000000001421, 16.63526396357264758 ) ) ;
#7420=CARTESIAN_POINT ( 'NONE',  ( 1.679787559701184688E-15, 2.049999998907525711, -27.43301270000000258 ) ) ;
#7421=CARTESIAN_POINT ( 'NONE',  ( -4.959819536546781389E-15, 1.399999999999999911, 27.00000000000000355 ) ) ;
#7422=DIRECTION ( 'NONE',  ( 0.000000000000000000, 0.000000000000000000, -1.000000000000000000 ) ) ;
#7423=CARTESIAN_POINT ( 'NONE',  ( 4.723706824522782455, 100.0000000000000000, -24.08630974238606370 ) ) ;
#7424=CARTESIAN_POINT ( 'NONE',  ( 8.133363296361027395, 100.0000000000000426, 19.85287606700953233 ) ) ;
#7426=CARTESIAN_POINT ( 'NONE',  ( 7.812290123947159159, 99.49999999999998579, 21.17203503082402349 ) ) ;
#7427=FACE_OUTER_BOUND ( 'NONE', #691, .T. ) ;
#7431=CARTESIAN_POINT ( 'NONE',  ( 8.901217755223779449, 99.50000000000004263, 19.92336871027421097 ) ) ;
#7432=CARTESIAN_POINT ( 'NONE',  ( 3.764204346677844093, 99.50000000000001421, -22.52576385118515745 ) ) ;
#7433=LINE ( 'NONE', #4458, #5093 ) ;
#7436=ORIENTED_EDGE ( 'NONE', *, *, #9968, .F. ) ;
#7438=CARTESIAN_POINT ( 'NONE',  ( -22.55793349878803156, 100.0000000000000000, -10.88926985104519929 ) ) ;
#7439=CARTESIAN_POINT ( 'NONE',  ( 3.198592217420132666, 99.50000000000000000, -21.96964977087737836 ) ) ;
#7446=CARTESIAN_POINT ( 'NONE',  ( 4.232798786556307036, 99.50000000000000000, -24.34936571594186105 ) ) ;
#7447=CARTESIAN_POINT ( 'NONE',  ( 4.835062408351179286, 99.50000000000000000, -21.79588013901878440 ) ) ;
#7448=VERTEX_POINT ( 'NONE', #7949 ) ;
#7449=VECTOR ( 'NONE', #7413, 1000.000000000000000 ) ;
#7450=CARTESIAN_POINT ( 'NONE',  ( 21.47055288461538325, 99.50000000000000000, -0.7081330128205128860 ) ) ;
#7451=CARTESIAN_POINT ( 'NONE',  ( 27.43301269999999548, 4.299999998907526155, 11.36312591709337738 ) ) ;
#7455=CARTESIAN_POINT ( 'NONE',  ( 3.306546357697854128E-15, 100.0000000000000000, 27.00000000000000355 ) ) ;
#7456=CARTESIAN_POINT ( 'NONE',  ( 7.856939908706818798, 99.99999999999995737, 20.19612520319305560 ) ) ;
#7457=EDGE_CURVE ( 'NONE', #4244, #10122, #3141, .T. ) ;
#7459=CARTESIAN_POINT ( 'NONE',  ( 3.659868213429061878, 100.0000000000000284, -22.50687739797974274 ) ) ;
#7460=CARTESIAN_POINT ( 'NONE',  ( -11.18376618407358336, 2.749999997815050445, 26.99999999999999645 ) ) ;
#7461=CARTESIAN_POINT ( 'NONE',  ( 5.725936192474917696, 99.50000000000000000, 21.08018326417248645 ) ) ;
#7462=CYLINDRICAL_SURFACE ( 'NONE', #6988, 7.500000000000000000 ) ;
#7463=CARTESIAN_POINT ( 'NONE',  ( -21.86704275050744073, 100.0000000000000142, -11.06111336656620026 ) ) ;
#7464=CARTESIAN_POINT ( 'NONE',  ( 2.955068081869620666, 99.99999999999998579, -21.57801138750623338 ) ) ;
#7468=EDGE_CURVE ( 'NONE', #3208, #3431, #2114, .T. ) ;
#7469=CARTESIAN_POINT ( 'NONE',  ( -14.83571502646304197, 99.50000000000004263, 16.32397075880403392 ) ) ;
#7471=CARTESIAN_POINT ( 'NONE',  ( -27.43301270000000969, 1.499999998907525445, 11.36312591709335429 ) ) ;
#7473=CARTESIAN_POINT ( 'NONE',  ( -20.42657152723830905, 99.99999999999997158, -10.54129411626120216 ) ) ;
#7476=CARTESIAN_POINT ( 'NONE',  ( 9.820792995160308791, 100.0000000000000000, 20.21220011423140761 ) ) ;
#7479=CARTESIAN_POINT ( 'NONE',  ( -21.03505001771060634, 99.99999999999994316, -9.476849197711761263 ) ) ;
#7480=CARTESIAN_POINT ( 'NONE',  ( 3.409892249890944527, 100.0000000000000000, -24.50637943905448779 ) ) ;
#7481=( NAMED_UNIT ( * ) SI_UNIT ( $, .STERADIAN. ) SOLID_ANGLE_UNIT ( ) );
#7482=VECTOR ( 'NONE', #9913, 1000.000000000000000 ) ;
#7484=DIRECTION ( 'NONE',  ( -0.000000000000000000, -1.000000000000000000, -0.000000000000000000 ) ) ;
#7486=CARTESIAN_POINT ( 'NONE',  ( 9.554054106072296548, 99.50000000000001421, 20.45778517829714360 ) ) ;
#7487=CARTESIAN_POINT ( 'NONE',  ( -21.59424432678268957, 99.99999999999997158, -9.639623801236600897 ) ) ;
#7488=VERTEX_POINT ( 'NONE', #1020 ) ;
#7489=DIRECTION ( 'NONE',  ( -0.000000000000000000, 1.000000000000000000, -0.000000000000000000 ) ) ;
#7491=ORIENTED_EDGE ( 'NONE', *, *, #1160, .T. ) ;
#7493=CARTESIAN_POINT ( 'NONE',  ( 3.497829868842083023, 99.50000000000000000, -21.50512556757917793 ) ) ;
#7494=CARTESIAN_POINT ( 'NONE',  ( 3.277744210708366079, 99.50000000000001421, -23.71256836663369327 ) ) ;
#7496=CARTESIAN_POINT ( 'NONE',  ( -15.27171031718473770, 99.50000000000002842, 15.44886715306589764 ) ) ;
#7499=PLANE ( 'NONE',  #7623 ) ;
#7500=CARTESIAN_POINT ( 'NONE',  ( 9.468852706215191262, 100.0000000000000000, 21.22967007823213237 ) ) ;
#7502=B_SPLINE_CURVE_WITH_KNOTS ( 'NONE', 3,
 ( #6018, #1315, #2095, #8376, #6910, #371, #2944, #2887, #7529, #3674, #3507 ),
 .UNSPECIFIED., .F., .F.,
 ( 4, 1, 1, 1, 1, 1, 1, 1, 4 ),
 ( 0.000000000000000000, 0.1243175037779491315, 0.2437391319546453605, 0.3610119291759345539, 0.4796059399169178006, 0.5994854737745749507, 0.7252340722053824962, 0.8585022233306516259, 1.000000000000000000 ),
 .UNSPECIFIED. ) ;
#7504=CARTESIAN_POINT ( 'NONE',  ( -27.43301270000000969, 2.399999998907525356, 11.36312591709335429 ) ) ;
#7505=CARTESIAN_POINT ( 'NONE',  ( 3.739209042966563867, 99.50000000000000000, -21.42288334414699236 ) ) ;
#7506=CARTESIAN_POINT ( 'NONE',  ( 3.538198506519217190, 99.49999999999998579, -24.58220198924426114 ) ) ;
#7507=CARTESIAN_POINT ( 'NONE',  ( 7.913184448816831029, 99.99999999999994316, 20.09878816755126252 ) ) ;
#7509=CARTESIAN_POINT ( 'NONE',  ( 3.028692941384139026, 99.50000000000001421, -22.52214499033115302 ) ) ;
#7510=CARTESIAN_POINT ( 'NONE',  ( -27.00000000000001421, 5.049999997815051600, 11.18376618407356382 ) ) ;
#7512=CARTESIAN_POINT ( 'NONE',  ( -21.73488407773357167, 99.50000000000000000, -9.647150398373231184 ) ) ;
#7513=DIRECTION ( 'NONE',  ( 0.000000000000000000, 0.000000000000000000, 1.000000000000000000 ) ) ;
#7514=CARTESIAN_POINT ( 'NONE',  ( -22.20893716642541804, 99.50000000000002842, -10.81429252070940272 ) ) ;
#7515=CARTESIAN_POINT ( 'NONE',  ( 3.428579745388047328, 99.99999999999998579, -21.16399209792802694 ) ) ;
#7521=CARTESIAN_POINT ( 'NONE',  ( 2.924645347134957163, 100.0000000000000142, -23.60918035669702064 ) ) ;
#7522=CARTESIAN_POINT ( 'NONE',  ( -27.43301270000000258, 2.249999998907525001, -3.359575119402369376E-15 ) ) ;
#7523=CARTESIAN_POINT ( 'NONE',  ( 0.000000000000000000, 85.00000000000000000, 0.000000000000000000 ) ) ;
#7525=CARTESIAN_POINT ( 'NONE',  ( 7.156925775808251622, 100.0000000000000000, 23.91622092442889524 ) ) ;
#7526=DIRECTION ( 'NONE',  ( 0.000000000000000000, 0.000000000000000000, -1.000000000000000000 ) ) ;
#7527=EDGE_LOOP ( 'NONE', ( #5082, #909, #8173, #8979 ) ) ;
#7528=DIRECTION ( 'NONE',  ( -0.9567206510497618943, 0.000000000000000000, 0.2910078965507976179 ) ) ;
#7529=CARTESIAN_POINT ( 'NONE',  ( 3.298672054714395063, 100.0000000000000142, -22.72039518595936869 ) ) ;
#7532=SURFACE_STYLE_USAGE ( .BOTH. , #8177 ) ;
#7535=CARTESIAN_POINT ( 'NONE',  ( 3.873456569393397331, 99.50000000000002842, -22.53291374702356364 ) ) ;
#7536=CARTESIAN_POINT ( 'NONE',  ( -21.94169572595625795, 100.0000000000000000, -9.715372641902229489 ) ) ;
#7537=ORIENTED_EDGE ( 'NONE', *, *, #7111, .F. ) ;
#7538=DIRECTION ( 'NONE',  ( 0.000000000000000000, 0.000000000000000000, -1.000000000000000000 ) ) ;
#7539=EDGE_CURVE ( 'NONE', #9964, #4732, #4171, .T. ) ;
#7544=LINE ( 'NONE', #6761, #8651 ) ;
#7545=CARTESIAN_POINT ( 'NONE',  ( 3.739209042966563867, 99.99999999999997158, -21.42288334414699236 ) ) ;
#7547=CARTESIAN_POINT ( 'NONE',  ( -27.00000000000001421, 3.449999997815051067, 11.18376618407356560 ) ) ;
#7548=AXIS2_PLACEMENT_3D ( 'NONE', #4221, #8349, #9086 ) ;
#7549=B_SPLINE_CURVE_WITH_KNOTS ( 'NONE', 3,
 ( #4202, #133, #8971, #7386, #4983, #3227, #6466, #2437, #2491, #7341, #4112, #6605, #870, #8182, #965, #1011, #225, #1697, #5632 ),
 .UNSPECIFIED., .F., .F.,
 ( 4, 1, 1, 1, 1, 1, 1, 1, 1, 1, 1, 1, 1, 1, 1, 1, 4 ),
 ( 0.000000000000000000, 0.06533929434940796699, 0.1284421010879715219, 0.1894557237235162950, 0.2487158350925330053, 0.3070727012892665031, 0.3650088636856013702, 0.4229902474982629723, 0.4815891416229265420, 0.5404453987529589387, 0.6002338948610608238, 0.6608164219703346332, 0.7232441343194829786, 0.7881366429682739039, 0.8556965829275263724, 0.9259544997225339635, 1.000000000000000000 ),
 .UNSPECIFIED. ) ;
#7550=CARTESIAN_POINT ( 'NONE',  ( -15.13293277027690209, 99.50000000000000000, 16.13104881108577970 ) ) ;
#7551=CARTESIAN_POINT ( 'NONE',  ( 9.676361905416721143, 99.50000000000001421, 21.63547735782115566 ) ) ;
#7552=LINE ( 'NONE', #772, #4292 ) ;
#7553=CARTESIAN_POINT ( 'NONE',  ( 9.342627931057743140, 100.0000000000000000, 21.59831790269294771 ) ) ;
#7556=CARTESIAN_POINT ( 'NONE',  ( 19.09188309203678813, 1.499999997815050223, -19.09188309203678813 ) ) ;
#7557=CARTESIAN_POINT ( 'NONE',  ( 27.43301270000000258, 4.399999998907525800, -11.36312591709336139 ) ) ;
#7559=CARTESIAN_POINT ( 'NONE',  ( 9.861577898019769250, 99.49999999999995737, 21.03794551367759169 ) ) ;
#7560=CARTESIAN_POINT ( 'NONE',  ( 11.18376618407357093, 4.749999997815051778, -27.00000000000000355 ) ) ;
#7562=LINE ( 'NONE', #3596, #4602 ) ;
#7563=CARTESIAN_POINT ( 'NONE',  ( 26.99999999999999645, 3.749999997815050445, 11.18376618407358691 ) ) ;
#7569=CARTESIAN_POINT ( 'NONE',  ( 4.887668416326221177, 100.0000000000000142, -23.70513093767710089 ) ) ;
#7570=CARTESIAN_POINT ( 'NONE',  ( 27.43301270000000258, 0.3999999989075253559, -11.36312591709336139 ) ) ;
#7574=CARTESIAN_POINT ( 'NONE',  ( -14.89910828679519739, 99.49999999999997158, 16.44921749203638939 ) ) ;
#7576=CARTESIAN_POINT ( 'NONE',  ( 11.36312591709336850, 1.699999998907525400, 27.43301269999999903 ) ) ;
#7578=EDGE_LOOP ( 'NONE', ( #9923, #598, #4843, #6124 ) ) ;
#7579=EDGE_CURVE ( 'NONE', #4720, #2877, #931, .T. ) ;
#7580=CARTESIAN_POINT ( 'NONE',  ( -16.11976138926855739, 99.99999999999997158, 16.60078749809536447 ) ) ;
#7581=CARTESIAN_POINT ( 'NONE',  ( 6.477538756577482459, 100.0000000000000000, 20.49684993083915430 ) ) ;
#7582=CARTESIAN_POINT ( 'NONE',  ( 4.739008722453744049, 99.50000000000001421, -24.06821587619827696 ) ) ;
#7583=DIRECTION ( 'NONE',  ( -0.000000000000000000, -1.000000000000000000, -0.000000000000000000 ) ) ;
#7584=CARTESIAN_POINT ( 'NONE',  ( -21.11719860449141351, 99.50000000000002842, -9.425423427278841970 ) ) ;
#7585=CARTESIAN_POINT ( 'NONE',  ( 4.835062408351179286, 100.0000000000000000, -21.79588013901878440 ) ) ;
#7587=CARTESIAN_POINT ( 'NONE',  ( 0.000000000000000000, 100.0000000000000000, 18.00000000000000000 ) ) ;
#7588=CARTESIAN_POINT ( 'NONE',  ( -15.62751930918662069, 99.49999999999998579, 15.20915780906945436 ) ) ;
#7589=CARTESIAN_POINT ( 'NONE',  ( -16.38049141020750099, 99.50000000000004263, 14.97568473612765416 ) ) ;
#7590=CARTESIAN_POINT ( 'NONE',  ( 9.342627931057743140, 99.99999999999994316, 21.59831790269294771 ) ) ;
#7591=CARTESIAN_POINT ( 'NONE',  ( 3.058419780146050648, 99.50000000000000000, -23.12871267107006545 ) ) ;
#7592=ORIENTED_EDGE ( 'NONE', *, *, #7355, .F. ) ;
#7593=EDGE_CURVE ( 'NONE', #4302, #6802, #3376, .T. ) ;
#7594=CARTESIAN_POINT ( 'NONE',  ( 4.901590909071964042, 100.0000000000000000, -23.62641080846013608 ) ) ;
#7596=ORIENTED_EDGE ( 'NONE', *, *, #1580, .T. ) ;
#7597=CARTESIAN_POINT ( 'NONE',  ( 4.457146071884139360, 99.50000000000001421, -24.28472590373185724 ) ) ;
#7599=AXIS2_PLACEMENT_3D ( 'NONE', #4965, #5116, #9154 ) ;
#7600=CARTESIAN_POINT ( 'NONE',  ( 3.434779879277784609, 99.50000000000001421, -23.17575050830969374 ) ) ;
#7602=EDGE_CURVE ( 'NONE', #2877, #4679, #5886, .T. ) ;
#7605=ORIENTED_EDGE ( 'NONE', *, *, #9018, .F. ) ;
#7606=CARTESIAN_POINT ( 'NONE',  ( -4.959819536546781389E-15, 1.999999997815050445, 27.00000000000000355 ) ) ;
#7607=CARTESIAN_POINT ( 'NONE',  ( -27.00000000000000355, 1.149999999999999689, -11.18376618407357270 ) ) ;
#7610=CARTESIAN_POINT ( 'NONE',  ( 4.486604876299897349, 99.50000000000000000, -21.85617661337775885 ) ) ;
#7611=CARTESIAN_POINT ( 'NONE',  ( -27.43301270000000969, 3.999999998907525001, 11.36312591709335429 ) ) ;
#7612=CARTESIAN_POINT ( 'NONE',  ( -18.01369080470046313, 99.50000000000000000, 17.15556831233607937 ) ) ;
#7613=DIRECTION ( 'NONE',  ( -0.000000000000000000, 1.000000000000000000, -0.000000000000000000 ) ) ;
#7614=VECTOR ( 'NONE', #1283, 1000.000000000000227 ) ;
#7615=CARTESIAN_POINT ( 'NONE',  ( 9.164845778125666698, 99.50000000000001421, 19.62003801130714820 ) ) ;
#7619=VERTEX_POINT ( 'NONE', #5786 ) ;
#7620=FACE_OUTER_BOUND ( 'NONE', #4683, .T. ) ;
#7621=CARTESIAN_POINT ( 'NONE',  ( 19.39806930854668110, 0.4499999989075251783, -19.39806930854668110 ) ) ;
#7622=ORIENTED_EDGE ( 'NONE', *, *, #2573, .T. ) ;
#7623=AXIS2_PLACEMENT_3D ( 'NONE', #2599, #2746, #1952 ) ;
#7624=AXIS2_PLACEMENT_3D ( 'NONE', #1894, #4993, #1750 ) ;
#7629=CARTESIAN_POINT ( 'NONE',  ( 4.906732565843439531, 99.50000000000001421, -23.57187248890526376 ) ) ;
#7630=CARTESIAN_POINT ( 'NONE',  ( 11.36312591709336139, 3.699999998907525622, -27.43301270000000258 ) ) ;
#7631=ORIENTED_EDGE ( 'NONE', *, *, #6677, .F. ) ;
#7632=CARTESIAN_POINT ( 'NONE',  ( 8.644881627383616873, 99.99999999999995737, 19.60534525227960145 ) ) ;
#7634=CARTESIAN_POINT ( 'NONE',  ( 4.054941747578200584, 99.49999999999998579, -24.36678493958047298 ) ) ;
#7635=CARTESIAN_POINT ( 'NONE',  ( 7.729958523985794194, 100.0000000000000142, 20.63140804260154937 ) ) ;
#7636=CARTESIAN_POINT ( 'NONE',  ( 0.000000000000000000, 87.00000000000001421, -7.500000000000000000 ) ) ;
#7639=VERTEX_POINT ( 'NONE', #2645 ) ;
#7641=LINE ( 'NONE', #537, #6964 ) ;
#7642=CARTESIAN_POINT ( 'NONE',  ( -19.39806930854668465, 2.349999998907525534, 19.39806930854667755 ) ) ;
#7645=ORIENTED_EDGE ( 'NONE', *, *, #2850, .T. ) ;
#7646=LINE ( 'NONE', #4566, #3582 ) ;
#7647=CARTESIAN_POINT ( 'NONE',  ( 9.576498344683301411, 99.99999999999992895, 20.78592410672095880 ) ) ;
#7648=AXIS2_PLACEMENT_3D ( 'NONE', #844, #4035, #4870 ) ;
#7650=ORIENTED_EDGE ( 'NONE', *, *, #956, .T. ) ;
#7651=CARTESIAN_POINT ( 'NONE',  ( -16.24524625128438515, 99.50000000000002842, 16.53274063862002308 ) ) ;
#7653=EDGE_LOOP ( 'NONE', ( #5863, #4940 ) ) ;
#7654=VECTOR ( 'NONE', #3239, 1000.000000000000114 ) ;
#7655=CARTESIAN_POINT ( 'NONE',  ( 4.232798786556307036, 99.50000000000000000, -24.34936571594186105 ) ) ;
#7657=LINE ( 'NONE', #550, #727 ) ;
#7658=EDGE_CURVE ( 'NONE', #1454, #8208, #9029, .T. ) ;
#7660=CARTESIAN_POINT ( 'NONE',  ( 2.958578797724396026, 100.0000000000000000, -23.36432507653281121 ) ) ;
#7661=EDGE_LOOP ( 'NONE', ( #1735, #1174, #7622, #4282 ) ) ;
#7662=B_SPLINE_CURVE_WITH_KNOTS ( 'NONE', 3,
 ( #8805, #803, #7327, #63 ),
 .UNSPECIFIED., .F., .F.,
 ( 4, 4 ),
 ( 0.000000000000000000, 1.000000000000000000 ),
 .UNSPECIFIED. ) ;
#7663=CARTESIAN_POINT ( 'NONE',  ( 4.295198626299898237, 99.50000000000001421, -24.68029520312135361 ) ) ;
#7664=CARTESIAN_POINT ( 'NONE',  ( -19.75840245672548789, 100.0000000000000000, -8.735905494466331689 ) ) ;
#7665=CARTESIAN_POINT ( 'NONE',  ( 0.000000000000000000, 100.0000000000000000, 0.000000000000000000 ) ) ;
#7666=VERTEX_POINT ( 'NONE', #286 ) ;
#7667=LINE ( 'NONE', #9918, #3241 ) ;
#7668=CARTESIAN_POINT ( 'NONE',  ( -27.43301270000000258, 3.099999998907525089, -11.36312591709336317 ) ) ;
#7670=CARTESIAN_POINT ( 'NONE',  ( 9.820792995160310568, 99.50000000000001421, 20.21220011423141116 ) ) ;
#7672=VERTEX_POINT ( 'NONE', #3478 ) ;
#7674=CARTESIAN_POINT ( 'NONE',  ( 5.243816414761435674, 99.50000000000000000, -23.48558366465980995 ) ) ;
#7677=B_SPLINE_CURVE_WITH_KNOTS ( 'NONE', 3,
 ( #8644, #4661, #4549, #10159, #6172, #5507, #7851, #1305, #681, #3717, #6284, #4495, #9481, #9309, #2141, #5399, #8696, #2307, #1357 ),
 .UNSPECIFIED., .F., .F.,
 ( 4, 1, 1, 1, 1, 1, 1, 1, 1, 1, 1, 1, 1, 1, 1, 1, 4 ),
 ( 0.000000000000000000, 0.06363772181477481138, 0.1253661190162797812, 0.1854850957718461035, 0.2454326483351531030, 0.3054881917026986415, 0.3659564384638642753, 0.4275766838088623234, 0.4913505196498278993, 0.5556437034595619329, 0.6183735394983103095, 0.6802114403575724166, 0.7422401234104337719, 0.8041288543812358247, 0.8678488776753463529, 0.9326351893241184854, 1.000000000000000000 ),
 .UNSPECIFIED. ) ;
#7678=ORIENTED_EDGE ( 'NONE', *, *, #2551, .F. ) ;
#7679=CARTESIAN_POINT ( 'NONE',  ( 9.248677610544923766, 100.0000000000000000, 22.83089001807756446 ) ) ;
#7680=CARTESIAN_POINT ( 'NONE',  ( -5.039362679103552881E-15, 0.9499999989075252893, 27.43301270000000258 ) ) ;
#7681=EDGE_CURVE ( 'NONE', #5894, #728, #6664, .T. ) ;
#7684=CARTESIAN_POINT ( 'NONE',  ( -22.33111803333905243, 99.49999999999997158, -9.558150950182401573 ) ) ;
#7685=CARTESIAN_POINT ( 'NONE',  ( 0.000000000000000000, 100.0000000000000000, 0.000000000000000000 ) ) ;
#7687=CARTESIAN_POINT ( 'NONE',  ( 11.36312591709336139, 4.399999998907525800, -27.43301270000000258 ) ) ;
#7688=CARTESIAN_POINT ( 'NONE',  ( 19.39806930854667399, 1.049999998907525045, 19.39806930854668465 ) ) ;
#7689=ORIENTED_EDGE ( 'NONE', *, *, #7457, .T. ) ;
#7693=CARTESIAN_POINT ( 'NONE',  ( 3.203979444200292015, 99.50000000000000000, -21.29640115293693725 ) ) ;
#7694=CARTESIAN_POINT ( 'NONE',  ( 3.296462644833695776, 100.0000000000000142, -23.81854410834942115 ) ) ;
#7696=ORIENTED_EDGE ( 'NONE', *, *, #6983, .F. ) ;
#7698=CARTESIAN_POINT ( 'NONE',  ( 4.793167276645844410, 99.49999999999998579, -21.69837440717521204 ) ) ;
#7701=CARTESIAN_POINT ( 'NONE',  ( 19.39806930854668110, 1.149999998907525356, -19.39806930854668110 ) ) ;
#7703=EDGE_LOOP ( 'NONE', ( #4770, #7631, #5488, #3191 ) ) ;
#7704=CARTESIAN_POINT ( 'NONE',  ( 1.670949432750432147E-15, 5.166666665938350000, -27.28867513333333505 ) ) ;
#7705=CARTESIAN_POINT ( 'NONE',  ( -27.00000000000001421, 0.4500000000000000666, 11.18376618407356382 ) ) ;
#7706=CARTESIAN_POINT ( 'NONE',  ( 9.482997300390421103, 100.0000000000000284, 20.28643943712827991 ) ) ;
#7709=CARTESIAN_POINT ( 'NONE',  ( 4.829054701479813083, 100.0000000000000000, -23.91032069601275367 ) ) ;
#7711=VERTEX_POINT ( 'NONE', #9081 ) ;
#7712=DIRECTION ( 'NONE',  ( -0.000000000000000000, -1.000000000000000000, -0.000000000000000000 ) ) ;
#7713=CARTESIAN_POINT ( 'NONE',  ( -21.66466628782423243, 99.50000000000001421, -9.640935998098070669 ) ) ;
#7715=CARTESIAN_POINT ( 'NONE',  ( 5.047889085735837611, 99.50000000000001421, -24.22022158424849536 ) ) ;
#7716=VECTOR ( 'NONE', #1820, 1000.000000000000000 ) ;
#7717=EDGE_CURVE ( 'NONE', #8640, #224, #1896, .T. ) ;
#7720=CARTESIAN_POINT ( 'NONE',  ( 11.18376618407357093, 0.9499999999999999556, -27.00000000000000355 ) ) ;
#7721=( BOUNDED_CURVE ( )  B_SPLINE_CURVE ( 2, ( #2700, #6041, #9231, #2805, #2063, #5257, #7556, #4475, #6721 ),
 .UNSPECIFIED., .F., .F. ) 
 B_SPLINE_CURVE_WITH_KNOTS ( ( 3, 2, 2, 2, 3 ),
 ( 0.1071428571428571369, 0.1250000000000000000, 0.1428571428571428492, 0.1607142857142857262, 0.1785714285714285754 ),
 .UNSPECIFIED. ) 
 CURVE ( )  GEOMETRIC_REPRESENTATION_ITEM ( )  RATIONAL_B_SPLINE_CURVE ( ( 1.000000000000000000, 0.9238795325112867385, 1.000000000000000000, 0.9238795325112867385, 1.000000000000000000, 0.9238795325112867385, 1.000000000000000000, 0.9238795325112867385, 1.000000000000000000 ) ) 
 REPRESENTATION_ITEM ( '' )  );
#7723=PLANE ( 'NONE',  #730 ) ;
#7727=CARTESIAN_POINT ( 'NONE',  ( 9.834295043520187463, 99.50000000000002842, 21.14079655679390513 ) ) ;
#7728=VERTEX_POINT ( 'NONE', #499 ) ;
#7729=DIRECTION ( 'NONE',  ( 0.3368601548094422582, 0.000000000000000000, -0.9415546909775122097 ) ) ;
#7730=CARTESIAN_POINT ( 'NONE',  ( 5.098880966732203035, 99.50000000000000000, -24.13374913903897223 ) ) ;
#7731=CARTESIAN_POINT ( 'NONE',  ( -22.57971655928959365, 100.0000000000000000, -10.84768434062017839 ) ) ;
#7734=ORIENTED_EDGE ( 'NONE', *, *, #2031, .F. ) ;
#7735=CARTESIAN_POINT ( 'NONE',  ( -15.43596444985078975, 99.50000000000002842, 15.30036492734783593 ) ) ;
#7736=CARTESIAN_POINT ( 'NONE',  ( -27.43301270000000258, 0.6999999989075252893, -11.36312591709336317 ) ) ;
#7740=LINE ( 'NONE', #573, #1861 ) ;
#7741=CARTESIAN_POINT ( 'NONE',  ( 2.864934851235464208, 99.50000000000000000, -21.80148171563692827 ) ) ;
#7743=EDGE_CURVE ( 'NONE', #5515, #4002, #6877, .T. ) ;
#7745=CARTESIAN_POINT ( 'NONE',  ( 11.36312591709336139, 2.899999998907526244, -27.43301270000000258 ) ) ;
#7748=ORIENTED_EDGE ( 'NONE', *, *, #5916, .F. ) ;
#7750=CARTESIAN_POINT ( 'NONE',  ( -16.05266356869597644, 100.0000000000000000, 16.62382211633880047 ) ) ;
#7751=LINE ( 'NONE', #3000, #2809 ) ;
#7752=CARTESIAN_POINT ( 'NONE',  ( -16.63177974700816009, 99.50000000000000000, 16.59747536361813403 ) ) ;
#7753=CARTESIAN_POINT ( 'NONE',  ( 3.735769352376668184, 99.99999999999998579, -24.30643046864489420 ) ) ;
#7757=EDGE_LOOP ( 'NONE', ( #7898, #1399, #8449, #2714 ) ) ;
#7759=CARTESIAN_POINT ( 'NONE',  ( 27.43301270000000258, 1.899999998907525134, -11.36312591709336139 ) ) ;
#7760=VERTEX_POINT ( 'NONE', #5316 ) ;
#7762=CARTESIAN_POINT ( 'NONE',  ( -4.959819536546781389E-15, 2.200000000000000178, 27.00000000000000355 ) ) ;
#7763=CARTESIAN_POINT ( 'NONE',  ( 9.182805720491336032, 99.50000000000000000, 20.00174565872165289 ) ) ;
#7766=CARTESIAN_POINT ( 'NONE',  ( -16.49419651247312046, 99.49999999999998579, 15.57134447358898477 ) ) ;
#7767=CARTESIAN_POINT ( 'NONE',  ( -15.31787750341841559, 99.50000000000000000, 16.43551622900274722 ) ) ;
#7769=VERTEX_POINT ( 'NONE', #7606 ) ;
#7770=CARTESIAN_POINT ( 'NONE',  ( 0.000000000000000000, 87.00000000000001421, 0.000000000000000000 ) ) ;
#7771=PLANE ( 'NONE',  #2202 ) ;
#7774=CARTESIAN_POINT ( 'NONE',  ( 3.411785164761435674, 100.0000000000000000, -22.76693382491622231 ) ) ;
#7777=CARTESIAN_POINT ( 'NONE',  ( -16.85368146453285831, 99.99999999999998579, 16.27421966797335529 ) ) ;
#7781=EDGE_CURVE ( 'NONE', #9021, #669, #5089, .T. ) ;
#7783=CARTESIAN_POINT ( 'NONE',  ( -21.20585021321354802, 100.0000000000000568, -9.381045134209834657 ) ) ;
#7784=CARTESIAN_POINT ( 'NONE',  ( 9.263267005978743640, 99.49999999999998579, 19.65676951151765905 ) ) ;
#7787=( BOUNDED_CURVE ( )  B_SPLINE_CURVE ( 2, ( #8958, #4832, #5622, #5021, #1734, #8218, #4927, #5675, #216 ),
 .UNSPECIFIED., .F., .F. ) 
 B_SPLINE_CURVE_WITH_KNOTS ( ( 3, 2, 2, 2, 3 ),
 ( 0.2500000000000000000, 0.2678571428571428492, 0.2857142857142856984, 0.3035714285714285476, 0.3214285714285714524 ),
 .UNSPECIFIED. ) 
 CURVE ( )  GEOMETRIC_REPRESENTATION_ITEM ( )  RATIONAL_B_SPLINE_CURVE ( ( 1.000000000000000000, 0.9238795325112867385, 1.000000000000000000, 0.9238795325112867385, 1.000000000000000000, 0.9238795325112867385, 1.000000000000000000, 0.9238795325112867385, 1.000000000000000000 ) ) 
 REPRESENTATION_ITEM ( '' )  );
#7788=DIRECTION ( 'NONE',  ( -0.000000000000000000, -1.000000000000000000, -0.000000000000000000 ) ) ;
#7789=VERTEX_POINT ( 'NONE', #9967 ) ;
#7790=CARTESIAN_POINT ( 'NONE',  ( -15.32348647777738826, 100.0000000000000000, 15.39505148541300450 ) ) ;
#7791=CARTESIAN_POINT ( 'NONE',  ( 9.248677610544923766, 99.50000000000000000, 22.83089001807756446 ) ) ;
#7792=ORIENTED_EDGE ( 'NONE', *, *, #7658, .F. ) ;
#7794=EDGE_CURVE ( 'NONE', #3612, #1490, #6150, .T. ) ;
#7795=CARTESIAN_POINT ( 'NONE',  ( 3.681717055787076642, 99.99999999999997158, -21.09125273517263111 ) ) ;
#7797=CARTESIAN_POINT ( 'NONE',  ( 1.653273178848927064E-15, 0.7999999978150503788, -27.00000000000000355 ) ) ;
#7798=CARTESIAN_POINT ( 'NONE',  ( 27.43301270000000258, 1.149999998907525356, 0.000000000000000000 ) ) ;
#7800=CARTESIAN_POINT ( 'NONE',  ( -16.30427144417478402, 99.99999999999998579, 16.48895498912494517 ) ) ;
#7802=CARTESIAN_POINT ( 'NONE',  ( 3.231466532446834350, 99.49999999999997158, -21.81145066552309686 ) ) ;
#7803=CARTESIAN_POINT ( 'NONE',  ( -16.12578516900833137, 100.0000000000000142, 15.23469143358620492 ) ) ;
#7804=VECTOR ( 'NONE', #2972, 1000.000000000000000 ) ;
#7807=CARTESIAN_POINT ( 'NONE',  ( 4.504418077186241653, 99.50000000000004263, -21.31258943653750393 ) ) ;
#7808=ORIENTED_EDGE ( 'NONE', *, *, #5959, .F. ) ;
#7809=VERTEX_POINT ( 'NONE', #6989 ) ;
#7811=CARTESIAN_POINT ( 'NONE',  ( -11.36312591709337383, 3.199999998907524734, 27.43301269999999548 ) ) ;
#7813=EDGE_CURVE ( 'NONE', #3209, #7282, #1227, .T. ) ;
#7814=AXIS2_PLACEMENT_3D ( 'NONE', #5349, #476, #8538 ) ;
#7816=CARTESIAN_POINT ( 'NONE',  ( 27.00000000000000355, 0.000000000000000000, 0.000000000000000000 ) ) ;
#7817=CARTESIAN_POINT ( 'NONE',  ( 9.482997300390421103, 99.50000000000000000, 20.28643943712827991 ) ) ;
#7818=VERTEX_POINT ( 'NONE', #2799 ) ;
#7819=VERTEX_POINT ( 'NONE', #4582 ) ;
#7820=CARTESIAN_POINT ( 'NONE',  ( -15.15871127190382417, 99.50000000000000000, 15.63231653451427761 ) ) ;
#7821=CARTESIAN_POINT ( 'NONE',  ( 8.467217662126737210, 99.50000000000001421, 20.02246181083229004 ) ) ;
#7823=ORIENTED_EDGE ( 'NONE', *, *, #7794, .T. ) ;
#7825=FACE_BOUND ( 'NONE', #5526, .T. ) ;
#7829=CARTESIAN_POINT ( 'NONE',  ( 2.940192896829773250, 100.0000000000000142, -23.44521981770616037 ) ) ;
#7831=VECTOR ( 'NONE', #9257, 1000.000000000000000 ) ;
#7833=CARTESIAN_POINT ( 'NONE',  ( 4.386516977709190357, 99.50000000000004263, -24.31220192127581825 ) ) ;
#7838=ORIENTED_EDGE ( 'NONE', *, *, #385, .F. ) ;
#7839=CARTESIAN_POINT ( 'NONE',  ( -20.82968571475833031, 100.0000000000000142, -9.677916414284339908 ) ) ;
#7840=CARTESIAN_POINT ( 'NONE',  ( 8.644881627383616873, 99.49999999999995737, 19.60534525227960145 ) ) ;
#7843=DIRECTION ( 'NONE',  ( -0.9985315370676781654, 0.000000000000000000, 0.05417351272771728926 ) ) ;
#7844=ORIENTED_EDGE ( 'NONE', *, *, #3252, .T. ) ;
#7846=CARTESIAN_POINT ( 'NONE',  ( -11.36312591709335962, 3.799999998907525711, -27.43301270000000258 ) ) ;
#7849=CARTESIAN_POINT ( 'NONE',  ( 6.477538756577482459, 99.50000000000000000, 20.49684993083915430 ) ) ;
#7851=CARTESIAN_POINT ( 'NONE',  ( -16.88522588321459494, 99.50000000000002842, 16.18266969485829421 ) ) ;
#7852=CARTESIAN_POINT ( 'NONE',  ( 19.39806930854667399, 3.449999998907525622, 19.39806930854668465 ) ) ;
#7854=CARTESIAN_POINT ( 'NONE',  ( -15.10617644529808423, 100.0000000000000000, 15.98944417891004477 ) ) ;
#7856=CARTESIAN_POINT ( 'NONE',  ( 3.638175769014108774, 99.49999999999998579, -21.10017783766535970 ) ) ;
#7858=B_SPLINE_SURFACE_WITH_KNOTS ( 'NONE', 3, 1, ( 
 ( #8761, #597 ),
 ( #756, #1586 ),
 ( #7821, #4778 ),
 ( #3121, #7974 ),
 ( #6247, #10287 ),
 ( #8664, #650 ),
 ( #7030, #1533 ),
 ( #807, #5421 ),
 ( #4729, #10338 ),
 ( #3793, #4001 ),
 ( #8611, #2277 ),
 ( #7922, #4571 ),
 ( #10120, #1487 ),
 ( #4681, #1435 ),
 ( #6138, #7082 ),
 ( #6305, #3169 ),
 ( #5364, #2163 ),
 ( #3948, #6978 ),
 ( #8553, #9502 ) ),
 .UNSPECIFIED., .F., .F., .F.,
 ( 4, 1, 1, 1, 1, 1, 1, 1, 1, 1, 1, 1, 1, 1, 1, 1, 4 ),
 ( 2, 2 ),
 ( 0.000000000000000000, 0.06282509715607415002, 0.1231380613775250599, 0.1822388757841713336, 0.2396184841454026548, 0.2973605923678978580, 0.3541959668311244203, 0.4122907788200148582, 0.4717534157231769720, 0.5322282553174864095, 0.5926403291039165078, 0.6546871955647078911, 0.7179012776534754448, 0.7839155840457150415, 0.8527518695723632636, 0.9242989153657757972, 1.000000000000000000 ),
 ( 0.000000000000000000, 1.000000000000000000 ),
 .UNSPECIFIED. ) ;
#7859=CARTESIAN_POINT ( 'NONE',  ( 27.00000000000000355, 4.049999999999999822, -11.18376618407356915 ) ) ;
#7861=CARTESIAN_POINT ( 'NONE',  ( 3.712044765110731337, 99.99999999999998579, -21.08683700305641651 ) ) ;
#7862=ORIENTED_EDGE ( 'NONE', *, *, #7977, .T. ) ;
#7864=CARTESIAN_POINT ( 'NONE',  ( -5.039362679103552881E-15, 3.249999998907525001, 27.43301270000000258 ) ) ;
#7865=CARTESIAN_POINT ( 'NONE',  ( -15.84712739808237103, 99.49999999999997158, 14.83079670662049310 ) ) ;
#7866=CARTESIAN_POINT ( 'NONE',  ( 11.18376618407356915, 1.750000000000000222, -27.00000000000000355 ) ) ;
#7867=CARTESIAN_POINT ( 'NONE',  ( 9.513000527211589841, 100.0000000000000284, 20.35102222961602436 ) ) ;
#7868=ORIENTED_EDGE ( 'NONE', *, *, #4990, .T. ) ;
#7869=CARTESIAN_POINT ( 'NONE',  ( -16.56313167360273297, 99.50000000000002842, 16.06491815633068398 ) ) ;
#7870=CARTESIAN_POINT ( 'NONE',  ( -15.37123125604856710, 100.0000000000000142, 16.48683530611566539 ) ) ;
#7873=CARTESIAN_POINT ( 'NONE',  ( -5.039362679103552881E-15, 2.449999998907525178, 27.43301270000000258 ) ) ;
#7876=CARTESIAN_POINT ( 'NONE',  ( -27.00000000000001421, 3.650000000000000355, 11.18376618407356560 ) ) ;
#7877=CARTESIAN_POINT ( 'NONE',  ( 11.18376618407357626, 4.449999997815051067, 27.00000000000000000 ) ) ;
#7882=ORIENTED_EDGE ( 'NONE', *, *, #8426, .T. ) ;
#7883=CARTESIAN_POINT ( 'NONE',  ( 4.311343222282856047, 99.50000000000000000, -24.33387958695581688 ) ) ;
#7884=CARTESIAN_POINT ( 'NONE',  ( 3.061616997868383043E-15, 87.00000000000001421, 25.00000000000000000 ) ) ;
#7888=ORIENTED_EDGE ( 'NONE', *, *, #7579, .T. ) ;
#7890=VERTEX_POINT ( 'NONE', #1191 ) ;
#7891=CARTESIAN_POINT ( 'NONE',  ( 2.924645347134957163, 99.50000000000001421, -23.60918035669702064 ) ) ;
#7892=CARTESIAN_POINT ( 'NONE',  ( 9.725694684612619767, 99.50000000000000000, 20.03234812723199454 ) ) ;
#7896=CARTESIAN_POINT ( 'NONE',  ( -16.34436021381890924, 99.50000000000000000, 15.38072013554846151 ) ) ;
#7897=CARTESIAN_POINT ( 'NONE',  ( -27.43301270000000258, 3.899999998907525800, -11.36312591709336317 ) ) ;
#7898=ORIENTED_EDGE ( 'NONE', *, *, #6836, .F. ) ;
#7901=CARTESIAN_POINT ( 'NONE',  ( 3.293841816516395848, 99.99999999999995737, -23.44781013845121009 ) ) ;
#7903=CARTESIAN_POINT ( 'NONE',  ( 3.659868213429061878, 99.50000000000000000, -22.50687739797974274 ) ) ;
#7904=CARTESIAN_POINT ( 'NONE',  ( 1.679787559701184688E-15, 4.549999998907526155, -27.43301270000000258 ) ) ;
#7906=CARTESIAN_POINT ( 'NONE',  ( 0.000000000000000000, 87.00000000000001421, 0.000000000000000000 ) ) ;
#7907=CARTESIAN_POINT ( 'NONE',  ( 3.349514647153394975, 99.49999999999998579, -23.95461210612682024 ) ) ;
#7908=CARTESIAN_POINT ( 'NONE',  ( 3.497829868842083023, 99.50000000000000000, -21.50512556757917793 ) ) ;
#7911=CARTESIAN_POINT ( 'NONE',  ( -21.20585021321354802, 99.50000000000005684, -9.381045134209834657 ) ) ;
#7912=ORIENTED_EDGE ( 'NONE', *, *, #8577, .F. ) ;
#7914=CARTESIAN_POINT ( 'NONE',  ( 27.43301269999999548, 4.199999998907525622, 11.36312591709337738 ) ) ;
#7915=CARTESIAN_POINT ( 'NONE',  ( 9.513000527211589841, 99.50000000000000000, 20.35102222961602436 ) ) ;
#7917=EDGE_CURVE ( 'NONE', #776, #2013, #4404, .T. ) ;
#7918=CARTESIAN_POINT ( 'NONE',  ( -11.18376618407356560, 1.050000000000000044, -27.00000000000000355 ) ) ;
#7919=CARTESIAN_POINT ( 'NONE',  ( 9.502908418173033667, 99.50000000000000000, 20.32929868008965002 ) ) ;
#7922=CARTESIAN_POINT ( 'NONE',  ( 8.074269155311188939, 99.50000000000001421, 20.56111086218762551 ) ) ;
#7926=CARTESIAN_POINT ( 'NONE',  ( 27.00000000000000355, 0.000000000000000000, 0.000000000000000000 ) ) ;
#7927=CARTESIAN_POINT ( 'NONE',  ( 1.679787559701184688E-15, 2.849999998907525534, -27.43301270000000258 ) ) ;
#7928=CARTESIAN_POINT ( 'NONE',  ( -27.00000000000001421, 2.050000000000000266, 11.18376618407356560 ) ) ;
#7929=FACE_OUTER_BOUND ( 'NONE', #8740, .T. ) ;
#7932=ADVANCED_FACE ( 'NONE', ( #1038 ), #306, .T. ) ;
#7933=CARTESIAN_POINT ( 'NONE',  ( -16.63177974700816009, 99.50000000000000000, 16.59747536361813403 ) ) ;
#7934=DIRECTION ( 'NONE',  ( 0.000000000000000000, 0.000000000000000000, 1.000000000000000000 ) ) ;
#7935=ADVANCED_FACE ( 'NONE', ( #2712 ), #4020, .T. ) ;
#7937=VERTEX_POINT ( 'NONE', #6458 ) ;
#7940=ADVANCED_FACE ( 'NONE', ( #1642 ), #5849, .T. ) ;
#7943=ORIENTED_EDGE ( 'NONE', *, *, #9667, .F. ) ;
#7944=B_SPLINE_SURFACE_WITH_KNOTS ( 'NONE', 3, 1, ( 
 ( #3758, #3815 ),
 ( #2070, #5384 ),
 ( #1237, #4649 ),
 ( #7840, #10144 ),
 ( #671, #9190 ),
 ( #2980, #6161 ),
 ( #4429, #9359 ),
 ( #1401, #4593 ),
 ( #7615, #456 ),
 ( #7784, #616 ),
 ( #3652, #6998 ),
 ( #10202, #9468 ),
 ( #2298, #724 ),
 ( #10258, #4701 ),
 ( #3088, #3918 ),
 ( #7892, #5494 ),
 ( #6273, #8683 ),
 ( #1506, #210 ),
 ( #5015, #1198 ) ),
 .UNSPECIFIED., .F., .F., .F.,
 ( 4, 1, 1, 1, 1, 1, 1, 1, 1, 1, 1, 1, 1, 1, 1, 1, 4 ),
 ( 2, 2 ),
 ( 0.000000000000000000, 0.07024023345195122559, 0.1375772235014411093, 0.2026681864156774648, 0.2655894380381068620, 0.3279415367477454546, 0.3896445486312665740, 0.4521557380645868096, 0.5154465764363311830, 0.5785479733725392704, 0.6397241484143471046, 0.6996998702489094502, 0.7590513234224176564, 0.8180896689983322423, 0.8773873076253557723, 0.9378402036119877216, 1.000000000000000000 ),
 ( 0.000000000000000000, 1.000000000000000000 ),
 .UNSPECIFIED. ) ;
#7945=ORIENTED_EDGE ( 'NONE', *, *, #10016, .F. ) ;
#7946=PLANE ( 'NONE',  #8790 ) ;
#7947=VECTOR ( 'NONE', #2044, 1000.000000000000000 ) ;
#7949=CARTESIAN_POINT ( 'NONE',  ( -4.959819536546781389E-15, 2.200000000000000178, 27.00000000000000355 ) ) ;
#7950=DIRECTION ( 'NONE',  ( 0.000000000000000000, 0.000000000000000000, -1.000000000000000000 ) ) ;
#7952=ORIENTED_EDGE ( 'NONE', *, *, #1752, .F. ) ;
#7954=CARTESIAN_POINT ( 'NONE',  ( 3.563396934924631942, 100.0000000000000142, -22.47881610735839431 ) ) ;
#7956=CARTESIAN_POINT ( 'NONE',  ( -20.93486371557392545, 99.49999999999998579, -10.61231311368802466 ) ) ;
#7957=CARTESIAN_POINT ( 'NONE',  ( -11.18376618407356560, 1.649999997815050357, -27.00000000000000355 ) ) ;
#7958=VECTOR ( 'NONE', #1937, 1000.000000000000000 ) ;
#7959=CARTESIAN_POINT ( 'NONE',  ( -20.63200021313574695, 100.0000000000000000, -10.19493994959453431 ) ) ;
#7960=CARTESIAN_POINT ( 'NONE',  ( 10.85214315541671759, 100.0000000000000000, 22.51047735782115211 ) ) ;
#7961=CARTESIAN_POINT ( 'NONE',  ( -16.34021191015031249, 99.50000000000000000, 16.45483272884350967 ) ) ;
#7964=CARTESIAN_POINT ( 'NONE',  ( -20.82968571475833031, 99.50000000000001421, -9.677916414284339908 ) ) ;
#7965=ORIENTED_EDGE ( 'NONE', *, *, #874, .T. ) ;
#7968=CARTESIAN_POINT ( 'NONE',  ( -19.39806930854668465, 1.649999998907525356, 19.39806930854667755 ) ) ;
#7970=CARTESIAN_POINT ( 'NONE',  ( 27.00000000000000355, 3.200000000000000178, 0.000000000000000000 ) ) ;
#7973=CARTESIAN_POINT ( 'NONE',  ( -16.37547766376588854, 99.50000000000000000, 16.41943072543956816 ) ) ;
#7974=CARTESIAN_POINT ( 'NONE',  ( 8.399337394135656609, 99.99999999999998579, 20.06291166101774692 ) ) ;
#7977=EDGE_CURVE ( 'NONE', #7639, #6902, #9418, .T. ) ;
#7978=CARTESIAN_POINT ( 'NONE',  ( 11.36312591709336850, 3.299999998907525711, 27.43301269999999903 ) ) ;
#7979=CARTESIAN_POINT ( 'NONE',  ( 3.024867170474271116, 99.99999999999995737, -24.05477125543085748 ) ) ;
#7985=CARTESIAN_POINT ( 'NONE',  ( 1.653273178848927064E-15, 1.800000000000000266, -27.00000000000000355 ) ) ;
#7986=CARTESIAN_POINT ( 'NONE',  ( 19.09188309203678813, 5.499999997815050001, -19.09188309203678813 ) ) ;
#7987=B_SPLINE_CURVE_WITH_KNOTS ( 'NONE', 3,
 ( #2816, #6049, #2982, #6163, #9361, #3038, #1293, #5387, #8579, #9239, #4595, #2072, #6217, #5267, #9414, #8465, #4024, #5495, #2300 ),
 .UNSPECIFIED., .F., .F.,
 ( 4, 1, 1, 1, 1, 1, 1, 1, 1, 1, 1, 1, 1, 1, 1, 1, 4 ),
 ( 0.000000000000000000, 0.06442465027149940626, 0.1272622498775801414, 0.1890519169419207224, 0.2498421757728049863, 0.3110425729590077792, 0.3720985300252119266, 0.4351465435385043490, 0.5001170788027262670, 0.5644817420234762295, 0.6276143074669133792, 0.6889588046791949028, 0.7501592018653976401, 0.8106582772613761811, 0.8724479443257179279, 0.9351683423010851426, 1.000000000000000000 ),
 .UNSPECIFIED. ) ;
#7989=VERTEX_POINT ( 'NONE', #8583 ) ;
#7993=CARTESIAN_POINT ( 'NONE',  ( -22.24883010645271852, 99.49999999999997158, -10.75389422444101939 ) ) ;
#8001=CARTESIAN_POINT ( 'NONE',  ( 11.36312591709336139, 4.499999998907525445, -27.43301270000000258 ) ) ;
#8003=AXIS2_PLACEMENT_3D ( 'NONE', #6946, #7788, #2866 ) ;
#8005=CARTESIAN_POINT ( 'NONE',  ( -21.28703419482447146, 99.99999999999997158, -11.01737971290317297 ) ) ;
#8006=( BOUNDED_CURVE ( )  B_SPLINE_CURVE ( 2, ( #8048, #4073, #1510, #7255, #2302, #980, #6616, #7353, #9760 ),
 .UNSPECIFIED., .F., .T. ) 
 B_SPLINE_CURVE_WITH_KNOTS ( ( 3, 2, 2, 2, 3 ),
 ( 0.3214285714285714524, 0.3392857142857143016, 0.3571428571428571508, 0.3750000000000000000, 0.3928571428571428492 ),
 .UNSPECIFIED. ) 
 CURVE ( )  GEOMETRIC_REPRESENTATION_ITEM ( )  RATIONAL_B_SPLINE_CURVE ( ( 1.000000000000000000, 0.9238795325112867385, 1.000000000000000000, 0.9238795325112867385, 1.000000000000000000, 0.9238795325112867385, 1.000000000000000000, 0.9238795325112867385, 1.000000000000000000 ) ) 
 REPRESENTATION_ITEM ( '' )  );
#8008=CARTESIAN_POINT ( 'NONE',  ( -21.16695614262292580, 100.0000000000000000, -11.33496398805607441 ) ) ;
#8009=CARTESIAN_POINT ( 'NONE',  ( 26.99999999999999645, 2.149999997815051245, 11.18376618407358691 ) ) ;
#8010=UNCERTAINTY_MEASURE_WITH_UNIT (LENGTH_MEASURE( 1.000000000000000082E-05 ), #1005, 'distance_accuracy_value', 'NONE');
#8011=B_SPLINE_CURVE_WITH_KNOTS ( 'NONE', 3,
 ( #9895, #2931, #5823, #2731, #174, #6057, #1058, #9013, #9248, #5275, #8968, #6113, #7431, #272, #3464, #8474, #4492, #2678, #6653 ),
 .UNSPECIFIED., .F., .F.,
 ( 4, 1, 1, 1, 1, 1, 1, 1, 1, 1, 1, 1, 1, 1, 1, 1, 4 ),
 ( 0.000000000000000000, 0.06222907146265880401, 0.1227741760084055250, 0.1821991178386986321, 0.2415152369242211383, 0.3014228132391471027, 0.3622599083280184651, 0.4248173832850619669, 0.4890434280230284148, 0.5537961591902206271, 0.6173286602167864512, 0.6798064121185800612, 0.7417947397634444551, 0.8039614856828293243, 0.8674939867093949264, 0.9325113003366737319, 1.000000000000000000 ),
 .UNSPECIFIED. ) ;
#8012=CARTESIAN_POINT ( 'NONE',  ( -20.66709314808276332, 99.50000000000002842, -10.01107456535036455 ) ) ;
#8016=CARTESIAN_POINT ( 'NONE',  ( -22.13144646319157260, 100.0000000000000142, -9.428651666388001118 ) ) ;
#8019=ORIENTED_EDGE ( 'NONE', *, *, #5442, .T. ) ;
#8021=CARTESIAN_POINT ( 'NONE',  ( -27.43301270000000258, 1.499999998907525223, -11.36312591709336317 ) ) ;
#8024=CARTESIAN_POINT ( 'NONE',  ( 27.00000000000000355, 4.049999999999999822, -11.18376618407356737 ) ) ;
#8025=DIRECTION ( 'NONE',  ( 0.000000000000000000, 0.000000000000000000, -1.000000000000000000 ) ) ;
#8026=DIRECTION ( 'NONE',  ( 0.000000000000000000, 1.000000000000000000, -0.000000000000000000 ) ) ;
#8027=DIRECTION ( 'NONE',  ( -0.000000000000000000, 1.000000000000000000, -0.000000000000000000 ) ) ;
#8028=CARTESIAN_POINT ( 'NONE',  ( 6.477538756577482459, 99.50000000000000000, 20.49684993083915430 ) ) ;
#8029=VERTEX_POINT ( 'NONE', #6002 ) ;
#8030=CARTESIAN_POINT ( 'NONE',  ( -19.39806930854668465, 3.949999998907525178, 19.39806930854667755 ) ) ;
#8033=CARTESIAN_POINT ( 'NONE',  ( -22.57971655928959365, 100.0000000000000000, -10.84768434062017839 ) ) ;
#8035=CARTESIAN_POINT ( 'NONE',  ( -16.41302370085497131, 99.99999999999998579, 15.45185748370271206 ) ) ;
#8036=CARTESIAN_POINT ( 'NONE',  ( -16.91659681606879317, 99.50000000000000000, 15.78485274883190392 ) ) ;
#8037=CARTESIAN_POINT ( 'NONE',  ( 8.122452352567329115, 100.0000000000000000, 21.04970292111833530 ) ) ;
#8040=CARTESIAN_POINT ( 'NONE',  ( 4.280752963211088336, 99.99999999999997158, -21.16602454745684270 ) ) ;
#8041=CARTESIAN_POINT ( 'NONE',  ( -20.64578974631102426, 99.49999999999995737, -10.10077944494247504 ) ) ;
#8042=CARTESIAN_POINT ( 'NONE',  ( 9.725694684612619767, 99.50000000000000000, 20.03234812723199454 ) ) ;
#8044=B_SPLINE_CURVE_WITH_KNOTS ( 'NONE', 3,
 ( #4922, #8710, #8755, #3260, #6398, #6449, #1579, #8857, #4143, #162, #902 ),
 .UNSPECIFIED., .F., .F.,
 ( 4, 1, 1, 1, 1, 1, 1, 1, 4 ),
 ( 0.000000000000000000, 0.09809051273808343241, 0.1997563395654988194, 0.3058527769869914259, 0.4162847437678430240, 0.5377099880548563693, 0.6743560419832976827, 0.8289895874771281425, 1.000000000000000000 ),
 .UNSPECIFIED. ) ;
#8045=EDGE_CURVE ( 'NONE', #2404, #2471, #2969, .T. ) ;
#8047=CARTESIAN_POINT ( 'NONE',  ( -22.33391032228853490, 99.50000000000002842, -10.55243757774135993 ) ) ;
#8048=CARTESIAN_POINT ( 'NONE',  ( 1.653273178848927064E-15, 2.399999997815050357, -27.00000000000000355 ) ) ;
#8049=CARTESIAN_POINT ( 'NONE',  ( 9.513000527211589841, 100.0000000000000000, 20.35102222961602436 ) ) ;
#8051=CARTESIAN_POINT ( 'NONE',  ( 0.000000000000000000, 97.50000000000000000, 0.000000000000000000 ) ) ;
#8053=CARTESIAN_POINT ( 'NONE',  ( 2.837666006185522782, 99.99999999999997158, -22.03040394835428373 ) ) ;
#8055=ADVANCED_FACE ( 'NONE', ( #7620 ), #5529, .T. ) ;
#8056=CARTESIAN_POINT ( 'NONE',  ( 4.100286767325537873, 99.50000000000000000, -22.51382885696750336 ) ) ;
#8057=CARTESIAN_POINT ( 'NONE',  ( 11.18376618407356915, 2.349999997815050090, -27.00000000000000355 ) ) ;
#8058=CARTESIAN_POINT ( 'NONE',  ( -15.31787750341841559, 99.50000000000000000, 16.43551622900274722 ) ) ;
#8059=CARTESIAN_POINT ( 'NONE',  ( -21.94169572595625795, 99.50000000000000000, -9.715372641902229489 ) ) ;
#8062=CARTESIAN_POINT ( 'NONE',  ( -22.63784607493503387, 100.0000000000000142, -10.71517552924587058 ) ) ;
#8064=CARTESIAN_POINT ( 'NONE',  ( 9.583828860305853681, 99.99999999999998579, 20.68614437522342797 ) ) ;
#8066=EDGE_LOOP ( 'NONE', ( #9194, #1855, #460, #3236, #4928, #9971 ) ) ;
#8069=CARTESIAN_POINT ( 'NONE',  ( 1.679787559701184688E-15, 2.149999998907525356, -27.43301270000000258 ) ) ;
#8070=ADVANCED_FACE ( 'NONE', ( #3819 ), #4501, .T. ) ;
#8075=CARTESIAN_POINT ( 'NONE',  ( 27.00000000000000355, 4.000000000000000000, 0.000000000000000000 ) ) ;
#8076=CARTESIAN_POINT ( 'NONE',  ( -20.88772068548257366, 100.0000000000000142, -11.14739719174079546 ) ) ;
#8079=CARTESIAN_POINT ( 'NONE',  ( 0.000000000000000000, 100.0000000000000000, 0.000000000000000000 ) ) ;
#8080=ORIENTED_EDGE ( 'NONE', *, *, #2037, .F. ) ;
#8081=CIRCLE ( 'NONE', #3553, 25.15000000000000213 ) ;
#8082=CARTESIAN_POINT ( 'NONE',  ( 27.43301269999999548, 3.399999998907525356, 11.36312591709337916 ) ) ;
#8084=CARTESIAN_POINT ( 'NONE',  ( 3.293272160652527258, 99.49999999999997158, -24.41359064397622802 ) ) ;
#8085=CARTESIAN_POINT ( 'NONE',  ( -22.43115009631934953, 100.0000000000000142, -11.08196351649073819 ) ) ;
#8087=CARTESIAN_POINT ( 'NONE',  ( -19.09188309203678457, 1.699999997815050401, -19.09188309203678813 ) ) ;
#8088=CARTESIAN_POINT ( 'NONE',  ( -16.74216497804568604, 99.50000000000001421, 15.31795814478965312 ) ) ;
#8089=CARTESIAN_POINT ( 'NONE',  ( 8.063732359723156051, 100.0000000000000142, 20.72384750152746236 ) ) ;
#8090=VECTOR ( 'NONE', #1277, 1000.000000000000000 ) ;
#8092=ORIENTED_EDGE ( 'NONE', *, *, #7781, .T. ) ;
#8093=EDGE_LOOP ( 'NONE', ( #6713, #10264, #2286, #5291 ) ) ;
#8094=CARTESIAN_POINT ( 'NONE',  ( -22.33391032228853490, 99.50000000000002842, -10.55243757774135993 ) ) ;
#8096=DIRECTION ( 'NONE',  ( -0.2149789550291109352, 0.000000000000000000, -0.9766186814179788067 ) ) ;
#8098=LINE ( 'NONE', #3477, #10154 ) ;
#8100=EDGE_CURVE ( 'NONE', #5685, #4986, #4806, .T. ) ;
#8101=CARTESIAN_POINT ( 'NONE',  ( -16.25072943800822500, 99.50000000000005684, 15.30228603765648820 ) ) ;
#8102=CARTESIAN_POINT ( 'NONE',  ( -27.00000000000000355, 4.350000000000000533, -11.18376618407357270 ) ) ;
#8103=ORIENTED_EDGE ( 'NONE', *, *, #8630, .T. ) ;
#8104=ADVANCED_FACE ( 'NONE', ( #2347 ), #7308, .T. ) ;
#8105=CARTESIAN_POINT ( 'NONE',  ( 4.232447118646125439, 99.49999999999998579, -21.54138831197867887 ) ) ;
#8107=CARTESIAN_POINT ( 'NONE',  ( -21.24310748994415832, 99.99999999999998579, -10.99527971241054658 ) ) ;
#8109=CARTESIAN_POINT ( 'NONE',  ( -20.42657152723830905, 100.0000000000000000, -10.54129411626120216 ) ) ;
#8110=CARTESIAN_POINT ( 'NONE',  ( 11.36312591709336850, 4.199999998907525622, 27.43301269999999903 ) ) ;
#8112=CARTESIAN_POINT ( 'NONE',  ( 27.00000000000000355, 3.799999997815050268, 0.000000000000000000 ) ) ;
#8113=CARTESIAN_POINT ( 'NONE',  ( 3.446946945638383664, 99.99999999999997158, -21.53774374131874580 ) ) ;
#8114=DIRECTION ( 'NONE',  ( 6.944978907077980968E-14, -1.000000000000000000, -3.537534599156363020E-12 ) ) ;
#8116=EDGE_CURVE ( 'NONE', #3729, #393, #1710, .T. ) ;
#8120=CARTESIAN_POINT ( 'NONE',  ( -27.43301270000000969, 0.6999999989075252893, 11.36312591709335429 ) ) ;
#8122=EDGE_CURVE ( 'NONE', #1073, #2960, #163, .T. ) ;
#8125=CARTESIAN_POINT ( 'NONE',  ( -21.30928386698190025, 99.50000000000000000, -11.02857376369709996 ) ) ;
#8126=ADVANCED_FACE ( 'NONE', ( #2401 ), #1611, .T. ) ;
#8128=( BOUNDED_CURVE ( )  B_SPLINE_CURVE ( 2, ( #709, #1335, #6257, #1443, #8672, #7876, #2967, #3690, #552 ),
 .UNSPECIFIED., .F., .F. ) 
 B_SPLINE_CURVE_WITH_KNOTS ( ( 3, 2, 2, 2, 3 ),
 ( 0.6071428571428570953, 0.6250000000000000000, 0.6428571428571429047, 0.6607142857142856984, 0.6785714285714286031 ),
 .UNSPECIFIED. ) 
 CURVE ( )  GEOMETRIC_REPRESENTATION_ITEM ( )  RATIONAL_B_SPLINE_CURVE ( ( 1.000000000000000000, 0.9238795325112867385, 1.000000000000000000, 0.9238795325112867385, 1.000000000000000000, 0.9238795325112867385, 1.000000000000000000, 0.9238795325112867385, 1.000000000000000000 ) ) 
 REPRESENTATION_ITEM ( '' )  );
#8131=CARTESIAN_POINT ( 'NONE',  ( 3.171774962637509798, 100.0000000000000000, -24.28498992023182268 ) ) ;
#8135=CARTESIAN_POINT ( 'NONE',  ( -22.69331084068295112, 99.49999999999998579, -10.43328931840349050 ) ) ;
#8139=ORIENTED_EDGE ( 'NONE', *, *, #5765, .F. ) ;
#8140=ORIENTED_EDGE ( 'NONE', *, *, #4682, .T. ) ;
#8142=CIRCLE ( 'NONE', #1108, 27.00000000000000355 ) ;
#8143=CARTESIAN_POINT ( 'NONE',  ( -22.29247428061501779, 99.50000000000000000, -10.66603791136541624 ) ) ;
#8144=CARTESIAN_POINT ( 'NONE',  ( -18.01369080470046313, 100.0000000000000000, 17.15556831233607937 ) ) ;
#8145=CARTESIAN_POINT ( 'NONE',  ( -21.44539290152690114, 99.50000000000000000, -11.08070480119962298 ) ) ;
#8147=AXIS2_PLACEMENT_3D ( 'NONE', #2578, #7136, #8718 ) ;
#8149=EDGE_LOOP ( 'NONE', ( #454, #8362, #8183, #5238 ) ) ;
#8150=CARTESIAN_POINT ( 'NONE',  ( 8.187169943530866689, 99.49999999999998579, 20.27434297626003712 ) ) ;
#8151=CARTESIAN_POINT ( 'NONE',  ( 21.47055288461538325, 99.50000000000000000, -0.7081330128205128860 ) ) ;
#8152=CARTESIAN_POINT ( 'NONE',  ( 0.000000000000000000, 100.0000000000000000, -25.15000000000000213 ) ) ;
#8153=CARTESIAN_POINT ( 'NONE',  ( 3.375079225685456041, 100.0000000000000000, -22.79123997459842954 ) ) ;
#8154=CARTESIAN_POINT ( 'NONE',  ( 4.241330131419338123, 99.49999999999998579, -24.68798891778770965 ) ) ;
#8155=CARTESIAN_POINT ( 'NONE',  ( 4.277141017070624329, 99.50000000000002842, -21.57940364907851816 ) ) ;
#8157=CARTESIAN_POINT ( 'NONE',  ( 19.09188309203678813, 5.499999997815050001, -19.09188309203678813 ) ) ;
#8158=PLANE ( 'NONE',  #4777 ) ;
#8164=CARTESIAN_POINT ( 'NONE',  ( -15.07178375341841381, 99.99999999999998579, 16.66969090848992607 ) ) ;
#8165=CARTESIAN_POINT ( 'NONE',  ( 0.000000000000000000, 97.50000000000000000, 18.00000000000000000 ) ) ;
#8166=CARTESIAN_POINT ( 'NONE',  ( 1.653273178848927064E-15, 5.000000000000000000, -27.00000000000000355 ) ) ;
#8167=CARTESIAN_POINT ( 'NONE',  ( 21.82251602564102910, 100.0000000000000000, -0.5181290064102563875 ) ) ;
#8168=B_SPLINE_CURVE_WITH_KNOTS ( 'NONE', 3,
 ( #9921, #2755, #6529, #5794, #1853, #4222, #8938, #5947, #1130, #1806, #9138, #7506, #1958, #244, #5153, #4953, #8351, #8154, #3428 ),
 .UNSPECIFIED., .F., .F.,
 ( 4, 1, 1, 1, 1, 1, 1, 1, 1, 1, 1, 1, 1, 1, 1, 1, 4 ),
 ( 0.000000000000000000, 0.08029080299619884009, 0.1602734547033792534, 0.2412010114815648643, 0.3246404098231062685, 0.3670482715230247162, 0.4085690013065461645, 0.4496707568484641926, 0.4905395156191099670, 0.5313644394553277417, 0.5726744073239632415, 0.6138178896263115636, 0.6555018086025313773, 0.7394546411270094266, 0.8240219501092651555, 0.9101625766452680066, 1.000000000000000000 ),
 .UNSPECIFIED. ) ;
#8169=EDGE_CURVE ( 'NONE', #7890, #5137, #1238, .T. ) ;
#8171=LINE ( 'NONE', #1203, #6149 ) ;
#8172=CARTESIAN_POINT ( 'NONE',  ( -20.99557965837879081, 99.49999999999997158, -10.74478602187354959 ) ) ;
#8173=ORIENTED_EDGE ( 'NONE', *, *, #2031, .T. ) ;
#8174=CARTESIAN_POINT ( 'NONE',  ( -21.30033281797529909, 99.99999999999995737, -9.345151174687854834 ) ) ;
#8176=CARTESIAN_POINT ( 'NONE',  ( 27.43301270000000258, 0.2999999989075252671, -11.36312591709336139 ) ) ;
#8177=SURFACE_SIDE_STYLE ('',( #961 ) ) ;
#8179=CARTESIAN_POINT ( 'NONE',  ( -22.21668755910108928, 99.50000000000004263, -9.472979539922778969 ) ) ;
#8180=CARTESIAN_POINT ( 'NONE',  ( -16.79604063091391097, 100.0000000000000000, 15.40463673182947701 ) ) ;
#8181=ORIENTED_EDGE ( 'NONE', *, *, #3637, .T. ) ;
#8182=CARTESIAN_POINT ( 'NONE',  ( 5.179363668139080445, 100.0000000000000711, -23.94265746362379943 ) ) ;
#8183=ORIENTED_EDGE ( 'NONE', *, *, #3389, .T. ) ;
#8185=EDGE_LOOP ( 'NONE', ( #3112, #3968, #2605, #3032 ) ) ;
#8186=ORIENTED_EDGE ( 'NONE', *, *, #4844, .T. ) ;
#8187=CARTESIAN_POINT ( 'NONE',  ( -22.43115009631934953, 100.0000000000000142, -11.08196351649073819 ) ) ;
#8188=CARTESIAN_POINT ( 'NONE',  ( 3.202955020264580899, 99.99999999999997158, -21.91595956354277064 ) ) ;
#8189=CARTESIAN_POINT ( 'NONE',  ( -22.20893716642541804, 99.50000000000002842, -10.81429252070940272 ) ) ;
#8190=CARTESIAN_POINT ( 'NONE',  ( -15.10382517959271098, 99.99999999999998579, 15.91526905993627317 ) ) ;
#8191=EDGE_CURVE ( 'NONE', #8491, #7890, #8006, .T. ) ;
#8192=ADVANCED_FACE ( 'NONE', ( #1802 ), #7499, .F. ) ;
#8195=CARTESIAN_POINT ( 'NONE',  ( -21.93524539549613550, 99.99999999999998579, -11.03420246938663318 ) ) ;
#8196=ORIENTED_EDGE ( 'NONE', *, *, #8116, .F. ) ;
#8197=CARTESIAN_POINT ( 'NONE',  ( 3.124251205490514494, 100.0000000000000000, -23.02140944421609703 ) ) ;
#8198=CARTESIAN_POINT ( 'NONE',  ( 3.817429849879703241, 99.49999999999998579, -22.92346308580664171 ) ) ;
#8199=CARTESIAN_POINT ( 'NONE',  ( 4.049441352997683374, 99.50000000000000000, -21.43849541167161732 ) ) ;
#8200=ORIENTED_EDGE ( 'NONE', *, *, #10192, .T. ) ;
#8201=CARTESIAN_POINT ( 'NONE',  ( 3.212364564527730337, 100.0000000000000284, -22.10366694310577884 ) ) ;
#8202=CARTESIAN_POINT ( 'NONE',  ( -27.00000000000000355, 4.149999997815050357, -11.18376618407357093 ) ) ;
#8203=FACE_OUTER_BOUND ( 'NONE', #4920, .T. ) ;
#8204=CARTESIAN_POINT ( 'NONE',  ( -21.66466628782423243, 99.50000000000001421, -9.640935998098070669 ) ) ;
#8205=CARTESIAN_POINT ( 'NONE',  ( -22.27115127098604574, 99.50000000000000000, -10.71048520281369676 ) ) ;
#8206=CARTESIAN_POINT ( 'NONE',  ( 3.681717055787076642, 100.0000000000000000, -21.09125273517263111 ) ) ;
#8208=VERTEX_POINT ( 'NONE', #3334 ) ;
#8211=CARTESIAN_POINT ( 'NONE',  ( -15.03933290382598820, 99.99999999999998579, 15.19633946010233849 ) ) ;
#8212=LINE ( 'NONE', #3552, #7716 ) ;
#8213=CARTESIAN_POINT ( 'NONE',  ( 19.39806930854668110, 4.349999998907525089, -19.39806930854668110 ) ) ;
#8214=CARTESIAN_POINT ( 'NONE',  ( 1.679787559701184688E-15, 0.5499999989075251561, -27.43301270000000258 ) ) ;
#8217=CARTESIAN_POINT ( 'NONE',  ( 0.000000000000000000, 100.0000000000000000, 0.000000000000000000 ) ) ;
#8218=CARTESIAN_POINT ( 'NONE',  ( 27.00000000000000355, 2.249999997815050001, -11.18376618407356915 ) ) ;
#8219=ORIENTED_EDGE ( 'NONE', *, *, #1615, .T. ) ;
#8220=CARTESIAN_POINT ( 'NONE',  ( -21.99154324187120579, 99.50000000000001421, -9.362771248264911250 ) ) ;
#8221=CARTESIAN_POINT ( 'NONE',  ( 3.824506687597884369, 100.0000000000000284, -24.68145443631992109 ) ) ;
#8222=CARTESIAN_POINT ( 'NONE',  ( -15.76955986605724647, 99.49999999999998579, 15.18352214517458698 ) ) ;
#8224=CARTESIAN_POINT ( 'NONE',  ( 3.739209042966563867, 100.0000000000000000, -21.42288334414699236 ) ) ;
#8225=CARTESIAN_POINT ( 'NONE',  ( -16.63177974700816009, 100.0000000000000000, 16.59747536361813403 ) ) ;
#8226=CARTESIAN_POINT ( 'NONE',  ( 9.468852706215191262, 99.99999999999994316, 21.22967007823213237 ) ) ;
#8228=CARTESIAN_POINT ( 'NONE',  ( -21.91899880027261460, 100.0000000000000000, -9.705014769524845875 ) ) ;
#8229=ORIENTED_EDGE ( 'NONE', *, *, #5805, .T. ) ;
#8232=ORIENTED_EDGE ( 'NONE', *, *, #9397, .F. ) ;
#8234=CARTESIAN_POINT ( 'NONE',  ( -22.34867803760930727, 99.99999999999995737, -10.48295844864103721 ) ) ;
#8235=CARTESIAN_POINT ( 'NONE',  ( 3.673732336774000018, 99.99999999999997158, -21.43557726391590279 ) ) ;
#8236=CARTESIAN_POINT ( 'NONE',  ( 4.122675185292913547, 99.49999999999997158, -22.83451320417363561 ) ) ;
#8237=CARTESIAN_POINT ( 'NONE',  ( -15.18657300206754179, 100.0000000000000000, 16.26161032743331347 ) ) ;
#8238=CARTESIAN_POINT ( 'NONE',  ( 8.515772100368442565, 99.50000000000000000, 20.00046577258137503 ) ) ;
#8240=B_SPLINE_CURVE_WITH_KNOTS ( 'NONE', 3,
 ( #6471, #9610, #8041, #4696, #6516, #87, #8677 ),
 .UNSPECIFIED., .F., .F.,
 ( 4, 1, 1, 1, 4 ),
 ( 0.000000000000000000, 0.2676680225848128147, 0.5230972062070123885, 0.7658030722156558001, 1.000000000000000000 ),
 .UNSPECIFIED. ) ;
#8243=CARTESIAN_POINT ( 'NONE',  ( -21.33175168474226879, 100.0000000000000142, -11.03889704119913162 ) ) ;
#8244=CARTESIAN_POINT ( 'NONE',  ( 9.389534246205572643, 100.0000000000000142, 21.46805835725047729 ) ) ;
#8246=EDGE_CURVE ( 'NONE', #7350, #6241, #5426, .T. ) ;
#8247=DIRECTION ( 'NONE',  ( -0.000000000000000000, 1.000000000000000000, -0.000000000000000000 ) ) ;
#8248=CARTESIAN_POINT ( 'NONE',  ( -19.39806930854667755, 2.249999998907525001, -19.39806930854668110 ) ) ;
#8249=CARTESIAN_POINT ( 'NONE',  ( -15.32348647777738826, 99.50000000000000000, 15.39505148541300450 ) ) ;
#8251=CARTESIAN_POINT ( 'NONE',  ( 7.826802610544922878, 99.50000000000000000, 21.21129867192371421 ) ) ;
#8253=CARTESIAN_POINT ( 'NONE',  ( 3.306546357697854128E-15, 100.0000000000000000, 27.00000000000000355 ) ) ;
#8254=CARTESIAN_POINT ( 'NONE',  ( -27.00000000000000355, 4.199999997815050179, -3.306546357697854128E-15 ) ) ;
#8255=CARTESIAN_POINT ( 'NONE',  ( -20.69312081029678296, 99.49999999999997158, -9.926742041671966277 ) ) ;
#8256=CARTESIAN_POINT ( 'NONE',  ( -21.04016555629948826, 99.50000000000001421, -9.929603401003973318 ) ) ;
#8258=CARTESIAN_POINT ( 'NONE',  ( -21.58460863908062066, 100.0000000000000284, -11.10356610083683648 ) ) ;
#8259=DIRECTION ( 'NONE',  ( -0.9985036676371303876, 0.000000000000000000, 0.05468478504300072762 ) ) ;
#8264=CARTESIAN_POINT ( 'NONE',  ( -15.07178375341841381, 99.50000000000000000, 16.66969090848992607 ) ) ;
#8265=EDGE_CURVE ( 'NONE', #7818, #2647, #1847, .T. ) ;
#8266=DIRECTION ( 'NONE',  ( -0.000000000000000000, 1.000000000000000000, -0.000000000000000000 ) ) ;
#8267=CARTESIAN_POINT ( 'NONE',  ( -27.43301270000000969, 3.899999998907524912, 11.36312591709335429 ) ) ;
#8268=CARTESIAN_POINT ( 'NONE',  ( 1.653273178848927064E-15, 0.2000000000000000111, -27.00000000000000355 ) ) ;
#8269=CARTESIAN_POINT ( 'NONE',  ( -19.75840245672548789, 99.50000000000000000, -8.735905494466331689 ) ) ;
#8270=FACE_OUTER_BOUND ( 'NONE', #7661, .T. ) ;
#8273=CARTESIAN_POINT ( 'NONE',  ( 7.978247738654171251, 99.50000000000000000, 20.00924965157036794 ) ) ;
#8274=CARTESIAN_POINT ( 'NONE',  ( -19.39806930854668465, 4.749999998907525445, 19.39806930854667755 ) ) ;
#8279=CARTESIAN_POINT ( 'NONE',  ( 0.000000000000000000, 0.000000000000000000, 0.000000000000000000 ) ) ;
#8280=CARTESIAN_POINT ( 'NONE',  ( -21.38163724633288965, 100.0000000000000568, -9.681902434707239991 ) ) ;
#8281=DIRECTION ( 'NONE',  ( -0.9197984731044490658, 0.000000000000000000, 0.3923910917372159246 ) ) ;
#8283=ORIENTED_EDGE ( 'NONE', *, *, #10227, .T. ) ;
#8284=CARTESIAN_POINT ( 'NONE',  ( -22.34945848979098670, 100.0000000000000000, -10.27225542379191481 ) ) ;
#8285=CARTESIAN_POINT ( 'NONE',  ( 3.214822648120007731, 99.99999999999997158, -21.86319392453323829 ) ) ;
#8288=EDGE_CURVE ( 'NONE', #9210, #2107, #5041, .T. ) ;
#8289=DIRECTION ( 'NONE',  ( -0.000000000000000000, 1.000000000000000000, -0.000000000000000000 ) ) ;
#8290=VECTOR ( 'NONE', #10050, 1000.000000000000000 ) ;
#8291=CARTESIAN_POINT ( 'NONE',  ( 21.43339342948717885, 99.50000000000000000, -1.392427884615384803 ) ) ;
#8292=DIRECTION ( 'NONE',  ( 0.000000000000000000, 1.000000000000000000, 0.000000000000000000 ) ) ;
#8293=CARTESIAN_POINT ( 'NONE',  ( 9.838488147574068421, 100.0000000000000000, 20.25735696016189280 ) ) ;
#8294=ORIENTED_EDGE ( 'NONE', *, *, #4984, .T. ) ;
#8295=AXIS2_PLACEMENT_3D ( 'NONE', #3880, #7068, #4819 ) ;
#8296=DIRECTION ( 'NONE',  ( -0.000000000000000000, 1.000000000000000000, -0.000000000000000000 ) ) ;
#8297=CARTESIAN_POINT ( 'NONE',  ( -27.43301270000000969, 4.799999998907525267, 11.36312591709335429 ) ) ;
#8300=CARTESIAN_POINT ( 'NONE',  ( 7.783718120363267268, 99.99999999999994316, 21.09473326129887027 ) ) ;
#8301=CARTESIAN_POINT ( 'NONE',  ( 3.341734429721257005, 100.0000000000000284, -22.34498040423979148 ) ) ;
#8302=CARTESIAN_POINT ( 'NONE',  ( 26.99999999999999645, 2.949999997815051067, 11.18376618407358691 ) ) ;
#8303=FACE_OUTER_BOUND ( 'NONE', #10250, .T. ) ;
#8306=CARTESIAN_POINT ( 'NONE',  ( 4.185097728209222545, 99.50000000000000000, -21.50746221358744847 ) ) ;
#8310=ORIENTED_EDGE ( 'NONE', *, *, #8691, .T. ) ;
#8313=CARTESIAN_POINT ( 'NONE',  ( -15.29853103387017121, 99.50000000000001421, 14.98378122532347057 ) ) ;
#8315=EDGE_CURVE ( 'NONE', #1699, #9838, #3480, .T. ) ;
#8316=CARTESIAN_POINT ( 'NONE',  ( -19.39806930854667755, 2.949999998907525178, -19.39806930854668110 ) ) ;
#8317=CARTESIAN_POINT ( 'NONE',  ( -27.43301270000000258, 0.6999999989075252893, -11.36312591709336317 ) ) ;
#8318=ADVANCED_FACE ( 'NONE', ( #1123 ), #6665, .T. ) ;
#8321=DIRECTION ( 'NONE',  ( -0.000000000000000000, -1.000000000000000000, -0.000000000000000000 ) ) ;
#8323=B_SPLINE_CURVE_WITH_KNOTS ( 'NONE', 3,
 ( #7536, #8228, #1060, #5976, #4252, #6655, #7487, #326, #9168, #8280, #5187, #1109, #9846, #1884, #2681, #8385, #9897, #5920, #8661 ),
 .UNSPECIFIED., .F., .F.,
 ( 4, 1, 1, 1, 1, 1, 1, 1, 1, 1, 1, 1, 1, 1, 1, 1, 4 ),
 ( 0.000000000000000000, 0.06505403082392276215, 0.1283503816230405770, 0.1902281050068566903, 0.2509397092642763338, 0.3119571365542418429, 0.3738829716944830350, 0.4367040802691206092, 0.5009896104483916313, 0.5655726868558689224, 0.6286067690057803858, 0.6898677555008378981, 0.7506620835893632604, 0.8110632348575060879, 0.8726242918051292374, 0.9355756365154705989, 0.9999999999999998890 ),
 .UNSPECIFIED. ) ;
#8324=VERTEX_POINT ( 'NONE', #3586 ) ;
#8325=PLANE ( 'NONE',  #5120 ) ;
#8328=CARTESIAN_POINT ( 'NONE',  ( -15.98972951825121669, 99.49999999999997158, 15.19400804711857411 ) ) ;
#8329=VECTOR ( 'NONE', #1173, 1000.000000000000000 ) ;
#8332=DIRECTION ( 'NONE',  ( 0.000000000000000000, 0.000000000000000000, -1.000000000000000000 ) ) ;
#8334=DIRECTION ( 'NONE',  ( 0.000000000000000000, 1.000000000000000000, 0.000000000000000000 ) ) ;
#8336=VERTEX_POINT ( 'NONE', #7664 ) ;
#8337=CARTESIAN_POINT ( 'NONE',  ( -22.31427554260534052, 100.0000000000000000, -10.13077409178744404 ) ) ;
#8338=LINE ( 'NONE', #1168, #1616 ) ;
#8339=VECTOR ( 'NONE', #8289, 1000.000000000000000 ) ;
#8340=CARTESIAN_POINT ( 'NONE',  ( -4.959819536546781389E-15, 5.199999997815050179, 27.00000000000000355 ) ) ;
#8341=CARTESIAN_POINT ( 'NONE',  ( -15.13520964245927836, 99.99999999999998579, 15.69931698147095034 ) ) ;
#8342=CARTESIAN_POINT ( 'NONE',  ( -4.959819536546781389E-15, 3.000000000000000000, 27.00000000000000355 ) ) ;
#8343=CARTESIAN_POINT ( 'NONE',  ( 3.306546357697854128E-15, 100.0000000000000000, 27.00000000000000355 ) ) ;
#8345=CARTESIAN_POINT ( 'NONE',  ( 9.500395184910136237, 100.0000000000000000, 21.12540332933289733 ) ) ;
#8346=EDGE_LOOP ( 'NONE', ( #4203, #2096, #9372, #8405, #6481, #9312, #1100, #7537, #2738, #1359, #4012, #1190, #8080, #557, #9887, #5996 ) ) ;
#8347=DIRECTION ( 'NONE',  ( 0.000000000000000000, 1.000000000000000000, 0.000000000000000000 ) ) ;
#8348=CARTESIAN_POINT ( 'NONE',  ( 1.679787559701184688E-15, 4.549999998907526155, -27.43301270000000258 ) ) ;
#8349=DIRECTION ( 'NONE',  ( 0.000000000000000000, 1.000000000000000000, 0.000000000000000000 ) ) ;
#8351=CARTESIAN_POINT ( 'NONE',  ( 4.135809822336132591, 99.49999999999998579, -24.70305975188825443 ) ) ;
#8352=CARTESIAN_POINT ( 'NONE',  ( 19.09188309203678102, 4.499999997815050001, 19.09188309203678813 ) ) ;
#8354=CARTESIAN_POINT ( 'NONE',  ( 9.915951879163557692, 99.50000000000002842, 20.63215000232408158 ) ) ;
#8355=CARTESIAN_POINT ( 'NONE',  ( -4.959819536546781389E-15, 3.599999997815050534, 27.00000000000000355 ) ) ;
#8356=CARTESIAN_POINT ( 'NONE',  ( 11.18376618407357093, 3.350000000000000089, -27.00000000000000355 ) ) ;
#8358=CARTESIAN_POINT ( 'NONE',  ( 3.817429849879703241, 99.99999999999998579, -22.92346308580664171 ) ) ;
#8359=ORIENTED_EDGE ( 'NONE', *, *, #1008, .F. ) ;
#8362=ORIENTED_EDGE ( 'NONE', *, *, #5641, .F. ) ;
#8367=CARTESIAN_POINT ( 'NONE',  ( -14.78677372028383097, 99.49999999999998579, 15.63810349997947569 ) ) ;
#8369=CARTESIAN_POINT ( 'NONE',  ( -5.039362679103552881E-15, 2.449999998907525178, 27.43301270000000258 ) ) ;
#8370=CARTESIAN_POINT ( 'NONE',  ( -20.45905772418405988, 100.0000000000000000, -10.59533404166311321 ) ) ;
#8371=CARTESIAN_POINT ( 'NONE',  ( -15.98658610793439117, 100.0000000000000142, 14.83943845084690949 ) ) ;
#8372=PLANE ( 'NONE',  #4306 ) ;
#8373=CARTESIAN_POINT ( 'NONE',  ( 3.970307086022987431, 100.0000000000000142, -24.36314111580913178 ) ) ;
#8374=ORIENTED_EDGE ( 'NONE', *, *, #5282, .T. ) ;
#8375=CARTESIAN_POINT ( 'NONE',  ( 7.826802610544922878, 99.50000000000000000, 21.21129867192371421 ) ) ;
#8376=CARTESIAN_POINT ( 'NONE',  ( 2.912748042341355870, 99.99999999999998579, -22.34826719014139940 ) ) ;
#8380=CARTESIAN_POINT ( 'NONE',  ( -27.43301270000000258, 0.5999999989075250895, -11.36312591709336317 ) ) ;
#8382=CARTESIAN_POINT ( 'NONE',  ( 26.99999999999999645, 4.750000000000000000, 11.18376618407358691 ) ) ;
#8384=CARTESIAN_POINT ( 'NONE',  ( 9.513000527211589841, 99.99999999999994316, 20.35102222961602436 ) ) ;
#8385=CARTESIAN_POINT ( 'NONE',  ( -21.04016555629948826, 100.0000000000000142, -9.929603401003973318 ) ) ;
#8387=CARTESIAN_POINT ( 'NONE',  ( -15.83671465916681242, 100.0000000000000000, 16.65403364262263608 ) ) ;
#8389=ORIENTED_EDGE ( 'NONE', *, *, #6951, .F. ) ;
#8390=VECTOR ( 'NONE', #8519, 1000.000000000000000 ) ;
#8391=CARTESIAN_POINT ( 'NONE',  ( 4.693123912524271191, 99.50000000000002842, -24.12247278045041554 ) ) ;
#8392=CARTESIAN_POINT ( 'NONE',  ( 27.43301269999999548, 0.9999999989075253337, 11.36312591709337916 ) ) ;
#8393=CARTESIAN_POINT ( 'NONE',  ( -4.959819536546781389E-15, 0.6000000000000000888, 27.00000000000000355 ) ) ;
#8394=CARTESIAN_POINT ( 'NONE',  ( -15.31787750341841559, 100.0000000000000000, 16.43551622900274722 ) ) ;
#8396=CARTESIAN_POINT ( 'NONE',  ( -16.67860655220511035, 99.99999999999998579, 15.23428378554110374 ) ) ;
#8397=CARTESIAN_POINT ( 'NONE',  ( -15.09818093130665773, 99.50000000000000000, 16.69478731934044191 ) ) ;
#8398=VECTOR ( 'NONE', #6439, 1000.000000000000227 ) ;
#8399=ORIENTED_EDGE ( 'NONE', *, *, #2242, .T. ) ;
#8400=DIRECTION ( 'NONE',  ( 0.9766186814179788067, 0.000000000000000000, -0.2149789550291109352 ) ) ;
#8402=CARTESIAN_POINT ( 'NONE',  ( -5.039362679103552881E-15, 4.149999998907524912, 27.43301270000000258 ) ) ;
#8405=ORIENTED_EDGE ( 'NONE', *, *, #967, .F. ) ;
#8407=CARTESIAN_POINT ( 'NONE',  ( 5.179363668139080445, 99.50000000000007105, -23.94265746362379943 ) ) ;
#8410=DIRECTION ( 'NONE',  ( 0.000000000000000000, 1.000000000000000000, 0.000000000000000000 ) ) ;
#8411=EDGE_CURVE ( 'NONE', #7177, #9070, #9017, .T. ) ;
#8413=CARTESIAN_POINT ( 'NONE',  ( -16.12578516900833137, 99.50000000000001421, 15.23469143358620492 ) ) ;
#8414=CARTESIAN_POINT ( 'NONE',  ( 11.36312591709336139, 2.099999998907525089, -27.43301270000000258 ) ) ;
#8415=ORIENTED_EDGE ( 'NONE', *, *, #531, .T. ) ;
#8420=CARTESIAN_POINT ( 'NONE',  ( -5.039362679103552881E-15, 1.649999998907525356, 27.43301270000000258 ) ) ;
#8421=CARTESIAN_POINT ( 'NONE',  ( 7.156925775808251622, 99.50000000000000000, 23.91622092442889524 ) ) ;
#8422=EDGE_LOOP ( 'NONE', ( #5747, #2822, #648, #2019 ) ) ;
#8423=CARTESIAN_POINT ( 'NONE',  ( -15.07178375341841559, 100.0000000000000142, 15.16157792772069968 ) ) ;
#8426=EDGE_CURVE ( 'NONE', #2804, #1454, #6586, .T. ) ;
#8427=EDGE_CURVE ( 'NONE', #5650, #6302, #2014, .T. ) ;
#8428=CARTESIAN_POINT ( 'NONE',  ( 4.232798786556307036, 100.0000000000000000, -24.34936571594186105 ) ) ;
#8431=ORIENTED_EDGE ( 'NONE', *, *, #237, .T. ) ;
#8433=CARTESIAN_POINT ( 'NONE',  ( 19.39806930854668110, 1.949999998907525178, -19.39806930854668110 ) ) ;
#8434=ORIENTED_EDGE ( 'NONE', *, *, #1792, .F. ) ;
#8436=CARTESIAN_POINT ( 'NONE',  ( 7.156925775808251622, 99.50000000000000000, 23.91622092442889524 ) ) ;
#8437=CARTESIAN_POINT ( 'NONE',  ( 1.653273178848927064E-15, 2.600000000000000533, -27.00000000000000355 ) ) ;
#8439=VECTOR ( 'NONE', #1081, 1000.000000000000000 ) ;
#8440=CARTESIAN_POINT ( 'NONE',  ( 4.803433990161294354, 100.0000000000000142, -23.96838578116891583 ) ) ;
#8443=CARTESIAN_POINT ( 'NONE',  ( -22.21584973381871464, 99.50000000000001421, -9.938501092090024969 ) ) ;
#8445=CARTESIAN_POINT ( 'NONE',  ( -21.31369174262763622, 99.49999999999997158, -9.710155485040722567 ) ) ;
#8448=CARTESIAN_POINT ( 'NONE',  ( 3.302864939465488536, 100.0000000000000142, -22.83905924565489443 ) ) ;
#8449=ORIENTED_EDGE ( 'NONE', *, *, #8746, .T. ) ;
#8450=EDGE_CURVE ( 'NONE', #8484, #3366, #7552, .T. ) ;
#8451=CARTESIAN_POINT ( 'NONE',  ( 3.306546357697854128E-15, 100.0000000000000000, 27.00000000000000355 ) ) ;
#8452=CARTESIAN_POINT ( 'NONE',  ( -11.18376618407356737, 1.050000000000000044, -27.00000000000000355 ) ) ;
#8453=CARTESIAN_POINT ( 'NONE',  ( 9.513000527211589841, 100.0000000000000000, 20.35102222961602436 ) ) ;
#8454=( BOUNDED_CURVE ( )  B_SPLINE_CURVE ( 2, ( #6557, #818, #2540, #9748, #4789, #7244, #7986, #5733, #7196 ),
 .UNSPECIFIED., .F., .T. ) 
 B_SPLINE_CURVE_WITH_KNOTS ( ( 3, 2, 2, 2, 3 ),
 ( 0.8214285714285713969, 0.8392857142857143016, 0.8571428571428570953, 0.8750000000000000000, 0.8928571428571429047 ),
 .UNSPECIFIED. ) 
 CURVE ( )  GEOMETRIC_REPRESENTATION_ITEM ( )  RATIONAL_B_SPLINE_CURVE ( ( 1.000000000000000000, 0.9238795325112867385, 1.000000000000000000, 0.9238795325112867385, 1.000000000000000000, 0.9238795325112867385, 1.000000000000000000, 0.9238795325112867385, 1.000000000000000000 ) ) 
 REPRESENTATION_ITEM ( '' )  );
#8455=ORIENTED_EDGE ( 'NONE', *, *, #2793, .T. ) ;
#8457=CARTESIAN_POINT ( 'NONE',  ( -27.43301270000000258, 4.749999998907525445, -3.359575119402369376E-15 ) ) ;
#8459=DIRECTION ( 'NONE',  ( 0.9789429660840186509, 0.000000000000000000, -0.2041339490496966447 ) ) ;
#8461=FACE_OUTER_BOUND ( 'NONE', #10194, .T. ) ;
#8463=DIRECTION ( 'NONE',  ( 0.000000000000000000, 0.000000000000000000, 1.000000000000000000 ) ) ;
#8465=CARTESIAN_POINT ( 'NONE',  ( -16.45391695211397831, 99.50000000000004263, 16.32580124622701589 ) ) ;
#8468=CARTESIAN_POINT ( 'NONE',  ( -15.62751930918662069, 99.49999999999998579, 15.20915780906945436 ) ) ;
#8469=CARTESIAN_POINT ( 'NONE',  ( 27.43301270000000258, 1.199999998907525178, -11.36312591709336139 ) ) ;
#8470=ORIENTED_EDGE ( 'NONE', *, *, #1973, .F. ) ;
#8474=CARTESIAN_POINT ( 'NONE',  ( 8.684839681857363658, 99.50000000000001421, 19.94043386883836178 ) ) ;
#8477=CARTESIAN_POINT ( 'NONE',  ( 4.852629679480013891, 99.50000000000001421, -23.84752007312514621 ) ) ;
#8478=CARTESIAN_POINT ( 'NONE',  ( -27.43301270000000969, 0.7999999989075252671, 11.36312591709335429 ) ) ;
#8479=CARTESIAN_POINT ( 'NONE',  ( -15.37123125604856710, 100.0000000000000142, 16.48683530611566539 ) ) ;
#8482=CARTESIAN_POINT ( 'NONE',  ( 7.771508748547515388, 100.0000000000000142, 20.40818475981234315 ) ) ;
#8483=CARTESIAN_POINT ( 'NONE',  ( -15.62751930918662069, 99.99999999999998579, 15.20915780906945436 ) ) ;
#8484=VERTEX_POINT ( 'NONE', #7199 ) ;
#8488=CARTESIAN_POINT ( 'NONE',  ( 27.00000000000000355, 0.5999999978150503122, 0.000000000000000000 ) ) ;
#8489=CARTESIAN_POINT ( 'NONE',  ( -27.43301270000000258, 2.999999998907525445, -11.36312591709336317 ) ) ;
#8491=VERTEX_POINT ( 'NONE', #86 ) ;
#8493=CARTESIAN_POINT ( 'NONE',  ( 11.18376618407357626, 1.450000000000000400, 27.00000000000000000 ) ) ;
#8495=LINE ( 'NONE', #1431, #1604 ) ;
#8496=ORIENTED_EDGE ( 'NONE', *, *, #4844, .F. ) ;
#8499=ORIENTED_EDGE ( 'NONE', *, *, #7813, .F. ) ;
#8502=CARTESIAN_POINT ( 'NONE',  ( 27.43301270000000258, 0.2999999989075252671, -11.36312591709336139 ) ) ;
#8505=CARTESIAN_POINT ( 'NONE',  ( 5.242860087038358152, 99.50000000000002842, -23.52699316036146371 ) ) ;
#8506=CARTESIAN_POINT ( 'NONE',  ( 4.820889542125314620, 99.49999999999998579, -21.76289454767624676 ) ) ;
#8509=EDGE_LOOP ( 'NONE', ( #4823, #6196 ) ) ;
#8511=CARTESIAN_POINT ( 'NONE',  ( -22.10910773081910818, 99.50000000000001421, -11.33820747227609793 ) ) ;
#8514=ADVANCED_FACE ( 'NONE', ( #823 ), #583, .T. ) ;
#8515=CARTESIAN_POINT ( 'NONE',  ( 9.897596448871711416, 99.99999999999997158, 20.85734708541456328 ) ) ;
#8516=B_SPLINE_SURFACE_WITH_KNOTS ( 'NONE', 3, 1, ( 
 ( #150, #2557 ),
 ( #4028, #8153 ),
 ( #195, #2455 ),
 ( #6431, #3378 ),
 ( #9761, #8197 ),
 ( #1668, #7400 ),
 ( #242, #2648 ) ),
 .UNSPECIFIED., .F., .F., .F.,
 ( 4, 1, 1, 1, 4 ),
 ( 2, 2 ),
 ( 0.000000000000000000, 0.2581490702850675056, 0.5078756004687992043, 0.7540928115589713432, 1.000000000000000000 ),
 ( 0.000000000000000000, 1.000000000000000000 ),
 .UNSPECIFIED. ) ;
#8519=DIRECTION ( 'NONE',  ( -0.000000000000000000, 1.000000000000000000, -0.000000000000000000 ) ) ;
#8524=B_SPLINE_CURVE_WITH_KNOTS ( 'NONE', 3,
 ( #1993, #9220, #8391, #1222, #2108, #4413, #7597, #10123, #2052, #2962, #7655 ),
 .UNSPECIFIED., .F., .F.,
 ( 4, 1, 1, 1, 1, 1, 1, 1, 4 ),
 ( 0.000000000000000000, 0.1199228846740813259, 0.2396820999030742083, 0.3587608595380448184, 0.4799620281296770319, 0.6043577515038436321, 0.7314057062717854718, 0.8632643124108332344, 1.000000000000000000 ),
 .UNSPECIFIED. ) ;
#8525=CARTESIAN_POINT ( 'NONE',  ( -16.05932294508833280, 99.50000000000000000, 15.21084698918278555 ) ) ;
#8526=CARTESIAN_POINT ( 'NONE',  ( -11.36312591709335962, 2.999999998907525445, -27.43301270000000258 ) ) ;
#8529=CARTESIAN_POINT ( 'NONE',  ( -22.67573144110267336, 99.50000000000001421, -10.14737752305977381 ) ) ;
#8530=CYLINDRICAL_SURFACE ( 'NONE', #2929, 27.00000000000000355 ) ;
#8532=CARTESIAN_POINT ( 'NONE',  ( 4.871887406949175769, 99.49999999999995737, -23.77896509604281405 ) ) ;
#8533=CARTESIAN_POINT ( 'NONE',  ( 19.39806930854667399, 1.849999998907525312, 19.39806930854668465 ) ) ;
#8535=CARTESIAN_POINT ( 'NONE',  ( -15.69015368034045643, 100.0000000000000142, 16.64011368054243434 ) ) ;
#8537=CARTESIAN_POINT ( 'NONE',  ( 2.847408871211157155, 99.50000000000001421, -22.10537533382872510 ) ) ;
#8538=DIRECTION ( 'NONE',  ( 0.000000000000000000, 0.000000000000000000, 1.000000000000000000 ) ) ;
#8540=ORIENTED_EDGE ( 'NONE', *, *, #2242, .F. ) ;
#8542=CARTESIAN_POINT ( 'NONE',  ( -21.20999280589743918, 99.50000000000002842, -11.35389291771566000 ) ) ;
#8544=DIRECTION ( 'NONE',  ( 0.000000000000000000, 0.000000000000000000, 1.000000000000000000 ) ) ;
#8545=CARTESIAN_POINT ( 'NONE',  ( -27.43301270000000258, 3.799999998907525711, -11.36312591709336317 ) ) ;
#8549=CARTESIAN_POINT ( 'NONE',  ( 27.00000000000000355, 1.600000000000000089, 0.000000000000000000 ) ) ;
#8550=CARTESIAN_POINT ( 'NONE',  ( 8.684839681857363658, 99.50000000000001421, 19.94043386883836178 ) ) ;
#8551=VERTEX_POINT ( 'NONE', #3182 ) ;
#8552=CARTESIAN_POINT ( 'NONE',  ( -16.56356094049941419, 99.49999999999997158, 15.77213757552179629 ) ) ;
#8553=CARTESIAN_POINT ( 'NONE',  ( 8.132491713109027742, 99.50000000000001421, 21.08089001807756446 ) ) ;
#8556=ORIENTED_EDGE ( 'NONE', *, *, #8315, .F. ) ;
#8558=EDGE_CURVE ( 'NONE', #8551, #9293, #6368, .T. ) ;
#8562=CARTESIAN_POINT ( 'NONE',  ( 4.922541232168287983, 100.0000000000000568, -24.37252920941159928 ) ) ;
#8564=CARTESIAN_POINT ( 'NONE',  ( 4.358720771404392735, 99.50000000000000000, -21.20742720589606378 ) ) ;
#8567=CARTESIAN_POINT ( 'NONE',  ( 3.411785164761435674, 99.50000000000000000, -22.76693382491622231 ) ) ;
#8568=CARTESIAN_POINT ( 'NONE',  ( 27.00000000000000355, 0.8000000000000000444, 0.000000000000000000 ) ) ;
#8571=LINE ( 'NONE', #3033, #4539 ) ;
#8573=VECTOR ( 'NONE', #3427, 1000.000000000000227 ) ;
#8575=CARTESIAN_POINT ( 'NONE',  ( -22.05573893622344173, 100.0000000000000000, -9.391591294897233766 ) ) ;
#8576=CARTESIAN_POINT ( 'NONE',  ( 4.772556553149396308, 99.49999999999997158, -24.49721679606612312 ) ) ;
#8577=EDGE_CURVE ( 'NONE', #519, #776, #1024, .T. ) ;
#8579=CARTESIAN_POINT ( 'NONE',  ( -16.57330815294036697, 99.50000000000001421, 15.84440382193293217 ) ) ;
#8580=VECTOR ( 'NONE', #419, 1000.000000000000114 ) ;
#8581=VERTEX_POINT ( 'NONE', #1839 ) ;
#8582=EDGE_CURVE ( 'NONE', #7789, #8960, #2544, .T. ) ;
#8583=CARTESIAN_POINT ( 'NONE',  ( 24.91446314102564230, 100.0000000000000000, -1.581029647435897578 ) ) ;
#8584=( GEOMETRIC_REPRESENTATION_CONTEXT ( 3 ) GLOBAL_UNCERTAINTY_ASSIGNED_CONTEXT ( ( #10098 ) ) GLOBAL_UNIT_ASSIGNED_CONTEXT ( ( #1933, #1104, #374 ) ) REPRESENTATION_CONTEXT ( 'NONE', 'WORKASPACE' ) );
#8585=CARTESIAN_POINT ( 'NONE',  ( 27.43301270000000258, 1.949999998907525178, 0.000000000000000000 ) ) ;
#8586=ORIENTED_EDGE ( 'NONE', *, *, #699, .F. ) ;
#8589=CARTESIAN_POINT ( 'NONE',  ( -22.08823018108446234, 100.0000000000000000, -9.406177930363766038 ) ) ;
#8591=CARTESIAN_POINT ( 'NONE',  ( -20.93575003794465061, 99.50000000000001421, -10.12220034237898503 ) ) ;
#8592=CARTESIAN_POINT ( 'NONE',  ( -11.36312591709335962, 1.399999998907525578, -27.43301270000000258 ) ) ;
#8593=ORIENTED_EDGE ( 'NONE', *, *, #3187, .T. ) ;
#8594=ORIENTED_EDGE ( 'NONE', *, *, #2386, .T. ) ;
#8595=CARTESIAN_POINT ( 'NONE',  ( -15.56505537928961047, 100.0000000000000284, 14.87309967080592088 ) ) ;
#8597=CARTESIAN_POINT ( 'NONE',  ( 3.207057600658871355, 99.50000000000000000, -22.07913334414698880 ) ) ;
#8599=CARTESIAN_POINT ( 'NONE',  ( -15.32348647777738826, 100.0000000000000000, 15.39505148541300450 ) ) ;
#8600=EDGE_LOOP ( 'NONE', ( #7792, #3904, #7868, #3572 ) ) ;
#8602=CARTESIAN_POINT ( 'NONE',  ( 4.743081672682207817, 99.50000000000002842, -21.60795120912350598 ) ) ;
#8605=CARTESIAN_POINT ( 'NONE',  ( 1.679787559701184688E-15, 2.849999998907525534, -27.43301270000000258 ) ) ;
#8606=ORIENTED_EDGE ( 'NONE', *, *, #7579, .F. ) ;
#8607=CARTESIAN_POINT ( 'NONE',  ( 4.486604876299897349, 99.50000000000000000, -21.85617661337775885 ) ) ;
#8608=DIRECTION ( 'NONE',  ( -0.000000000000000000, 1.000000000000000000, -0.000000000000000000 ) ) ;
#8610=CARTESIAN_POINT ( 'NONE',  ( -15.19031985176477662, 99.49999999999998579, 15.56880617076518547 ) ) ;
#8611=CARTESIAN_POINT ( 'NONE',  ( 8.091962505948220752, 99.49999999999995737, 20.48385654212622242 ) ) ;
#8614=EDGE_LOOP ( 'NONE', ( #4150, #10285, #5269, #1001 ) ) ;
#8615=DIRECTION ( 'NONE',  ( 0.000000000000000000, -0.000000000000000000, 1.000000000000000000 ) ) ;
#8616=CARTESIAN_POINT ( 'NONE',  ( -21.73488407773357167, 99.50000000000000000, -9.647150398373231184 ) ) ;
#8617=B_SPLINE_SURFACE_WITH_KNOTS ( 'NONE', 3, 1, ( 
 ( #6714, #9501 ),
 ( #9965, #1378 ),
 ( #7029, #6246 ),
 ( #5420, #9333 ),
 ( #7766, #6137 ),
 ( #3014, #4363 ),
 ( #7081, #337 ),
 ( #8552, #3894 ),
 ( #5363, #3792 ),
 ( #4627, #6977 ),
 ( #2325, #649 ),
 ( #7869, #10286 ),
 ( #3120, #10178 ),
 ( #2744, #4313 ),
 ( #2276, #5936 ),
 ( #5472, #8663 ),
 ( #1486, #5674 ),
 ( #7973, #9592 ),
 ( #907, #4926 ) ),
 .UNSPECIFIED., .F., .F., .F.,
 ( 4, 1, 1, 1, 1, 1, 1, 1, 1, 1, 1, 1, 1, 1, 1, 1, 4 ),
 ( 2, 2 ),
 ( 0.000000000000000000, 0.06442465027149940626, 0.1272622498775801414, 0.1890519169419207224, 0.2498421757728049863, 0.3110425729590077792, 0.3720985300252119266, 0.4351465435385043490, 0.5001170788027262670, 0.5644817420234762295, 0.6276143074669133792, 0.6889588046791949028, 0.7501592018653976401, 0.8106582772613761811, 0.8724479443257179279, 0.9351683423010851426, 1.000000000000000000 ),
 ( 0.000000000000000000, 1.000000000000000000 ),
 .UNSPECIFIED. ) ;
#8619=CARTESIAN_POINT ( 'NONE',  ( 3.124251205490514494, 100.0000000000000000, -23.02140944421609703 ) ) ;
#8625=CARTESIAN_POINT ( 'NONE',  ( 3.080354370726382296, 99.50000000000004263, -23.09295995363041598 ) ) ;
#8626=CARTESIAN_POINT ( 'NONE',  ( 9.575551604960836016, 100.0000000000000142, 20.57049984249936969 ) ) ;
#8628=CARTESIAN_POINT ( 'NONE',  ( 4.486604876299897349, 100.0000000000000000, -21.85617661337775885 ) ) ;
#8630=EDGE_CURVE ( 'NONE', #6174, #9675, #1667, .T. ) ;
#8631=EDGE_LOOP ( 'NONE', ( #7247, #137, #5483, #70 ) ) ;
#8632=CARTESIAN_POINT ( 'NONE',  ( 1.662111305799679408E-15, 5.516666664845875090, -27.14433756666667108 ) ) ;
#8633=CARTESIAN_POINT ( 'NONE',  ( 4.922541232168287983, 99.50000000000002842, -24.37252920941159928 ) ) ;
#8638=CARTESIAN_POINT ( 'NONE',  ( -15.91768310440539658, 100.0000000000000284, 15.18344740530786652 ) ) ;
#8639=CARTESIAN_POINT ( 'NONE',  ( -27.43301270000000969, 1.599999998907525756, 11.36312591709335784 ) ) ;
#8640=VERTEX_POINT ( 'NONE', #9904 ) ;
#8642=DIRECTION ( 'NONE',  ( 0.2907756355032780071, 0.000000000000000000, 0.9567912676219745283 ) ) ;
#8644=CARTESIAN_POINT ( 'NONE',  ( -16.63177974700816009, 99.50000000000000000, 16.59747536361813403 ) ) ;
#8645=CARTESIAN_POINT ( 'NONE',  ( -5.039362679103552881E-15, 3.349999998907525534, 27.43301270000000258 ) ) ;
#8647=CARTESIAN_POINT ( 'NONE',  ( -15.27171031718473770, 100.0000000000000000, 15.44886715306589764 ) ) ;
#8648=CARTESIAN_POINT ( 'NONE',  ( 3.888553205800344248, 99.49999999999995737, -24.35333287445124739 ) ) ;
#8649=CARTESIAN_POINT ( 'NONE',  ( 3.317038232150706367, 99.49999999999998579, -21.66195598387956878 ) ) ;
#8650=CARTESIAN_POINT ( 'NONE',  ( -19.46743691185369585, 99.50000000000000000, -8.912588186774021537 ) ) ;
#8651=VECTOR ( 'NONE', #9174, 1000.000000000000227 ) ;
#8653=CARTESIAN_POINT ( 'NONE',  ( 4.200543313440712190, 99.50000000000000000, -21.13206004899810608 ) ) ;
#8654=VERTEX_POINT ( 'NONE', #2739 ) ;
#8656=CARTESIAN_POINT ( 'NONE',  ( 27.43301269999999548, 3.399999998907525356, 11.36312591709337738 ) ) ;
#8659=EDGE_CURVE ( 'NONE', #1908, #8324, #9966, .T. ) ;
#8660=CARTESIAN_POINT ( 'NONE',  ( -27.00000000000001421, 1.250000000000000222, 11.18376618407356382 ) ) ;
#8661=CARTESIAN_POINT ( 'NONE',  ( -20.96643530928959365, 99.99999999999997158, -10.05541671241504886 ) ) ;
#8662=ORIENTED_EDGE ( 'NONE', *, *, #4290, .F. ) ;
#8663=CARTESIAN_POINT ( 'NONE',  ( -16.45391695211397831, 100.0000000000000000, 16.32580124622701589 ) ) ;
#8664=CARTESIAN_POINT ( 'NONE',  ( 8.281567445270807681, 99.50000000000000000, 20.15885744430370252 ) ) ;
#8667=ORIENTED_EDGE ( 'NONE', *, *, #6377, .F. ) ;
#8669=CARTESIAN_POINT ( 'NONE',  ( -27.43301270000000969, 3.899999998907525356, 11.36312591709335784 ) ) ;
#8670=FACE_OUTER_BOUND ( 'NONE', #6446, .T. ) ;
#8672=CARTESIAN_POINT ( 'NONE',  ( -27.00000000000000355, 3.600000000000000533, -3.306546357697854128E-15 ) ) ;
#8673=CARTESIAN_POINT ( 'NONE',  ( 27.00000000000000355, 4.599999997815050534, 0.000000000000000000 ) ) ;
#8674=AXIS2_PLACEMENT_3D ( 'NONE', #6689, #9004, #5068 ) ;
#8677=CARTESIAN_POINT ( 'NONE',  ( -20.72805389903318130, 99.50000000000000000, -9.848585782927868237 ) ) ;
#8678=ORIENTED_EDGE ( 'NONE', *, *, #6951, .T. ) ;
#8682=CARTESIAN_POINT ( 'NONE',  ( 2.958578797724396026, 99.50000000000000000, -23.36432507653281121 ) ) ;
#8683=CARTESIAN_POINT ( 'NONE',  ( 9.778118981323553172, 99.99999999999998579, 20.11889122584574352 ) ) ;
#8684=( BOUNDED_CURVE ( )  B_SPLINE_CURVE ( 2, ( #1723, #2358, #5555, #6287, #8112, #4083, #8748, #942, #5659 ),
 .UNSPECIFIED., .F., .F. ) 
 B_SPLINE_CURVE_WITH_KNOTS ( ( 3, 2, 2, 2, 3 ),
 ( 0.5357142857142856984, 0.5535714285714286031, 0.5714285714285713969, 0.5892857142857143016, 0.6071428571428570953 ),
 .UNSPECIFIED. ) 
 CURVE ( )  GEOMETRIC_REPRESENTATION_ITEM ( )  RATIONAL_B_SPLINE_CURVE ( ( 1.000000000000000000, 0.9238795325112867385, 1.000000000000000000, 0.9238795325112867385, 1.000000000000000000, 0.9238795325112867385, 1.000000000000000000, 0.9238795325112867385, 1.000000000000000000 ) ) 
 REPRESENTATION_ITEM ( '' )  );
#8686=CARTESIAN_POINT ( 'NONE',  ( -16.36254897777739004, 99.50000000000001421, 15.39785597259249350 ) ) ;
#8688=CARTESIAN_POINT ( 'NONE',  ( 1.653273178848927064E-15, 3.199999997815050623, -27.00000000000000355 ) ) ;
#8689=CARTESIAN_POINT ( 'NONE',  ( -27.43301270000000258, 4.749999998907525445, -3.359575119402369376E-15 ) ) ;
#8690=ORIENTED_EDGE ( 'NONE', *, *, #2685, .F. ) ;
#8691=EDGE_CURVE ( 'NONE', #9173, #8491, #231, .T. ) ;
#8694=CARTESIAN_POINT ( 'NONE',  ( 3.291601991079349698, 99.99999999999997158, -22.28586332678438353 ) ) ;
#8696=CARTESIAN_POINT ( 'NONE',  ( -16.67860655220511035, 99.49999999999998579, 15.23428378554110374 ) ) ;
#8697=CARTESIAN_POINT ( 'NONE',  ( 27.00000000000000355, 1.399999997815050579, 0.000000000000000000 ) ) ;
#8698=CARTESIAN_POINT ( 'NONE',  ( 4.486604876299897349, 100.0000000000000000, -21.85617661337775885 ) ) ;
#8700=CARTESIAN_POINT ( 'NONE',  ( 3.204253864046738176, 99.50000000000000000, -22.06071064728738662 ) ) ;
#8701=B_SPLINE_SURFACE_WITH_KNOTS ( 'NONE', 3, 1, ( 
 ( #8058, #1519 ),
 ( #5605, #684 ),
 ( #842, #739 ),
 ( #4665, #4034 ),
 ( #3297, #6385 ),
 ( #892, #5554 ),
 ( #4082, #7170 ),
 ( #6487, #7215 ),
 ( #8747, #7854 ),
 ( #51, #2256 ),
 ( #3156, #7264 ),
 ( #4761, #9578 ),
 ( #2462, #4713 ),
 ( #2126, #2357 ),
 ( #106, #6286 ),
 ( #5458, #2410 ),
 ( #7064, #8647 ),
 ( #5509, #10271 ),
 ( #1674, #3876 ) ),
 .UNSPECIFIED., .F., .F., .F.,
 ( 4, 1, 1, 1, 1, 1, 1, 1, 1, 1, 1, 1, 1, 1, 1, 1, 4 ),
 ( 2, 2 ),
 ( 0.000000000000000000, 0.06473908249738200005, 0.1274869542813800993, 0.1888754624962200035, 0.2498352098569301405, 0.3101749858420705941, 0.3718734486855839183, 0.4342313324889700565, 0.4990836447755341299, 0.5639614065304963120, 0.6264045329497629488, 0.6882484937299673255, 0.7493615009078817835, 0.8100377551054726011, 0.8717391907241844873, 0.9348513958286107650, 1.000000000000000000 ),
 ( 0.000000000000000000, 1.000000000000000000 ),
 .UNSPECIFIED. ) ;
#8702=PLANE ( 'NONE',  #8295 ) ;
#8704=CARTESIAN_POINT ( 'NONE',  ( -20.72805389903318130, 99.50000000000000000, -9.848585782927868237 ) ) ;
#8705=ORIENTED_EDGE ( 'NONE', *, *, #5584, .F. ) ;
#8706=ADVANCED_FACE ( 'NONE', ( #4162 ), #495, .T. ) ;
#8707=EDGE_LOOP ( 'NONE', ( #8499, #9934, #4205, #3967, #1965, #3633 ) ) ;
#8709=CARTESIAN_POINT ( 'NONE',  ( 1.679787559701184688E-15, 0.5499999989075251561, -27.43301270000000258 ) ) ;
#8710=CARTESIAN_POINT ( 'NONE',  ( -15.09818093130665773, 99.50000000000000000, 16.69478731934044191 ) ) ;
#8711=CARTESIAN_POINT ( 'NONE',  ( 19.09188309203678813, 0.1000000000000000056, -19.09188309203678813 ) ) ;
#8715=CARTESIAN_POINT ( 'NONE',  ( -15.42956291708403782, 99.99999999999998579, 16.53061251458192515 ) ) ;
#8716=EDGE_CURVE ( 'NONE', #6863, #2532, #7544, .T. ) ;
#8718=DIRECTION ( 'NONE',  ( -0.9197984731044490658, 0.000000000000000000, 0.3923910917372159246 ) ) ;
#8720=CARTESIAN_POINT ( 'NONE',  ( 11.36312591709336139, 1.999999998907525445, -27.43301270000000258 ) ) ;
#8721=CARTESIAN_POINT ( 'NONE',  ( 3.824506687597884369, 100.0000000000000284, -24.68145443631992109 ) ) ;
#8723=LINE ( 'NONE', #10347, #1201 ) ;
#8724=FACE_OUTER_BOUND ( 'NONE', #7389, .T. ) ;
#8725=CARTESIAN_POINT ( 'NONE',  ( 4.446585460023182890, 99.50000000000002842, -21.79057454014859019 ) ) ;
#8726=EDGE_LOOP ( 'NONE', ( #1526, #278, #4100, #5789, #1023, #4459, #2879, #6251, #5437, #7650, #1803, #1791, #3921, #6293, #180, #7101, #8140 ) ) ;
#8728=ORIENTED_EDGE ( 'NONE', *, *, #2179, .T. ) ;
#8731=CARTESIAN_POINT ( 'NONE',  ( 8.857094148306096315, 99.50000000000001421, 19.57755665027156766 ) ) ;
#8734=CARTESIAN_POINT ( 'NONE',  ( -22.28244091826395135, 100.0000000000000000, -10.68852969318427881 ) ) ;
#8736=CARTESIAN_POINT ( 'NONE',  ( -22.28244091826395135, 99.50000000000000000, -10.68852969318427881 ) ) ;
#8737=CARTESIAN_POINT ( 'NONE',  ( -14.83571502646304197, 99.50000000000004263, 16.32397075880403392 ) ) ;
#8738=CARTESIAN_POINT ( 'NONE',  ( 19.39806930854668110, 4.449999998907525622, -19.39806930854668110 ) ) ;
#8739=VECTOR ( 'NONE', #4050, 1000.000000000000000 ) ;
#8740=EDGE_LOOP ( 'NONE', ( #1316, #4531, #3068, #2995 ) ) ;
#8742=CARTESIAN_POINT ( 'NONE',  ( 3.986298408513477387, 100.0000000000000284, -22.53092616755505162 ) ) ;
#8744=CARTESIAN_POINT ( 'NONE',  ( -20.45905772418405988, 99.50000000000000000, -10.59533404166311321 ) ) ;
#8745=CARTESIAN_POINT ( 'NONE',  ( 19.39806930854667399, 4.249999998907525445, 19.39806930854668465 ) ) ;
#8746=EDGE_CURVE ( 'NONE', #2748, #9210, #8524, .T. ) ;
#8747=CARTESIAN_POINT ( 'NONE',  ( -15.10617644529808423, 99.50000000000002842, 15.98944417891004477 ) ) ;
#8748=CARTESIAN_POINT ( 'NONE',  ( 19.09188309203678813, 3.899999997815050357, -19.09188309203678813 ) ) ;
#8749=CARTESIAN_POINT ( 'NONE',  ( 3.207057600658871355, 100.0000000000000000, -22.07913334414698880 ) ) ;
#8752=LINE ( 'NONE', #3835, #6469 ) ;
#8754=CARTESIAN_POINT ( 'NONE',  ( 19.39806930854667399, 1.049999998907525045, 19.39806930854668465 ) ) ;
#8755=CARTESIAN_POINT ( 'NONE',  ( -15.15193744131588183, 99.50000000000001421, 16.74589488344418697 ) ) ;
#8757=CARTESIAN_POINT ( 'NONE',  ( -11.18376618407356560, 4.250000000000000888, -27.00000000000000355 ) ) ;
#8759=ADVANCED_FACE ( 'NONE', ( #435 ), #1329, .F. ) ;
#8761=CARTESIAN_POINT ( 'NONE',  ( 8.540544597724410991, 99.50000000000000000, 19.98924338346217766 ) ) ;
#8765=CARTESIAN_POINT ( 'NONE',  ( -27.43301270000000969, 2.299999998907525267, 11.36312591709335784 ) ) ;
#8766=CARTESIAN_POINT ( 'NONE',  ( -19.09188309203678457, 1.899999999999999911, -19.09188309203678813 ) ) ;
#8767=CARTESIAN_POINT ( 'NONE',  ( -27.00000000000000355, 0.9499999978150504010, -11.18376618407357270 ) ) ;
#8769=DIRECTION ( 'NONE',  ( 0.9569724629708533659, 0.000000000000000000, -0.2901787468363226097 ) ) ;
#8770=CARTESIAN_POINT ( 'NONE',  ( -22.67573144110267336, 99.50000000000001421, -10.14737752305977381 ) ) ;
#8771=CARTESIAN_POINT ( 'NONE',  ( 8.074269155311188939, 100.0000000000000142, 20.56111086218762551 ) ) ;
#8774=ORIENTED_EDGE ( 'NONE', *, *, #1641, .T. ) ;
#8775=CARTESIAN_POINT ( 'NONE',  ( 4.584380863705032283, 100.0000000000000284, -24.21384527865288305 ) ) ;
#8776=DIRECTION ( 'NONE',  ( 1.000000000000000000, 0.000000000000000000, 0.000000000000000000 ) ) ;
#8777=CARTESIAN_POINT ( 'NONE',  ( 10.72103337977569204, 99.50000000000000000, 22.20268488987243316 ) ) ;
#8782=CARTESIAN_POINT ( 'NONE',  ( 2.940192896829773250, 99.50000000000001421, -23.44521981770616037 ) ) ;
#8784=DIRECTION ( 'NONE',  ( -0.000000000000000000, -1.000000000000000000, -0.000000000000000000 ) ) ;
#8786=CARTESIAN_POINT ( 'NONE',  ( -14.74935495356232984, 99.50000000000001421, 15.91322402822111926 ) ) ;
#8788=VERTEX_POINT ( 'NONE', #548 ) ;
#8790=AXIS2_PLACEMENT_3D ( 'NONE', #6325, #7204, #4853 ) ;
#8794=CARTESIAN_POINT ( 'NONE',  ( 11.18376618407357626, 2.049999997815050268, 27.00000000000000000 ) ) ;
#8796=CARTESIAN_POINT ( 'NONE',  ( -20.64578974631102426, 99.49999999999995737, -10.10077944494247504 ) ) ;
#8798=CARTESIAN_POINT ( 'NONE',  ( 3.214822648120007731, 100.0000000000000000, -21.86319392453323829 ) ) ;
#8800=CARTESIAN_POINT ( 'NONE',  ( 4.143207896384923039, 99.49999999999998579, -24.36264353342416911 ) ) ;
#8803=CARTESIAN_POINT ( 'NONE',  ( 19.39806930854668110, 2.049999998907525711, -19.39806930854668110 ) ) ;
#8805=CARTESIAN_POINT ( 'NONE',  ( 1.679787559701184688E-15, 5.349999998907525089, -27.43301270000000258 ) ) ;
#8806=CARTESIAN_POINT ( 'NONE',  ( 11.18376618407357626, 3.850000000000000089, 27.00000000000000000 ) ) ;
#8808=ORIENTED_EDGE ( 'NONE', *, *, #4146, .F. ) ;
#8809=VECTOR ( 'NONE', #10012, 1000.000000000000000 ) ;
#8810=FACE_OUTER_BOUND ( 'NONE', #3092, .T. ) ;
#8811=CARTESIAN_POINT ( 'NONE',  ( -20.93575003794465061, 99.50000000000001421, -10.12220034237898503 ) ) ;
#8812=CARTESIAN_POINT ( 'NONE',  ( 4.739008722453744049, 100.0000000000000142, -24.06821587619827696 ) ) ;
#8815=CARTESIAN_POINT ( 'NONE',  ( -5.039362679103552881E-15, 3.249999998907525001, 27.43301270000000258 ) ) ;
#8816=CARTESIAN_POINT ( 'NONE',  ( 1.653273178848927064E-15, 3.999999997815050889, -27.00000000000000355 ) ) ;
#8817=EDGE_CURVE ( 'NONE', #369, #2588, #7279, .T. ) ;
#8818=LINE ( 'NONE', #7290, #2402 ) ;
#8820=CARTESIAN_POINT ( 'NONE',  ( -16.36254897777739004, 100.0000000000000142, 15.39785597259249350 ) ) ;
#8821=CARTESIAN_POINT ( 'NONE',  ( -16.91946509138130139, 99.50000000000001421, 15.98858002463268413 ) ) ;
#8822=CARTESIAN_POINT ( 'NONE',  ( 8.102924533678123709, 100.0000000000000000, 20.98904009517733726 ) ) ;
#8823=ORIENTED_EDGE ( 'NONE', *, *, #3786, .F. ) ;
#8827=DIRECTION ( 'NONE',  ( -0.9198211419112228837, 0.000000000000000000, 0.3923379498508065000 ) ) ;
#8830=CARTESIAN_POINT ( 'NONE',  ( -14.75894607058735630, 100.0000000000000284, 15.77473972644577849 ) ) ;
#8832=LINE ( 'NONE', #1505, #9115 ) ;
#8833=AXIS2_PLACEMENT_3D ( 'NONE', #1979, #5768, #5173 ) ;
#8837=CARTESIAN_POINT ( 'NONE',  ( 19.09188309203678813, 3.099999997815050090, -19.09188309203678813 ) ) ;
#8838=CARTESIAN_POINT ( 'NONE',  ( 9.044794778432494908, 100.0000000000000142, 19.94873160813952140 ) ) ;
#8841=VECTOR ( 'NONE', #5091, 1000.000000000000114 ) ;
#8843=CARTESIAN_POINT ( 'NONE',  ( 1.653273178848927064E-15, 4.799999997815051600, -27.00000000000000355 ) ) ;
#8845=CARTESIAN_POINT ( 'NONE',  ( -21.16695614262292580, 99.50000000000000000, -11.33496398805607441 ) ) ;
#8846=CARTESIAN_POINT ( 'NONE',  ( 11.36312591709336139, 4.499999998907525445, -27.43301270000000258 ) ) ;
#8848=CARTESIAN_POINT ( 'NONE',  ( -20.66709314808276332, 100.0000000000000284, -10.01107456535036455 ) ) ;
#8850=CARTESIAN_POINT ( 'NONE',  ( 3.198738776810544415, 100.0000000000000142, -22.02447230026614022 ) ) ;
#8851=FACE_OUTER_BOUND ( 'NONE', #5407, .T. ) ;
#8853=CARTESIAN_POINT ( 'NONE',  ( 9.802580223201115217, 99.99999999999997158, 21.25247094773282086 ) ) ;
#8856=CARTESIAN_POINT ( 'NONE',  ( 27.43301269999999548, 1.899999998907525356, 11.36312591709337738 ) ) ;
#8857=CARTESIAN_POINT ( 'NONE',  ( -15.72775836928289017, 99.50000000000000000, 17.03252426573849476 ) ) ;
#8858=CARTESIAN_POINT ( 'NONE',  ( -19.09188309203678813, 3.700000000000000178, 19.09188309203678457 ) ) ;
#8859=CYLINDRICAL_SURFACE ( 'NONE', #9212, 27.00000000000000355 ) ;
#8862=DIRECTION ( 'NONE',  ( 0.9985355274883277454, 0.000000000000000000, -0.05409991075415104128 ) ) ;
#8864=CARTESIAN_POINT ( 'NONE',  ( -20.72805389903318130, 99.99999999999994316, -9.848585782927868237 ) ) ;
#8865=CARTESIAN_POINT ( 'NONE',  ( 27.43301270000000258, 2.649999998907525356, 0.000000000000000000 ) ) ;
#8866=CARTESIAN_POINT ( 'NONE',  ( -11.18376618407358336, 2.149999999999999911, 26.99999999999999645 ) ) ;
#8868=CARTESIAN_POINT ( 'NONE',  ( -22.33589105551819642, 100.0000000000000284, -11.18147695539509812 ) ) ;
#8870=DIRECTION ( 'NONE',  ( -0.000000000000000000, -1.000000000000000000, -0.000000000000000000 ) ) ;
#8871=CARTESIAN_POINT ( 'NONE',  ( 19.09188309203678102, 1.500000000000000000, 19.09188309203678813 ) ) ;
#8874=EDGE_CURVE ( 'NONE', #2013, #1313, #7502, .T. ) ;
#8876=EDGE_LOOP ( 'NONE', ( #9046, #6947, #2216, #3794 ) ) ;
#8878=CARTESIAN_POINT ( 'NONE',  ( 4.570993444255353921, 99.99999999999998579, -21.37574484917381668 ) ) ;
#8880=CARTESIAN_POINT ( 'NONE',  ( 9.820792995160308791, 99.50000000000000000, 20.21220011423140761 ) ) ;
#8883=CARTESIAN_POINT ( 'NONE',  ( 8.102924533678123709, 99.50000000000000000, 20.98904009517733726 ) ) ;
#8885=CARTESIAN_POINT ( 'NONE',  ( -14.83363727892122519, 99.50000000000001421, 15.50654517199034466 ) ) ;
#8888=DIRECTION ( 'NONE',  ( -0.000000000000000000, -1.000000000000000000, -0.000000000000000000 ) ) ;
#8889=CARTESIAN_POINT ( 'NONE',  ( 2.847408871211157155, 99.99999999999998579, -22.10537533382872510 ) ) ;
#8891=EDGE_CURVE ( 'NONE', #6656, #1438, #6749, .T. ) ;
#8894=CARTESIAN_POINT ( 'NONE',  ( 27.43301270000000258, 4.399999998907525800, -11.36312591709336139 ) ) ;
#8895=CARTESIAN_POINT ( 'NONE',  ( -19.75840245672548789, 100.0000000000000000, -8.735905494466331689 ) ) ;
#8897=CARTESIAN_POINT ( 'NONE',  ( -16.35834224700816009, 99.50000000000000000, 16.43761959438736397 ) ) ;
#8899=CARTESIAN_POINT ( 'NONE',  ( -22.24883010645271852, 99.49999999999997158, -10.75389422444101939 ) ) ;
#8901=ADVANCED_FACE ( 'NONE', ( #9947 ), #3935, .T. ) ;
#8902=VERTEX_POINT ( 'NONE', #587 ) ;
#8905=CARTESIAN_POINT ( 'NONE',  ( -27.00000000000000355, 4.400000000000000355, -3.306546357697854128E-15 ) ) ;
#8906=CARTESIAN_POINT ( 'NONE',  ( 2.874264611687397331, 100.0000000000000142, -22.24889838548798693 ) ) ;
#8909=CARTESIAN_POINT ( 'NONE',  ( -20.89948324804827706, 99.50000000000001421, -10.26098411820691858 ) ) ;
#8911=VERTEX_POINT ( 'NONE', #3882 ) ;
#8913=CARTESIAN_POINT ( 'NONE',  ( 3.472565890032746960, 100.0000000000000284, -24.54662015932514052 ) ) ;
#8918=CARTESIAN_POINT ( 'NONE',  ( -27.00000000000001421, 1.849999997815050534, 11.18376618407356560 ) ) ;
#8919=CARTESIAN_POINT ( 'NONE',  ( -16.92301558088953328, 100.0000000000000142, 15.88693424423437683 ) ) ;
#8920=CARTESIAN_POINT ( 'NONE',  ( 3.739209042966563867, 99.50000000000000000, -21.42288334414699236 ) ) ;
#8924=ORIENTED_EDGE ( 'NONE', *, *, #4672, .F. ) ;
#8925=CARTESIAN_POINT ( 'NONE',  ( 3.207057600658871355, 99.50000000000000000, -22.07913334414698880 ) ) ;
#8927=CARTESIAN_POINT ( 'NONE',  ( -22.28244091826395135, 99.50000000000000000, -10.68852969318427881 ) ) ;
#8931=DIRECTION ( 'NONE',  ( -0.000000000000000000, 1.000000000000000000, -0.000000000000000000 ) ) ;
#8934=B_SPLINE_CURVE_WITH_KNOTS ( 'NONE', 3,
 ( #6255, #3900, #6925, #10125, #8616, #7713, #2226, #3743, #4688, #9341, #8445, #5428, #3687, #6310, #657, #2171, #1441, #5369, #2904 ),
 .UNSPECIFIED., .F., .F.,
 ( 4, 1, 1, 1, 1, 1, 1, 1, 1, 1, 1, 1, 1, 1, 1, 1, 4 ),
 ( 0.000000000000000000, 0.06505403082392276215, 0.1283503816230405770, 0.1902281050068566903, 0.2509397092642763338, 0.3119571365542418429, 0.3738829716944830350, 0.4367040802691206092, 0.5009896104483916313, 0.5655726868558689224, 0.6286067690057803858, 0.6898677555008378981, 0.7506620835893632604, 0.8110632348575060879, 0.8726242918051292374, 0.9355756365154705989, 0.9999999999999998890 ),
 .UNSPECIFIED. ) ;
#8936=VECTOR ( 'NONE', #7180, 1000.000000000000000 ) ;
#8937=EDGE_CURVE ( 'NONE', #3431, #3123, #8752, .T. ) ;
#8938=CARTESIAN_POINT ( 'NONE',  ( 3.238942592553923472, 99.50000000000001421, -24.36085717291697250 ) ) ;
#8939=FACE_OUTER_BOUND ( 'NONE', #8093, .T. ) ;
#8940=CARTESIAN_POINT ( 'NONE',  ( 2.874264611687397331, 99.50000000000001421, -22.24889838548798693 ) ) ;
#8941=CARTESIAN_POINT ( 'NONE',  ( -27.00000000000000355, 3.399999997815049912, -3.306546357697854128E-15 ) ) ;
#8942=CARTESIAN_POINT ( 'NONE',  ( 2.940631318607589417, 100.0000000000000000, -23.77584808773673331 ) ) ;
#8943=DIRECTION ( 'NONE',  ( -0.000000000000000000, -1.000000000000000000, -0.000000000000000000 ) ) ;
#8944=CARTESIAN_POINT ( 'NONE',  ( 3.204253864046738176, 100.0000000000000000, -22.06071064728738662 ) ) ;
#8945=CARTESIAN_POINT ( 'NONE',  ( -21.99951964646687941, 99.50000000000001421, -11.00094659099690553 ) ) ;
#8947=AXIS2_PLACEMENT_3D ( 'NONE', #6485, #3929, #9531 ) ;
#8951=CARTESIAN_POINT ( 'NONE',  ( -15.03933290382598820, 99.50000000000000000, 15.19633946010233849 ) ) ;
#8952=VECTOR ( 'NONE', #5057, 999.9999999999998863 ) ;
#8953=CARTESIAN_POINT ( 'NONE',  ( 2.936358689207804851, 99.50000000000000000, -23.74786164940363875 ) ) ;
#8954=CARTESIAN_POINT ( 'NONE',  ( 19.09188309203678813, 4.899999999999999467, -19.09188309203678813 ) ) ;
#8957=CARTESIAN_POINT ( 'NONE',  ( 4.232798786556307036, 100.0000000000000000, -24.34936571594186105 ) ) ;
#8958=CARTESIAN_POINT ( 'NONE',  ( -4.959819536546781389E-15, 1.999999997815050445, 27.00000000000000355 ) ) ;
#8959=CIRCLE ( 'NONE', #5940, 18.00000000000000000 ) ;
#8960=VERTEX_POINT ( 'NONE', #744 ) ;
#8961=CARTESIAN_POINT ( 'NONE',  ( 7.726884419709978857, 99.50000000000000000, 20.74516479202295471 ) ) ;
#8962=EDGE_CURVE ( 'NONE', #9616, #9118, #667, .T. ) ;
#8964=CARTESIAN_POINT ( 'NONE',  ( -16.25072943800822500, 99.50000000000005684, 15.30228603765648820 ) ) ;
#8965=EDGE_CURVE ( 'NONE', #9210, #2398, #5658, .T. ) ;
#8966=CARTESIAN_POINT ( 'NONE',  ( -21.29537297865864431, 99.50000000000000000, -11.39144590536739976 ) ) ;
#8968=CARTESIAN_POINT ( 'NONE',  ( 9.044794778432494908, 99.50000000000001421, 19.94873160813952140 ) ) ;
#8969=CARTESIAN_POINT ( 'NONE',  ( -16.79604063091391097, 99.50000000000000000, 15.40463673182947701 ) ) ;
#8971=CARTESIAN_POINT ( 'NONE',  ( 4.401614252286283779, 100.0000000000000284, -24.65974366035752396 ) ) ;
#8973=ORIENTED_EDGE ( 'NONE', *, *, #3496, .T. ) ;
#8974=VECTOR ( 'NONE', #8292, 1000.000000000000000 ) ;
#8975=CARTESIAN_POINT ( 'NONE',  ( -22.33589105551819642, 100.0000000000000284, -11.18147695539509812 ) ) ;
#8978=CARTESIAN_POINT ( 'NONE',  ( 4.688812652749139609, 99.50000000000001421, -24.54863390154074310 ) ) ;
#8979=ORIENTED_EDGE ( 'NONE', *, *, #7162, .T. ) ;
#8980=DIRECTION ( 'NONE',  ( -0.000000000000000000, 1.000000000000000000, -0.000000000000000000 ) ) ;
#8982=CARTESIAN_POINT ( 'NONE',  ( -21.58460863908062066, 100.0000000000000284, -11.10356610083683648 ) ) ;
#8983=ORIENTED_EDGE ( 'NONE', *, *, #2927, .T. ) ;
#8984=CARTESIAN_POINT ( 'NONE',  ( 4.187832255138415505, 99.50000000000001421, -21.50835573230103037 ) ) ;
#8986=CARTESIAN_POINT ( 'NONE',  ( 4.122675185292913547, 99.99999999999994316, -22.83451320417363561 ) ) ;
#8987=CARTESIAN_POINT ( 'NONE',  ( 7.734522023158566739, 99.99999999999997158, 20.86022014488863618 ) ) ;
#8988=LINE ( 'NONE', #8253, #8439 ) ;
#8989=CARTESIAN_POINT ( 'NONE',  ( 11.18376618407356915, 3.949999997815050179, -27.00000000000000355 ) ) ;
#8990=CARTESIAN_POINT ( 'NONE',  ( 10.85214315541671759, 99.50000000000000000, 22.51047735782115211 ) ) ;
#8991=CARTESIAN_POINT ( 'NONE',  ( -21.00001322343447541, 100.0000000000000142, -9.990026185521596602 ) ) ;
#8992=CARTESIAN_POINT ( 'NONE',  ( -15.32348647777738826, 100.0000000000000000, 15.39505148541300450 ) ) ;
#8994=CARTESIAN_POINT ( 'NONE',  ( -22.20893716642541804, 100.0000000000000284, -10.81429252070940272 ) ) ;
#8995=CARTESIAN_POINT ( 'NONE',  ( 3.023131990384279710, 100.0000000000000284, -21.47496011329876708 ) ) ;
#8997=ORIENTED_EDGE ( 'NONE', *, *, #7717, .F. ) ;
#9001=CARTESIAN_POINT ( 'NONE',  ( 2.940631318607589417, 99.50000000000000000, -23.77584808773673331 ) ) ;
#9002=CARTESIAN_POINT ( 'NONE',  ( 11.36312591709336850, 4.099999998907525089, 27.43301269999999903 ) ) ;
#9003=CARTESIAN_POINT ( 'NONE',  ( -27.00000000000000355, 0.4000000000000000222, -3.306546357697854128E-15 ) ) ;
#9004=DIRECTION ( 'NONE',  ( 0.000000000000000000, 1.000000000000000000, 0.000000000000000000 ) ) ;
#9005=CARTESIAN_POINT ( 'NONE',  ( -21.12798922145720582, 99.99999999999998579, -10.90888695829967325 ) ) ;
#9006=EDGE_CURVE ( 'NONE', #4720, #3772, #2747, .T. ) ;
#9007=ORIENTED_EDGE ( 'NONE', *, *, #4397, .F. ) ;
#9008=CARTESIAN_POINT ( 'NONE',  ( -22.08823018108446234, 99.50000000000000000, -9.406177930363766038 ) ) ;
#9009=CARTESIAN_POINT ( 'NONE',  ( 2.971063225226878046, 100.0000000000000000, -23.91837856253154015 ) ) ;
#9010=LINE ( 'NONE', #4247, #4881 ) ;
#9012=CARTESIAN_POINT ( 'NONE',  ( -16.49882833452567965, 99.99999999999995737, 15.05677840364783115 ) ) ;
#9013=CARTESIAN_POINT ( 'NONE',  ( 9.245739950628269810, 99.50000000000002842, 20.03726560014620617 ) ) ;
#9014=LINE ( 'NONE', #6025, #7103 ) ;
#9015=CARTESIAN_POINT ( 'NONE',  ( 19.09188309203678102, 2.299999999999999822, 19.09188309203678813 ) ) ;
#9016=ADVANCED_FACE ( 'NONE', ( #5664 ), #898, .T. ) ;
#9017=B_SPLINE_CURVE_WITH_KNOTS ( 'NONE', 3,
 ( #6206, #6038, #9286, #3747, #9179, #7777, #9228, #9404, #9969, #6151, #6821, #2060, #4421, #1999, #5198, #9348, #8396, #5254, #442 ),
 .UNSPECIFIED., .F., .F.,
 ( 4, 1, 1, 1, 1, 1, 1, 1, 1, 1, 1, 1, 1, 1, 1, 1, 4 ),
 ( 0.000000000000000000, 0.06363772181477481138, 0.1253661190162797812, 0.1854850957718461035, 0.2454326483351531030, 0.3054881917026986415, 0.3659564384638642753, 0.4275766838088623234, 0.4913505196498278993, 0.5556437034595619329, 0.6183735394983103095, 0.6802114403575724166, 0.7422401234104337719, 0.8041288543812358247, 0.8678488776753463529, 0.9326351893241184854, 1.000000000000000000 ),
 .UNSPECIFIED. ) ;
#9018=EDGE_CURVE ( 'NONE', #6706, #1490, #4653, .T. ) ;
#9021=VERTEX_POINT ( 'NONE', #7447 ) ;
#9022=CARTESIAN_POINT ( 'NONE',  ( -21.71039561923405969, 100.0000000000000426, -11.44438725057713313 ) ) ;
#9023=CARTESIAN_POINT ( 'NONE',  ( 3.356341388373609291, 99.50000000000001421, -21.61643044175963979 ) ) ;
#9024=CARTESIAN_POINT ( 'NONE',  ( 4.154273145530666511, 99.50000000000000000, -22.82723029927519676 ) ) ;
#9025=CARTESIAN_POINT ( 'NONE',  ( -15.15871127190382417, 100.0000000000000000, 15.63231653451427761 ) ) ;
#9026=PLANE ( 'NONE',  #7624 ) ;
#9029=LINE ( 'NONE', #1846, #9338 ) ;
#9031=ORIENTED_EDGE ( 'NONE', *, *, #2850, .F. ) ;
#9032=FACE_OUTER_BOUND ( 'NONE', #9525, .T. ) ;
#9033=CARTESIAN_POINT ( 'NONE',  ( 19.39806930854668110, 5.149999998907524912, -19.39806930854668110 ) ) ;
#9034=LINE ( 'NONE', #3647, #8573 ) ;
#9035=B_SPLINE_CURVE_WITH_KNOTS ( 'NONE', 3,
 ( #4029, #936, #8742, #45, #10266, #5653, #7954, #1566, #4811, #9625, #8694, #3098, #4756, #787, #3979 ),
 .UNSPECIFIED., .F., .F.,
 ( 4, 1, 1, 1, 1, 1, 1, 1, 1, 1, 1, 1, 4 ),
 ( 0.000000000000000000, 0.1055296353700490852, 0.2070742529895955586, 0.3056622059958778448, 0.4023599870273183998, 0.4943057198019382148, 0.5778637904027289496, 0.6550095244395398586, 0.7278863574113029200, 0.7976678238154090161, 0.8645871040366396310, 0.9319858836656568224, 1.000000000000000000 ),
 .UNSPECIFIED. ) ;
#9037=CARTESIAN_POINT ( 'NONE',  ( 4.049441352997683374, 99.99999999999997158, -21.43849541167161732 ) ) ;
#9038=CARTESIAN_POINT ( 'NONE',  ( -15.31787750341841559, 100.0000000000000000, 16.43551622900274722 ) ) ;
#9039=CARTESIAN_POINT ( 'NONE',  ( -27.00000000000000355, 2.599999997815050534, -3.306546357697854128E-15 ) ) ;
#9041=CARTESIAN_POINT ( 'NONE',  ( -21.45221949983897858, 100.0000000000000000, -9.661157428473494235 ) ) ;
#9042=CARTESIAN_POINT ( 'NONE',  ( 3.293841816516395848, 99.99999999999998579, -23.44781013845121009 ) ) ;
#9043=CARTESIAN_POINT ( 'NONE',  ( -22.24883010645271852, 99.99999999999997158, -10.75389422444101939 ) ) ;
#9044=DIRECTION ( 'NONE',  ( -0.9567912676219745283, 0.000000000000000000, 0.2907756355032780071 ) ) ;
#9045=CARTESIAN_POINT ( 'NONE',  ( 0.000000000000000000, 100.0000000000000000, -27.00000000000000355 ) ) ;
#9046=ORIENTED_EDGE ( 'NONE', *, *, #956, .F. ) ;
#9048=EDGE_CURVE ( 'NONE', #7160, #4075, #394, .T. ) ;
#9049=CARTESIAN_POINT ( 'NONE',  ( -15.56505537928961047, 99.50000000000002842, 14.87309967080592088 ) ) ;
#9050=CARTESIAN_POINT ( 'NONE',  ( 2.852289972453743161, 99.50000000000000000, -22.14293542748032451 ) ) ;
#9052=B_SPLINE_CURVE_WITH_KNOTS ( 'NONE', 3,
 ( #3539, #5843, #8940, #401, #4226, #7509, #9818, #1758, #347, #1856, #6728 ),
 .UNSPECIFIED., .F., .F.,
 ( 4, 1, 1, 1, 1, 1, 1, 1, 4 ),
 ( 0.000000000000000000, 0.1243175037779491315, 0.2437391319546453605, 0.3610119291759345539, 0.4796059399169178006, 0.5994854737745749507, 0.7252340722053824962, 0.8585022233306516259, 1.000000000000000000 ),
 .UNSPECIFIED. ) ;
#9053=CARTESIAN_POINT ( 'NONE',  ( -19.39806930854668465, 3.949999998907525178, 19.39806930854667755 ) ) ;
#9055=VECTOR ( 'NONE', #6315, 1000.000000000000114 ) ;
#9058=CARTESIAN_POINT ( 'NONE',  ( -11.18376618407358336, 4.349999997815050534, 26.99999999999999645 ) ) ;
#9059=EDGE_LOOP ( 'NONE', ( #4443, #6868, #2761, #7223 ) ) ;
#9060=CARTESIAN_POINT ( 'NONE',  ( 7.753999887479250397, 99.50000000000000000, 20.97676509141502166 ) ) ;
#9061=CARTESIAN_POINT ( 'NONE',  ( -27.43301270000000258, 4.599999998907525978, -11.36312591709336317 ) ) ;
#9063=CARTESIAN_POINT ( 'NONE',  ( -21.43094455402013310, 99.50000000000000000, -11.42705968398779426 ) ) ;
#9064=CARTESIAN_POINT ( 'NONE',  ( 4.472992770554171216, 99.99999999999998579, -21.83386288566719458 ) ) ;
#9066=EDGE_CURVE ( 'NONE', #341, #2567, #9287, .T. ) ;
#9067=CARTESIAN_POINT ( 'NONE',  ( 9.583828860305853681, 99.99999999999992895, 20.68614437522342797 ) ) ;
#9068=DIRECTION ( 'NONE',  ( 1.000000000000000000, 0.000000000000000000, -0.000000000000000000 ) ) ;
#9070=VERTEX_POINT ( 'NONE', #2178 ) ;
#9071=CARTESIAN_POINT ( 'NONE',  ( -16.35834224700816009, 99.50000000000000000, 16.43761959438736397 ) ) ;
#9076=CARTESIAN_POINT ( 'NONE',  ( 3.681717055787076642, 100.0000000000000000, -21.09125273517263111 ) ) ;
#9077=CARTESIAN_POINT ( 'NONE',  ( 3.552835461024879127, 99.50000000000000000, -21.47801279722421697 ) ) ;
#9079=CARTESIAN_POINT ( 'NONE',  ( -15.13293277027690209, 100.0000000000000000, 16.13104881108577970 ) ) ;
#9081=CARTESIAN_POINT ( 'NONE',  ( 4.739008722453744049, 100.0000000000000142, -24.06821587619827696 ) ) ;
#9082=CARTESIAN_POINT ( 'NONE',  ( 3.597125852879613728, 99.49999999999998579, -24.22990373345680126 ) ) ;
#9083=ORIENTED_EDGE ( 'NONE', *, *, #4088, .F. ) ;
#9085=CARTESIAN_POINT ( 'NONE',  ( 19.39806930854667399, 4.249999998907525445, 19.39806930854668465 ) ) ;
#9086=DIRECTION ( 'NONE',  ( 0.000000000000000000, 0.000000000000000000, 1.000000000000000000 ) ) ;
#9087=EDGE_CURVE ( 'NONE', #498, #7819, #7044, .T. ) ;
#9088=CARTESIAN_POINT ( 'NONE',  ( 21.47055288461538325, 99.50000000000000000, -0.7081330128205128860 ) ) ;
#9089=CARTESIAN_POINT ( 'NONE',  ( 7.753999887479250397, 99.99999999999994316, 20.97676509141502166 ) ) ;
#9091=CARTESIAN_POINT ( 'NONE',  ( 3.252389375388976323, 100.0000000000000711, -22.22144413113850447 ) ) ;
#9092=CARTESIAN_POINT ( 'NONE',  ( -11.18376618407358336, 3.549999997815050268, 26.99999999999999645 ) ) ;
#9095=CARTESIAN_POINT ( 'NONE',  ( 4.122675185292913547, 99.99999999999997158, -22.83451320417363561 ) ) ;
#9096=CARTESIAN_POINT ( 'NONE',  ( -21.93524539549613550, 99.99999999999998579, -11.03420246938663318 ) ) ;
#9100=CARTESIAN_POINT ( 'NONE',  ( -14.74935495356232984, 99.50000000000001421, 15.91322402822111926 ) ) ;
#9102=CARTESIAN_POINT ( 'NONE',  ( 19.39806930854668110, 3.549999998907525267, -19.39806930854668110 ) ) ;
#9103=CARTESIAN_POINT ( 'NONE',  ( -19.09188309203678813, 0.5000000000000000000, 19.09188309203678457 ) ) ;
#9104=DIRECTION ( 'NONE',  ( -0.5137073458062109133, 0.000000000000000000, -0.8579654788304353907 ) ) ;
#9105=FACE_OUTER_BOUND ( 'NONE', #7527, .T. ) ;
#9106=CARTESIAN_POINT ( 'NONE',  ( 7.746148141271532950, 100.0000000000000284, 20.51930889200067298 ) ) ;
#9107=CIRCLE ( 'NONE', #420, 25.15000000000000213 ) ;
#9111=PLANE ( 'NONE',  #4283 ) ;
#9112=CARTESIAN_POINT ( 'NONE',  ( 9.554054106072296548, 99.50000000000001421, 20.45778517829714360 ) ) ;
#9113=CARTESIAN_POINT ( 'NONE',  ( -21.16695614262292580, 99.50000000000000000, -11.33496398805607441 ) ) ;
#9115=VECTOR ( 'NONE', #879, 1000.000000000000227 ) ;
#9116=CARTESIAN_POINT ( 'NONE',  ( 9.389534246205572643, 99.50000000000001421, 21.46805835725047729 ) ) ;
#9117=CARTESIAN_POINT ( 'NONE',  ( 11.18376618407357626, 2.250000000000000888, 27.00000000000000000 ) ) ;
#9118=VERTEX_POINT ( 'NONE', #10249 ) ;
#9120=CARTESIAN_POINT ( 'NONE',  ( -16.34021191015031249, 99.50000000000000000, 16.45483272884350967 ) ) ;
#9124=CARTESIAN_POINT ( 'NONE',  ( -22.51488550592518934, 99.49999999999997158, -10.97145172607810615 ) ) ;
#9126=CARTESIAN_POINT ( 'NONE',  ( -27.00000000000000355, 4.949999997815051067, -11.18376618407357270 ) ) ;
#9128=CARTESIAN_POINT ( 'NONE',  ( 4.599186066243659887, 99.50000000000002842, -24.59301055568561623 ) ) ;
#9129=CARTESIAN_POINT ( 'NONE',  ( -15.10382517959271098, 99.49999999999998579, 15.91526905993627317 ) ) ;
#9130=AXIS2_PLACEMENT_3D ( 'NONE', #5094, #2698, #340 ) ;
#9132=CARTESIAN_POINT ( 'NONE',  ( -21.99951964646687941, 100.0000000000000142, -11.00094659099690553 ) ) ;
#9136=CARTESIAN_POINT ( 'NONE',  ( 27.43301269999999548, 5.099999998907525978, 11.36312591709337738 ) ) ;
#9138=CARTESIAN_POINT ( 'NONE',  ( 3.472565890032746960, 99.50000000000002842, -24.54662015932514052 ) ) ;
#9139=CARTESIAN_POINT ( 'NONE',  ( 3.775125937424839151, 99.50000000000000000, -21.41825520325024712 ) ) ;
#9141=CARTESIAN_POINT ( 'NONE',  ( 3.563396934924631942, 100.0000000000000426, -22.47881610735839431 ) ) ;
#9142=CARTESIAN_POINT ( 'NONE',  ( -27.00000000000000355, 3.349999997815050090, -11.18376618407357093 ) ) ;
#9143=EDGE_CURVE ( 'NONE', #3764, #2804, #5175, .T. ) ;
#9145=CARTESIAN_POINT ( 'NONE',  ( -21.91899880027261460, 100.0000000000000000, -9.705014769524845875 ) ) ;
#9148=ORIENTED_EDGE ( 'NONE', *, *, #1606, .F. ) ;
#9149=CARTESIAN_POINT ( 'NONE',  ( 4.887668416326221177, 99.50000000000001421, -23.70513093767710089 ) ) ;
#9154=DIRECTION ( 'NONE',  ( -0.2907782774943305504, 0.000000000000000000, -0.9567904646982169359 ) ) ;
#9156=CARTESIAN_POINT ( 'NONE',  ( 27.43301270000000258, 3.499999998907525445, -11.36312591709336139 ) ) ;
#9157=EDGE_LOOP ( 'NONE', ( #928, #9267, #5770, #7592 ) ) ;
#9160=DIRECTION ( 'NONE',  ( -0.5190318799156541374, 0.000000000000000000, -0.8547548816071318667 ) ) ;
#9161=CARTESIAN_POINT ( 'NONE',  ( -21.11719860449141351, 99.99999999999995737, -9.425423427278841970 ) ) ;
#9163=EDGE_LOOP ( 'NONE', ( #6976, #8728, #3348, #2792 ) ) ;
#9165=CARTESIAN_POINT ( 'NONE',  ( -15.34161522349497808, 99.49999999999998579, 15.37783959465231121 ) ) ;
#9166=CARTESIAN_POINT ( 'NONE',  ( -16.60513711880303234, 99.99999999999997158, 15.15667007515659748 ) ) ;
#9167=FACE_OUTER_BOUND ( 'NONE', #8149, .T. ) ;
#9168=CARTESIAN_POINT ( 'NONE',  ( -21.45221949983897858, 100.0000000000000000, -9.661157428473494235 ) ) ;
#9170=CARTESIAN_POINT ( 'NONE',  ( 4.750280232731688201, 100.0000000000000284, -24.05275076595185624 ) ) ;
#9171=B_SPLINE_CURVE_WITH_KNOTS ( 'NONE', 3,
 ( #4017, #5639, #29, #1796, #1017, #5591, #8830, #140, #3283, #7303, #875, #4943, #7393, #2395, #185 ),
 .UNSPECIFIED., .F., .F.,
 ( 4, 1, 1, 1, 1, 1, 1, 1, 1, 1, 1, 1, 4 ),
 ( 0.000000000000000000, 0.08490232564366416435, 0.1680779112633816463, 0.2506304657828534177, 0.3338427399641299420, 0.4169763759729993580, 0.4990117930239920674, 0.5811067191809071719, 0.6656374296971073745, 0.7500328835558887075, 0.8331455368193440014, 0.9159638734519762737, 1.000000000000000000 ),
 .UNSPECIFIED. ) ;
#9173=VERTEX_POINT ( 'NONE', #3031 ) ;
#9174=DIRECTION ( 'NONE',  ( -0.2907782774943305504, 0.000000000000000000, -0.9567904646982169359 ) ) ;
#9176=CARTESIAN_POINT ( 'NONE',  ( 3.750007936853901658, 99.50000000000001421, -22.95001988029826734 ) ) ;
#9177=CARTESIAN_POINT ( 'NONE',  ( -27.00000000000000355, 3.399999997815049912, -3.306546357697854128E-15 ) ) ;
#9178=ADVANCED_FACE ( 'NONE', ( #4584 ), #443, .T. ) ;
#9179=CARTESIAN_POINT ( 'NONE',  ( -16.81182640597031508, 100.0000000000000000, 16.36129326314865295 ) ) ;
#9180=CARTESIAN_POINT ( 'NONE',  ( 3.386276725104728769, 99.50000000000001421, -24.01678749451497907 ) ) ;
#9181=( BOUNDED_CURVE ( )  B_SPLINE_CURVE ( 2, ( #6363, #9698, #8087, #2385, #9557, #8918, #3225, #3127, #4108 ),
 .UNSPECIFIED., .F., .T. ) 
 B_SPLINE_CURVE_WITH_KNOTS ( ( 3, 2, 2, 2, 3 ),
 ( 0.1785714285714285754, 0.1964285714285714246, 0.2142857142857142738, 0.2321428571428571508, 0.2500000000000000000 ),
 .UNSPECIFIED. ) 
 CURVE ( )  GEOMETRIC_REPRESENTATION_ITEM ( )  RATIONAL_B_SPLINE_CURVE ( ( 1.000000000000000000, 0.9238795325112867385, 1.000000000000000000, 0.9238795325112867385, 1.000000000000000000, 0.9238795325112867385, 1.000000000000000000, 0.9238795325112867385, 1.000000000000000000 ) ) 
 REPRESENTATION_ITEM ( '' )  );
#9183=DIRECTION ( 'NONE',  ( -0.000000000000000000, 1.000000000000000000, -0.000000000000000000 ) ) ;
#9184=CARTESIAN_POINT ( 'NONE',  ( -19.39806930854667755, 3.049999998907525711, -19.39806930854668110 ) ) ;
#9186=CARTESIAN_POINT ( 'NONE',  ( 9.723125805078051798, 99.50000000000000000, 21.50134635983626907 ) ) ;
#9187=EDGE_CURVE ( 'NONE', #6069, #7809, #9405, .T. ) ;
#9188=ORIENTED_EDGE ( 'NONE', *, *, #9518, .T. ) ;
#9189=CARTESIAN_POINT ( 'NONE',  ( -21.11719860449141351, 100.0000000000000284, -9.425423427278841970 ) ) ;
#9190=CARTESIAN_POINT ( 'NONE',  ( 8.751508028230254865, 99.99999999999998579, 19.58480916780017722 ) ) ;
#9191=CARTESIAN_POINT ( 'NONE',  ( 27.00000000000000355, 3.200000000000000178, 0.000000000000000000 ) ) ;
#9192=FACE_OUTER_BOUND ( 'NONE', #9253, .T. ) ;
#9194=ORIENTED_EDGE ( 'NONE', *, *, #85, .F. ) ;
#9195=CARTESIAN_POINT ( 'NONE',  ( -15.98972951825121669, 99.49999999999997158, 15.19400804711857411 ) ) ;
#9196=CARTESIAN_POINT ( 'NONE',  ( -11.36312591709337561, 2.499999998907525445, 27.43301269999999548 ) ) ;
#9197=ORIENTED_EDGE ( 'NONE', *, *, #7406, .T. ) ;
#9199=CARTESIAN_POINT ( 'NONE',  ( 3.106448761625311139, 99.49999999999998579, -21.38062202216113761 ) ) ;
#9201=CARTESIAN_POINT ( 'NONE',  ( 27.43301269999999548, 2.599999998907525089, 11.36312591709337738 ) ) ;
#9202=CARTESIAN_POINT ( 'NONE',  ( 1.653273178848927064E-15, 1.800000000000000266, -27.00000000000000355 ) ) ;
#9203=CARTESIAN_POINT ( 'NONE',  ( 8.536201443755420115, 100.0000000000000284, 19.63502355897212581 ) ) ;
#9204=CARTESIAN_POINT ( 'NONE',  ( 3.810791133452845703, 100.0000000000000568, -24.33305202239136733 ) ) ;
#9205=CARTESIAN_POINT ( 'NONE',  ( 3.349514647153394975, 99.99999999999998579, -23.95461210612682024 ) ) ;
#9209=CARTESIAN_POINT ( 'NONE',  ( 11.36312591709336850, 0.8999999989075253559, 27.43301269999999903 ) ) ;
#9210=VERTEX_POINT ( 'NONE', #2233 ) ;
#9211=CARTESIAN_POINT ( 'NONE',  ( 19.09188309203678813, 4.899999999999999467, -19.09188309203678813 ) ) ;
#9212=AXIS2_PLACEMENT_3D ( 'NONE', #4924, #6545, #8025 ) ;
#9214=CARTESIAN_POINT ( 'NONE',  ( 3.986298408513477387, 99.50000000000002842, -22.53092616755505162 ) ) ;
#9217=CARTESIAN_POINT ( 'NONE',  ( 4.871887406949175769, 99.99999999999995737, -23.77896509604281405 ) ) ;
#9220=CARTESIAN_POINT ( 'NONE',  ( 4.723706824522782455, 99.50000000000000000, -24.08630974238606370 ) ) ;
#9223=CARTESIAN_POINT ( 'NONE',  ( 2.936358689207804851, 100.0000000000000000, -23.74786164940363875 ) ) ;
#9225=VECTOR ( 'NONE', #6697, 1000.000000000000000 ) ;
#9226=ORIENTED_EDGE ( 'NONE', *, *, #2174, .F. ) ;
#9227=CARTESIAN_POINT ( 'NONE',  ( 3.948639947730041566, 99.49999999999998579, -21.07692942975820927 ) ) ;
#9228=CARTESIAN_POINT ( 'NONE',  ( -16.88522588321459494, 100.0000000000000284, 16.18266969485829421 ) ) ;
#9231=CARTESIAN_POINT ( 'NONE',  ( 19.09188309203678102, 1.299999997815050268, 19.09188309203678813 ) ) ;
#9232=CARTESIAN_POINT ( 'NONE',  ( -5.039362679103552881E-15, 4.949999998907525622, 27.43301270000000258 ) ) ;
#9233=CARTESIAN_POINT ( 'NONE',  ( 4.909381318607588973, 100.0000000000000000, -23.54377677363417121 ) ) ;
#9234=CARTESIAN_POINT ( 'NONE',  ( 9.766630880609509902, 100.0000000000000142, 21.37293705761699059 ) ) ;
#9235=CARTESIAN_POINT ( 'NONE',  ( -21.99154324187120579, 100.0000000000000142, -9.362771248264911250 ) ) ;
#9236=CARTESIAN_POINT ( 'NONE',  ( 4.688812652749139609, 99.50000000000001421, -24.54863390154074310 ) ) ;
#9239=CARTESIAN_POINT ( 'NONE',  ( -16.57687742313193269, 99.50000000000002842, 15.91855687263828756 ) ) ;
#9241=ORIENTED_EDGE ( 'NONE', *, *, #10227, .F. ) ;
#9242=CARTESIAN_POINT ( 'NONE',  ( -16.36470918167357169, 99.50000000000000000, 16.79054296464299867 ) ) ;
#9243=CARTESIAN_POINT ( 'NONE',  ( -19.39806930854668465, 2.449999998907525622, 19.39806930854667755 ) ) ;
#9245=ADVANCED_FACE ( 'NONE', ( #3857 ), #90, .T. ) ;
#9248=CARTESIAN_POINT ( 'NONE',  ( 9.182805720491336032, 99.50000000000000000, 20.00174565872165289 ) ) ;
#9251=CARTESIAN_POINT ( 'NONE',  ( 19.39806930854667399, 4.949999998907525622, 19.39806930854668465 ) ) ;
#9252=CARTESIAN_POINT ( 'NONE',  ( -5.039362679103552881E-15, 2.549999998907525267, 27.43301270000000258 ) ) ;
#9253=EDGE_LOOP ( 'NONE', ( #113, #2343 ) ) ;
#9256=CARTESIAN_POINT ( 'NONE',  ( -15.17782247516205274, 99.99999999999998579, 15.06300032623928686 ) ) ;
#9257=DIRECTION ( 'NONE',  ( 0.9985355274883277454, 0.000000000000000000, -0.05409991075415104128 ) ) ;
#9258=CARTESIAN_POINT ( 'NONE',  ( 7.783718120363267268, 99.99999999999998579, 21.09473326129887027 ) ) ;
#9260=CARTESIAN_POINT ( 'NONE',  ( -15.49723655759404295, 99.99999999999997158, 15.26389171799780264 ) ) ;
#9262=CARTESIAN_POINT ( 'NONE',  ( -21.29537297865864431, 99.50000000000000000, -11.39144590536739976 ) ) ;
#9265=CARTESIAN_POINT ( 'NONE',  ( 1.679787559701184688E-15, 2.049999998907525711, -27.43301270000000258 ) ) ;
#9267=ORIENTED_EDGE ( 'NONE', *, *, #6476, .F. ) ;
#9268=CARTESIAN_POINT ( 'NONE',  ( -15.07178375341841559, 99.50000000000001421, 15.16157792772069968 ) ) ;
#9269=CARTESIAN_POINT ( 'NONE',  ( 26.99999999999999645, 1.550000000000000044, 11.18376618407358691 ) ) ;
#9270=CARTESIAN_POINT ( 'NONE',  ( 6.477538756577482459, 99.50000000000000000, 20.49684993083915430 ) ) ;
#9273=CARTESIAN_POINT ( 'NONE',  ( -15.91084591538827198, 99.50000000000001421, 16.65047278764667027 ) ) ;
#9278=CARTESIAN_POINT ( 'NONE',  ( -22.12191435419165941, 99.99999999999998579, -9.834338183724410598 ) ) ;
#9279=CARTESIAN_POINT ( 'NONE',  ( -15.07178375341841381, 100.0000000000000000, 16.66969090848992607 ) ) ;
#9280=DIRECTION ( 'NONE',  ( -0.9854855627156250408, 0.000000000000000000, -0.1697592580069431922 ) ) ;
#9282=CARTESIAN_POINT ( 'NONE',  ( 2.940631318607589417, 100.0000000000000000, -23.77584808773673331 ) ) ;
#9284=ORIENTED_EDGE ( 'NONE', *, *, #2500, .T. ) ;
#9285=CARTESIAN_POINT ( 'NONE',  ( 3.861186820804014097, 99.50000000000004263, -21.07288982789904708 ) ) ;
#9286=CARTESIAN_POINT ( 'NONE',  ( -16.70213339477928471, 99.99999999999998579, 16.52464093453885852 ) ) ;
#9287=LINE ( 'NONE', #2854, #7804 ) ;
#9288=ORIENTED_EDGE ( 'NONE', *, *, #5103, .T. ) ;
#9290=CARTESIAN_POINT ( 'NONE',  ( -11.36312591709335962, 2.999999998907524557, -27.43301270000000258 ) ) ;
#9292=PLANE ( 'NONE',  #5086 ) ;
#9293=VERTEX_POINT ( 'NONE', #873 ) ;
#9295=CARTESIAN_POINT ( 'NONE',  ( 5.242860087038358152, 99.50000000000002842, -23.52699316036146371 ) ) ;
#9299=CARTESIAN_POINT ( 'NONE',  ( -15.91768310440539658, 99.50000000000002842, 15.18344740530786652 ) ) ;
#9301=CARTESIAN_POINT ( 'NONE',  ( -11.36312591709335962, 0.5999999989075253115, -27.43301270000000258 ) ) ;
#9306=CARTESIAN_POINT ( 'NONE',  ( -22.43208371148383762, 99.50000000000000000, -9.654966607469265938 ) ) ;
#9307=CARTESIAN_POINT ( 'NONE',  ( 2.901827748664965068, 99.49999999999998579, -21.68759887446373469 ) ) ;
#9309=CARTESIAN_POINT ( 'NONE',  ( -16.84090648038580085, 99.49999999999998579, 15.49469789757679727 ) ) ;
#9310=CARTESIAN_POINT ( 'NONE',  ( -19.39806930854667755, 3.049999998907525711, -19.39806930854668110 ) ) ;
#9311=ORIENTED_EDGE ( 'NONE', *, *, #8817, .F. ) ;
#9312=ORIENTED_EDGE ( 'NONE', *, *, #820, .F. ) ;
#9313=EDGE_CURVE ( 'NONE', #2748, #7711, #7249, .T. ) ;
#9314=B_SPLINE_CURVE_WITH_KNOTS ( 'NONE', 3,
 ( #2979, #8632, #10026, #1236 ),
 .UNSPECIFIED., .F., .F.,
 ( 4, 4 ),
 ( 0.000000000000000000, 1.000000000000000000 ),
 .UNSPECIFIED. ) ;
#9315=CARTESIAN_POINT ( 'NONE',  ( 9.063633472794011325, 99.99999999999998579, 19.59517414759687526 ) ) ;
#9316=CARTESIAN_POINT ( 'NONE',  ( 8.105710127743357418, 99.50000000000000000, 20.44429669797862559 ) ) ;
#9317=CARTESIAN_POINT ( 'NONE',  ( -16.42071764973191250, 99.50000000000001421, 16.76105279315999042 ) ) ;
#9318=CARTESIAN_POINT ( 'NONE',  ( 3.282077632710153292, 100.0000000000000000, -23.74569985055724786 ) ) ;
#9322=ORIENTED_EDGE ( 'NONE', *, *, #1009, .F. ) ;
#9324=CARTESIAN_POINT ( 'NONE',  ( -11.36312591709335962, 2.899999998907525356, -27.43301270000000258 ) ) ;
#9325=ORIENTED_EDGE ( 'NONE', *, *, #9664, .F. ) ;
#9326=CARTESIAN_POINT ( 'NONE',  ( -15.70584307919286893, 99.99999999999995737, 14.84247401567675162 ) ) ;
#9327=CARTESIAN_POINT ( 'NONE',  ( -27.00000000000000355, 0.4000000000000000222, -3.306546357697854128E-15 ) ) ;
#9328=VECTOR ( 'NONE', #10337, 1000.000000000000000 ) ;
#9329=CARTESIAN_POINT ( 'NONE',  ( 9.304660012616079001, 100.0000000000000284, 20.07619068507570859 ) ) ;
#9330=ORIENTED_EDGE ( 'NONE', *, *, #2246, .F. ) ;
#9333=CARTESIAN_POINT ( 'NONE',  ( -16.45635306197508996, 99.99999999999995737, 15.51056558312563105 ) ) ;
#9334=FACE_OUTER_BOUND ( 'NONE', #5191, .T. ) ;
#9337=ORIENTED_EDGE ( 'NONE', *, *, #1160, .F. ) ;
#9338=VECTOR ( 'NONE', #4265, 1000.000000000000000 ) ;
#9339=CARTESIAN_POINT ( 'NONE',  ( -22.57971655928959365, 99.50000000000000000, -10.84768434062017839 ) ) ;
#9340=CARTESIAN_POINT ( 'NONE',  ( -19.39806930854668465, 0.7499999989075252227, 19.39806930854667755 ) ) ;
#9341=CARTESIAN_POINT ( 'NONE',  ( -21.38163724633288965, 99.50000000000005684, -9.681902434707239991 ) ) ;
#9345=CARTESIAN_POINT ( 'NONE',  ( -19.75840245672548789, 99.50000000000000000, -8.735905494466331689 ) ) ;
#9346=EDGE_CURVE ( 'NONE', #1470, #2280, #8142, .T. ) ;
#9348=CARTESIAN_POINT ( 'NONE',  ( -16.74216497804568604, 100.0000000000000142, 15.31795814478965312 ) ) ;
#9354=CARTESIAN_POINT ( 'NONE',  ( 9.676361905416721143, 100.0000000000000000, 21.63547735782115566 ) ) ;
#9355=B_SPLINE_SURFACE_WITH_KNOTS ( 'NONE', 3, 1, ( 
 ( #8059, #894 ),
 ( #3299, #9145 ),
 ( #2609, #4328 ),
 ( #2656, #1812 ),
 ( #7512, #9821 ),
 ( #8204, #202 ),
 ( #7361, #2564 ),
 ( #3491, #5846 ),
 ( #351, #9041 ),
 ( #3387, #1034 ),
 ( #5953, #9770 ),
 ( #6579, #156 ),
 ( #5755, #5159 ),
 ( #5800, #7408 ),
 ( #2709, #5898 ),
 ( #8256, #5004 ),
 ( #249, #8991 ),
 ( #1859, #4229 ),
 ( #2763, #3436 ) ),
 .UNSPECIFIED., .F., .F., .F.,
 ( 4, 1, 1, 1, 1, 1, 1, 1, 1, 1, 1, 1, 1, 1, 1, 1, 4 ),
 ( 2, 2 ),
 ( 0.000000000000000000, 0.06505403082392276215, 0.1283503816230405770, 0.1902281050068566903, 0.2509397092642763338, 0.3119571365542418429, 0.3738829716944830350, 0.4367040802691206092, 0.5009896104483916313, 0.5655726868558689224, 0.6286067690057803858, 0.6898677555008378981, 0.7506620835893632604, 0.8110632348575060879, 0.8726242918051292374, 0.9355756365154705989, 0.9999999999999998890 ),
 ( 0.000000000000000000, 1.000000000000000000 ),
 .UNSPECIFIED. ) ;
#9356=ORIENTED_EDGE ( 'NONE', *, *, #1606, .T. ) ;
#9359=CARTESIAN_POINT ( 'NONE',  ( 8.961048541867139505, 100.0000000000000142, 19.57961630251783092 ) ) ;
#9360=CARTESIAN_POINT ( 'NONE',  ( -16.07368679829020763, 99.50000000000000000, 17.11560437002838952 ) ) ;
#9361=CARTESIAN_POINT ( 'NONE',  ( -16.49419651247312046, 99.49999999999998579, 15.57134447358898477 ) ) ;
#9364=CARTESIAN_POINT ( 'NONE',  ( -11.36312591709335962, 1.399999998907525578, -27.43301270000000258 ) ) ;
#9365=EDGE_LOOP ( 'NONE', ( #6550, #6840, #4324, #6316 ) ) ;
#9371=CARTESIAN_POINT ( 'NONE',  ( -19.39806930854668465, 2.449999998907525622, 19.39806930854667755 ) ) ;
#9372=ORIENTED_EDGE ( 'NONE', *, *, #5394, .F. ) ;
#9373=CARTESIAN_POINT ( 'NONE',  ( -16.12311789350856017, 100.0000000000000000, 14.86696503675854686 ) ) ;
#9374=LINE ( 'NONE', #7014, #2135 ) ;
#9375=CARTESIAN_POINT ( 'NONE',  ( 2.864934851235464208, 99.50000000000000000, -21.80148171563692827 ) ) ;
#9377=CIRCLE ( 'NONE', #4183, 27.00000000000000355 ) ;
#9379=CARTESIAN_POINT ( 'NONE',  ( 4.433602057339688152, 100.0000000000000000, -21.25644978738549540 ) ) ;
#9381=FACE_OUTER_BOUND ( 'NONE', #8509, .T. ) ;
#9382=CARTESIAN_POINT ( 'NONE',  ( 11.36312591709336139, 2.799999998907525267, -27.43301270000000258 ) ) ;
#9383=EDGE_LOOP ( 'NONE', ( #4685, #267, #662, #8283 ) ) ;
#9384=LINE ( 'NONE', #10282, #236 ) ;
#9385=CARTESIAN_POINT ( 'NONE',  ( 3.207057600658871355, 99.50000000000000000, -22.07913334414698880 ) ) ;
#9386=CARTESIAN_POINT ( 'NONE',  ( 9.357295078982289738, 100.0000000000000711, 20.12145687760884627 ) ) ;
#9388=EDGE_LOOP ( 'NONE', ( #2872, #4908, #226, #5476 ) ) ;
#9389=CARTESIAN_POINT ( 'NONE',  ( -15.32348647777738826, 99.50000000000000000, 15.39505148541300450 ) ) ;
#9390=CARTESIAN_POINT ( 'NONE',  ( -15.37123125604856710, 99.50000000000001421, 16.48683530611566539 ) ) ;
#9393=ORIENTED_EDGE ( 'NONE', *, *, #9851, .T. ) ;
#9394=PLANE ( 'NONE',  #1456 ) ;
#9397=EDGE_CURVE ( 'NONE', #1366, #9616, #8240, .T. ) ;
#9399=CARTESIAN_POINT ( 'NONE',  ( 5.243816414761435674, 100.0000000000000284, -23.48558366465980995 ) ) ;
#9400=VERTEX_POINT ( 'NONE', #4016 ) ;
#9404=CARTESIAN_POINT ( 'NONE',  ( -16.90689012439429462, 99.99999999999998579, 16.08742389234230785 ) ) ;
#9405=LINE ( 'NONE', #6095, #786 ) ;
#9406=VERTEX_POINT ( 'NONE', #7884 ) ;
#9409=VECTOR ( 'NONE', #8862, 1000.000000000000000 ) ;
#9410=VERTEX_POINT ( 'NONE', #9661 ) ;
#9412=CARTESIAN_POINT ( 'NONE',  ( 4.401614252286283779, 99.50000000000002842, -24.65974366035752396 ) ) ;
#9414=CARTESIAN_POINT ( 'NONE',  ( -16.49092618789450526, 99.50000000000000000, 16.26472549871478179 ) ) ;
#9417=ORIENTED_EDGE ( 'NONE', *, *, #9720, .T. ) ;
#9418=LINE ( 'NONE', #7679, #7140 ) ;
#9419=CIRCLE ( 'NONE', #3906, 27.00000000000000355 ) ;
#9420=CARTESIAN_POINT ( 'NONE',  ( -11.36312591709337561, 0.8999999989075252449, 27.43301269999999548 ) ) ;
#9421=ORIENTED_EDGE ( 'NONE', *, *, #7468, .T. ) ;
#9425=CARTESIAN_POINT ( 'NONE',  ( 3.023131990384279710, 100.0000000000000000, -21.47496011329876708 ) ) ;
#9427=CARTESIAN_POINT ( 'NONE',  ( -5.039362679103552881E-15, 4.849999998907525089, 27.43301270000000258 ) ) ;
#9428=CARTESIAN_POINT ( 'NONE',  ( 27.43301270000000258, 1.999999998907524779, -11.36312591709336139 ) ) ;
#9431=CARTESIAN_POINT ( 'NONE',  ( 8.429066232339796017, 100.0000000000000000, 19.67794530653910101 ) ) ;
#9432=CARTESIAN_POINT ( 'NONE',  ( 4.202475441399873723, 100.0000000000000000, -24.35385978717689071 ) ) ;
#9433=CARTESIAN_POINT ( 'NONE',  ( 3.399971579580567393, 99.50000000000000000, -21.57509867787664248 ) ) ;
#9434=CARTESIAN_POINT ( 'NONE',  ( 7.486453019397995234, 99.50000000000000000, 23.81666162955709964 ) ) ;
#9436=CARTESIAN_POINT ( 'NONE',  ( 4.743081672682207817, 100.0000000000000284, -21.60795120912350598 ) ) ;
#9437=ORIENTED_EDGE ( 'NONE', *, *, #3903, .F. ) ;
#9438=ORIENTED_EDGE ( 'NONE', *, *, #1008, .T. ) ;
#9440=CARTESIAN_POINT ( 'NONE',  ( -11.36312591709335962, 2.099999998907525089, -27.43301270000000258 ) ) ;
#9443=CARTESIAN_POINT ( 'NONE',  ( 11.18376618407357626, 2.250000000000000444, 27.00000000000000000 ) ) ;
#9444=CARTESIAN_POINT ( 'NONE',  ( 8.757234875838378230, 99.50000000000000000, 19.92790116963689329 ) ) ;
#9445=ORIENTED_EDGE ( 'NONE', *, *, #3027, .F. ) ;
#9446=CARTESIAN_POINT ( 'NONE',  ( -15.10617644529808423, 99.50000000000002842, 15.98944417891004477 ) ) ;
#9447=CARTESIAN_POINT ( 'NONE',  ( -15.55395551812965671, 100.0000000000000284, 16.59868653893595791 ) ) ;
#9448=ORIENTED_EDGE ( 'NONE', *, *, #4537, .T. ) ;
#9451=ORIENTED_EDGE ( 'NONE', *, *, #1453, .F. ) ;
#9452=CARTESIAN_POINT ( 'NONE',  ( 19.39806930854667399, 1.749999998907525223, 19.39806930854668465 ) ) ;
#9455=B_SPLINE_SURFACE_WITH_KNOTS ( 'NONE', 3, 1, ( 
 ( #4863, #3198 ),
 ( #9478, #7260 ),
 ( #5505, #888 ),
 ( #6380, #1515 ),
 ( #4708, #7901 ),
 ( #5601, #1617 ),
 ( #7114, #1756 ),
 ( #6670, #982 ),
 ( #4174, #7402 ),
 ( #7313, #4273 ),
 ( #3379, #6725 ),
 ( #4998, #7356 ),
 ( #5892, #151 ),
 ( #8198, #6574 ),
 ( #4322, #196 ),
 ( #5749, #9866 ),
 ( #6622, #2703 ),
 ( #5841, #8986 ),
 ( #345, #3486 ) ),
 .UNSPECIFIED., .F., .F., .F.,
 ( 4, 1, 1, 1, 1, 1, 1, 1, 1, 1, 1, 1, 1, 1, 1, 1, 4 ),
 ( 2, 2 ),
 ( 0.000000000000000000, 0.07039602572822099835, 0.1400447079551435658, 0.2099027554305550880, 0.2826152692239142783, 0.3556467613428230812, 0.4271065942619623468, 0.4986634349892335449, 0.5720141774457471184, 0.6112909118483191850, 0.6543288624652392471, 0.7009162800881839628, 0.7518538071550001645, 0.8072437197097745987, 0.8671654997918389896, 0.9315515937071113806, 1.000000000000000000 ),
 ( 0.000000000000000000, 1.000000000000000000 ),
 .UNSPECIFIED. ) ;
#9457=CARTESIAN_POINT ( 'NONE',  ( 5.098880966732203035, 99.50000000000000000, -24.13374913903897223 ) ) ;
#9458=DIRECTION ( 'NONE',  ( 0.000000000000000000, 0.000000000000000000, 1.000000000000000000 ) ) ;
#9459=EDGE_CURVE ( 'NONE', #5889, #5894, #3474, .T. ) ;
#9462=CARTESIAN_POINT ( 'NONE',  ( 3.948639947730041566, 99.99999999999998579, -21.07692942975820927 ) ) ;
#9463=CARTESIAN_POINT ( 'NONE',  ( 1.653273178848927064E-15, 1.000000000000000000, -27.00000000000000355 ) ) ;
#9464=CARTESIAN_POINT ( 'NONE',  ( 9.164845778125666698, 99.50000000000001421, 19.62003801130714820 ) ) ;
#9467=CARTESIAN_POINT ( 'NONE',  ( 3.044406660298407452, 99.50000000000000000, -23.15442635585071685 ) ) ;
#9468=CARTESIAN_POINT ( 'NONE',  ( 9.445361748092775400, 100.0000000000000142, 19.75398588445988324 ) ) ;
#9469=EDGE_CURVE ( 'NONE', #5423, #6706, #5139, .T. ) ;
#9473=CARTESIAN_POINT ( 'NONE',  ( -14.97579057656165169, 99.50000000000001421, 16.56690896377573452 ) ) ;
#9474=CARTESIAN_POINT ( 'NONE',  ( 27.43301270000000258, 4.349999998907525089, 0.000000000000000000 ) ) ;
#9477=AXIS2_PLACEMENT_3D ( 'NONE', #7391, #1794, #2688 ) ;
#9478=CARTESIAN_POINT ( 'NONE',  ( 3.277744210708366079, 99.50000000000001421, -23.71256836663369327 ) ) ;
#9480=EDGE_CURVE ( 'NONE', #4830, #1392, #232, .T. ) ;
#9481=CARTESIAN_POINT ( 'NONE',  ( -16.87593989452418697, 99.49999999999998579, 15.58794934546231126 ) ) ;
#9482=CARTESIAN_POINT ( 'NONE',  ( -19.39806930854667755, 3.849999998907525089, -19.39806930854668110 ) ) ;
#9484=ADVANCED_FACE ( 'NONE', ( #972 ), #2918, .T. ) ;
#9485=CARTESIAN_POINT ( 'NONE',  ( 4.909381318607588973, 99.50000000000000000, -23.54377677363417121 ) ) ;
#9486=CARTESIAN_POINT ( 'NONE',  ( 3.428794695218988053, 100.0000000000000142, -24.07607503615978572 ) ) ;
#9487=CARTESIAN_POINT ( 'NONE',  ( 2.843562173796539749, 99.50000000000001421, -21.91597968833000110 ) ) ;
#9488=CARTESIAN_POINT ( 'NONE',  ( -22.08823018108446234, 100.0000000000000000, -9.406177930363766038 ) ) ;
#9489=VECTOR ( 'NONE', #5596, 1000.000000000000114 ) ;
#9491=CARTESIAN_POINT ( 'NONE',  ( 4.358720771404392735, 99.50000000000000000, -21.20742720589606378 ) ) ;
#9493=CARTESIAN_POINT ( 'NONE',  ( -11.36312591709335962, 0.5999999989075250895, -27.43301270000000258 ) ) ;
#9495=VECTOR ( 'NONE', #10000, 1000.000000000000114 ) ;
#9497=CARTESIAN_POINT ( 'NONE',  ( -27.00000000000000355, 2.750000000000000888, -11.18376618407357093 ) ) ;
#9498=CARTESIAN_POINT ( 'NONE',  ( 9.404665101723468368, 99.50000000000000000, 20.17141824467128686 ) ) ;
#9501=CARTESIAN_POINT ( 'NONE',  ( -16.36254897777738648, 99.99999999999995737, 15.39785597259249172 ) ) ;
#9502=CARTESIAN_POINT ( 'NONE',  ( 8.132491713109027742, 100.0000000000000142, 21.08089001807756446 ) ) ;
#9504=ORIENTED_EDGE ( 'NONE', *, *, #3753, .T. ) ;
#9505=CARTESIAN_POINT ( 'NONE',  ( 11.36312591709336139, 2.799999998907524823, -27.43301270000000258 ) ) ;
#9506=CARTESIAN_POINT ( 'NONE',  ( 3.409892249890944527, 99.50000000000000000, -24.50637943905448779 ) ) ;
#9513=CARTESIAN_POINT ( 'NONE',  ( 4.433602057339688152, 100.0000000000000000, -21.25644978738549540 ) ) ;
#9517=B_SPLINE_CURVE_WITH_KNOTS ( 'NONE', 3,
 ( #8820, #7090, #8035, #6412, #131, #10295, #868, #9602, #9651, #3320, #2434, #5532, #7142, #4058, #2489, #1695, #4892, #917, #5868 ),
 .UNSPECIFIED., .F., .F.,
 ( 4, 1, 1, 1, 1, 1, 1, 1, 1, 1, 1, 1, 1, 1, 1, 1, 4 ),
 ( 0.000000000000000000, 0.06442465027149940626, 0.1272622498775801414, 0.1890519169419207224, 0.2498421757728049863, 0.3110425729590077792, 0.3720985300252119266, 0.4351465435385043490, 0.5001170788027262670, 0.5644817420234762295, 0.6276143074669133792, 0.6889588046791949028, 0.7501592018653976401, 0.8106582772613761811, 0.8724479443257179279, 0.9351683423010851426, 1.000000000000000000 ),
 .UNSPECIFIED. ) ;
#9518=EDGE_CURVE ( 'NONE', #5650, #1313, #3523, .T. ) ;
#9521=CARTESIAN_POINT ( 'NONE',  ( 3.058419780146050648, 99.50000000000000000, -23.12871267107006545 ) ) ;
#9523=CARTESIAN_POINT ( 'NONE',  ( -16.18965924272485779, 99.49999999999998579, 15.26525457555968224 ) ) ;
#9524=CARTESIAN_POINT ( 'NONE',  ( 27.43301270000000258, 4.399999998907524912, -11.36312591709336139 ) ) ;
#9525=EDGE_LOOP ( 'NONE', ( #9571, #6051, #4663, #6276 ) ) ;
#9527=EDGE_CURVE ( 'NONE', #7809, #4040, #8338, .T. ) ;
#9529=CARTESIAN_POINT ( 'NONE',  ( -20.89948324804827706, 100.0000000000000142, -10.26098411820691858 ) ) ;
#9531=DIRECTION ( 'NONE',  ( 1.000000000000000000, 0.000000000000000000, 0.000000000000000000 ) ) ;
#9532=CARTESIAN_POINT ( 'NONE',  ( -11.18376618407358336, 1.949999997815050401, 26.99999999999999645 ) ) ;
#9533=FACE_OUTER_BOUND ( 'NONE', #637, .T. ) ;
#9534=CARTESIAN_POINT ( 'NONE',  ( 3.535161742238301041, 100.0000000000000142, -24.18247714022527006 ) ) ;
#9535=CARTESIAN_POINT ( 'NONE',  ( 3.611424427577684781, 99.50000000000001421, -21.45475674085064099 ) ) ;
#9537=CARTESIAN_POINT ( 'NONE',  ( 27.00000000000000355, 4.000000000000000000, 0.000000000000000000 ) ) ;
#9539=CARTESIAN_POINT ( 'NONE',  ( 4.280752963211088336, 99.99999999999997158, -21.16602454745684270 ) ) ;
#9542=CARTESIAN_POINT ( 'NONE',  ( 27.43301270000000258, 0.3999999989075252449, -11.36312591709336139 ) ) ;
#9544=CARTESIAN_POINT ( 'NONE',  ( 27.43301270000000258, 0.2999999989075253226, -11.36312591709336139 ) ) ;
#9545=CARTESIAN_POINT ( 'NONE',  ( 3.028692941384139026, 100.0000000000000142, -22.52214499033115302 ) ) ;
#9548=CARTESIAN_POINT ( 'NONE',  ( -15.62070810370258833, 99.50000000000000000, 16.62245103965875970 ) ) ;
#9549=ORIENTED_EDGE ( 'NONE', *, *, #3419, .F. ) ;
#9552=CARTESIAN_POINT ( 'NONE',  ( 11.36312591709336850, 1.699999998907525400, 27.43301269999999903 ) ) ;
#9553=CARTESIAN_POINT ( 'NONE',  ( 3.350143586568126164, 99.50000000000001421, -24.46212657588250394 ) ) ;
#9555=CARTESIAN_POINT ( 'NONE',  ( -22.43115009631934953, 99.50000000000001421, -11.08196351649073819 ) ) ;
#9557=CARTESIAN_POINT ( 'NONE',  ( -27.00000000000000355, 1.799999997815050490, -3.306546357697854128E-15 ) ) ;
#9558=CARTESIAN_POINT ( 'NONE',  ( -16.81182640597031508, 99.50000000000000000, 16.36129326314865295 ) ) ;
#9562=CARTESIAN_POINT ( 'NONE',  ( 10.85214315541671759, 99.50000000000000000, 22.51047735782115211 ) ) ;
#9567=CARTESIAN_POINT ( 'NONE',  ( 2.927917759182871560, 99.49999999999997158, -23.69257214368879261 ) ) ;
#9569=DIRECTION ( 'NONE',  ( -0.000000000000000000, 1.000000000000000000, -0.000000000000000000 ) ) ;
#9570=CARTESIAN_POINT ( 'NONE',  ( 27.43301270000000258, 3.599999998907525534, -11.36312591709336139 ) ) ;
#9571=ORIENTED_EDGE ( 'NONE', *, *, #3890, .F. ) ;
#9573=CARTESIAN_POINT ( 'NONE',  ( -20.93486371557392545, 99.99999999999998579, -10.61231311368802466 ) ) ;
#9575=CARTESIAN_POINT ( 'NONE',  ( -20.70854316912038229, 100.0000000000000142, -10.95957977981033515 ) ) ;
#9576=CARTESIAN_POINT ( 'NONE',  ( 19.39806930854668110, 4.449999998907525622, -19.39806930854668110 ) ) ;
#9577=AXIS2_PLACEMENT_3D ( 'NONE', #1256, #9886, #6850 ) ;
#9578=CARTESIAN_POINT ( 'NONE',  ( -15.11748654497029953, 99.99999999999995737, 15.76872032455190897 ) ) ;
#9579=CARTESIAN_POINT ( 'NONE',  ( 3.349514647153394975, 99.99999999999998579, -23.95461210612682024 ) ) ;
#9580=CARTESIAN_POINT ( 'NONE',  ( 3.739209042966563867, 100.0000000000000000, -21.42288334414699236 ) ) ;
#9581=ADVANCED_FACE ( 'NONE', ( #5246, #7825 ), #9394, .T. ) ;
#9586=CARTESIAN_POINT ( 'NONE',  ( -27.43301270000000258, 0.6999999989075252893, -11.36312591709336317 ) ) ;
#9588=LINE ( 'NONE', #7915, #8936 ) ;
#9589=( GEOMETRIC_REPRESENTATION_CONTEXT ( 3 ) GLOBAL_UNCERTAINTY_ASSIGNED_CONTEXT ( ( #8010 ) ) GLOBAL_UNIT_ASSIGNED_CONTEXT ( ( #1005, #2675, #7481 ) ) REPRESENTATION_CONTEXT ( 'NONE', 'WORKASPACE' ) );
#9590=CARTESIAN_POINT ( 'NONE',  ( -11.18376618407356560, 3.450000000000000178, -27.00000000000000355 ) ) ;
#9591=PLANE ( 'NONE',  #877 ) ;
#9592=CARTESIAN_POINT ( 'NONE',  ( -16.37547766376588854, 99.99999999999995737, 16.41943072543956816 ) ) ;
#9593=CARTESIAN_POINT ( 'NONE',  ( 8.540544597724410991, 99.50000000000000000, 19.98924338346217766 ) ) ;
#9598=CARTESIAN_POINT ( 'NONE',  ( 27.43301270000000258, 1.899999998907525134, -11.36312591709336139 ) ) ;
#9599=CARTESIAN_POINT ( 'NONE',  ( 2.950788281418828429, 99.50000000000001421, -23.82341910423825837 ) ) ;
#9600=DIRECTION ( 'NONE',  ( 0.3924386850477849520, 0.000000000000000000, 0.9197781680807419757 ) ) ;
#9602=CARTESIAN_POINT ( 'NONE',  ( -16.56356094049941419, 99.99999999999997158, 15.77213757552179629 ) ) ;
#9603=CARTESIAN_POINT ( 'NONE',  ( -22.67573144110267336, 100.0000000000000142, -10.14737752305977381 ) ) ;
#9608=ORIENTED_EDGE ( 'NONE', *, *, #8746, .F. ) ;
#9609=CARTESIAN_POINT ( 'NONE',  ( 4.386516977709190357, 100.0000000000000568, -24.31220192127581825 ) ) ;
#9610=CARTESIAN_POINT ( 'NONE',  ( -20.63666786535793207, 99.49999999999998579, -10.16306733409737717 ) ) ;
#9611=CARTESIAN_POINT ( 'NONE',  ( -21.72555844818415594, 99.50000000000001421, -11.09629251537910655 ) ) ;
#9615=CARTESIAN_POINT ( 'NONE',  ( -22.17094027205346052, 100.0000000000000142, -9.884352203306939089 ) ) ;
#9616=VERTEX_POINT ( 'NONE', #436 ) ;
#9617=VECTOR ( 'NONE', #296, 1000.000000000000000 ) ;
#9619=CARTESIAN_POINT ( 'NONE',  ( -21.96365545856212265, 99.50000000000001421, -9.726658277667754149 ) ) ;
#9620=CARTESIAN_POINT ( 'NONE',  ( 27.00000000000000355, 3.049999997815050268, -11.18376618407356915 ) ) ;
#9621=CARTESIAN_POINT ( 'NONE',  ( 19.39806930854668110, 5.249999998907525445, -19.39806930854668110 ) ) ;
#9624=VECTOR ( 'NONE', #5121, 1000.000000000000000 ) ;
#9625=CARTESIAN_POINT ( 'NONE',  ( 3.341734429721257005, 100.0000000000000000, -22.34498040423979148 ) ) ;
#9627=CARTESIAN_POINT ( 'NONE',  ( -20.89145576992255116, 99.49999999999997158, -10.33073932272468198 ) ) ;
#9628=CARTESIAN_POINT ( 'NONE',  ( 27.00000000000000355, 2.199999997815050623, 0.000000000000000000 ) ) ;
#9630=CARTESIAN_POINT ( 'NONE',  ( 3.282077632710153292, 99.50000000000000000, -23.74569985055724786 ) ) ;
#9631=CARTESIAN_POINT ( 'NONE',  ( 3.739209042966563867, 99.50000000000000000, -21.42288334414699236 ) ) ;
#9634=CARTESIAN_POINT ( 'NONE',  ( 9.902568905804752575, 99.99999999999998579, 20.48863403721516363 ) ) ;
#9635=EDGE_LOOP ( 'NONE', ( #2868, #819, #4574, #1835 ) ) ;
#9637=CARTESIAN_POINT ( 'NONE',  ( 11.36312591709336139, 0.4999999989075251672, -27.43301270000000258 ) ) ;
#9641=CARTESIAN_POINT ( 'NONE',  ( 26.99999999999999645, 4.750000000000001776, 11.18376618407358691 ) ) ;
#9642=CARTESIAN_POINT ( 'NONE',  ( -21.13504512532655610, 100.0000000000000000, -11.31853095674525100 ) ) ;
#9643=AXIS2_PLACEMENT_3D ( 'NONE', #6856, #2209, #5355 ) ;
#9644=CARTESIAN_POINT ( 'NONE',  ( -21.18296228862668329, 100.0000000000000000, -10.95406920104765724 ) ) ;
#9645=CARTESIAN_POINT ( 'NONE',  ( 24.91446314102564230, 99.50000000000000000, -1.581029647435897578 ) ) ;
#9647=AXIS2_PLACEMENT_3D ( 'NONE', #5804, #1764, #7364 ) ;
#9648=CARTESIAN_POINT ( 'NONE',  ( 1.679787559701184688E-15, 1.249999998907525223, -27.43301270000000258 ) ) ;
#9649=CYLINDRICAL_SURFACE ( 'NONE', #3386, 27.00000000000000355 ) ;
#9651=CARTESIAN_POINT ( 'NONE',  ( -16.57330815294036697, 100.0000000000000142, 15.84440382193293217 ) ) ;
#9652=EDGE_CURVE ( 'NONE', #1073, #3821, #1223, .T. ) ;
#9653=CARTESIAN_POINT ( 'NONE',  ( -16.90147242988460263, 99.49999999999998579, 15.68472263728856753 ) ) ;
#9654=CARTESIAN_POINT ( 'NONE',  ( 8.091962505948220752, 99.99999999999995737, 20.48385654212622242 ) ) ;
#9655=VERTEX_POINT ( 'NONE', #493 ) ;
#9659=EDGE_LOOP ( 'NONE', ( #4275, #120, #4048, #4127 ) ) ;
#9660=CARTESIAN_POINT ( 'NONE',  ( 4.584380863705032283, 99.50000000000001421, -24.21384527865288305 ) ) ;
#9661=CARTESIAN_POINT ( 'NONE',  ( -15.32348647777738826, 99.50000000000000000, 15.39505148541300450 ) ) ;
#9662=DIRECTION ( 'NONE',  ( 0.8660254037844393737, 0.4999999999999988898, 0.000000000000000000 ) ) ;
#9664=EDGE_CURVE ( 'NONE', #2104, #498, #5236, .T. ) ;
#9665=ORIENTED_EDGE ( 'NONE', *, *, #874, .F. ) ;
#9667=EDGE_CURVE ( 'NONE', #7275, #7177, #4576, .T. ) ;
#9669=CARTESIAN_POINT ( 'NONE',  ( 19.09188309203678102, 2.899999997815050357, 19.09188309203678813 ) ) ;
#9670=CARTESIAN_POINT ( 'NONE',  ( 9.404665101723468368, 100.0000000000000000, 20.17141824467128686 ) ) ;
#9671=CARTESIAN_POINT ( 'NONE',  ( 4.472992770554171216, 99.49999999999998579, -21.83386288566719458 ) ) ;
#9672=EDGE_CURVE ( 'NONE', #653, #7728, #10210, .T. ) ;
#9673=CARTESIAN_POINT ( 'NONE',  ( 2.837666006185522782, 99.50000000000000000, -22.03040394835428373 ) ) ;
#9675=VERTEX_POINT ( 'NONE', #1102 ) ;
#9676=CARTESIAN_POINT ( 'NONE',  ( 4.100286767325537873, 100.0000000000000284, -22.51382885696750336 ) ) ;
#9677=CARTESIAN_POINT ( 'NONE',  ( -11.36312591709337383, 4.899999998907526688, 27.43301269999999548 ) ) ;
#9678=DIRECTION ( 'NONE',  ( 0.2499845035238856816, 0.000000000000000000, -0.9682498375925071565 ) ) ;
#9679=CARTESIAN_POINT ( 'NONE',  ( 3.535161742238301041, 99.50000000000001421, -24.18247714022527006 ) ) ;
#9680=CARTESIAN_POINT ( 'NONE',  ( 3.269123371500344710, 100.0000000000000142, -23.64665713169964434 ) ) ;
#9681=CARTESIAN_POINT ( 'NONE',  ( -22.21668755910108928, 100.0000000000000426, -9.472979539922778969 ) ) ;
#9687=CARTESIAN_POINT ( 'NONE',  ( -16.60513711880302878, 99.50000000000000000, 15.15667007515659570 ) ) ;
#9688=CARTESIAN_POINT ( 'NONE',  ( -11.36312591709337383, 0.7999999989075252671, 27.43301269999999548 ) ) ;
#9689=CARTESIAN_POINT ( 'NONE',  ( 10.72103337977569204, 99.50000000000000000, 22.20268488987243316 ) ) ;
#9691=CARTESIAN_POINT ( 'NONE',  ( -20.91430522584054330, 99.50000000000001421, -10.19152558580213608 ) ) ;
#9692=ORIENTED_EDGE ( 'NONE', *, *, #7602, .T. ) ;
#9694=CARTESIAN_POINT ( 'NONE',  ( 19.39806930854668110, 5.149999998907524912, -19.39806930854668110 ) ) ;
#9696=CARTESIAN_POINT ( 'NONE',  ( -19.09188309203678813, 1.099999997815050312, 19.09188309203678457 ) ) ;
#9698=CARTESIAN_POINT ( 'NONE',  ( -11.18376618407356737, 1.649999997815050579, -27.00000000000000355 ) ) ;
#9699=B_SPLINE_CURVE_WITH_KNOTS ( 'NONE', 3,
 ( #8428, #4448, #4398, #6799, #8373, #6963, #2885, #7753, #6068, #9999, #3002, #1204, #1258, #421, #9205, #4502, #7694, #6233, #9318 ),
 .UNSPECIFIED., .F., .F.,
 ( 4, 1, 1, 1, 1, 1, 1, 1, 1, 1, 1, 1, 1, 1, 1, 1, 4 ),
 ( 0.000000000000000000, 0.07313710028058939550, 0.1429478298248799129, 0.2105045057187734658, 0.2751999312753631854, 0.3390602298032547868, 0.4018764873508149926, 0.4650016082884899093, 0.5281538368899733049, 0.5906348070863262079, 0.6510495490485337378, 0.7103018853965116230, 0.7674338915725752441, 0.8249350906448947862, 0.8823686014076175255, 0.9405824579944982444, 1.000000000000000000 ),
 .UNSPECIFIED. ) ;
#9700=CARTESIAN_POINT ( 'NONE',  ( -16.60513711880302878, 99.50000000000000000, 15.15667007515659570 ) ) ;
#9701=CARTESIAN_POINT ( 'NONE',  ( 8.132491713109025966, 100.0000000000000000, 21.08089001807756091 ) ) ;
#9703=ORIENTED_EDGE ( 'NONE', *, *, #1009, .T. ) ;
#9704=EDGE_CURVE ( 'NONE', #5989, #4002, #5385, .T. ) ;
#9706=CARTESIAN_POINT ( 'NONE',  ( -22.35673484330673944, 99.50000000000001421, -10.41320610523044721 ) ) ;
#9708=CARTESIAN_POINT ( 'NONE',  ( -17.94007301623892658, 99.50000000000000000, 17.49000340848992607 ) ) ;
#9710=ORIENTED_EDGE ( 'NONE', *, *, #966, .T. ) ;
#9711=CARTESIAN_POINT ( 'NONE',  ( -15.31787750341841559, 99.50000000000001421, 16.43551622900274722 ) ) ;
#9714=CARTESIAN_POINT ( 'NONE',  ( 8.684839681857363658, 100.0000000000000142, 19.94043386883836178 ) ) ;
#9716=VECTOR ( 'NONE', #8096, 1000.000000000000114 ) ;
#9717=CARTESIAN_POINT ( 'NONE',  ( 3.845216150098881513, 99.50000000000000000, -21.40922359334548020 ) ) ;
#9718=CARTESIAN_POINT ( 'NONE',  ( -20.61566945723384592, 99.50000000000000000, -10.83949095114527594 ) ) ;
#9719=CARTESIAN_POINT ( 'NONE',  ( 19.09188309203678102, 1.299999997815050268, 19.09188309203678813 ) ) ;
#9720=EDGE_CURVE ( 'NONE', #6902, #463, #4104, .T. ) ;
#9721=CARTESIAN_POINT ( 'NONE',  ( -20.70854316912038229, 99.50000000000001421, -10.95957977981033515 ) ) ;
#9723=CARTESIAN_POINT ( 'NONE',  ( -15.91084591538827198, 99.50000000000001421, 16.65047278764667027 ) ) ;
#9726=CARTESIAN_POINT ( 'NONE',  ( -22.11394672483139701, 100.0000000000000000, -10.91855052283267646 ) ) ;
#9727=CYLINDRICAL_SURFACE ( 'NONE', #9647, 25.15000000000000213 ) ;
#9731=DIRECTION ( 'NONE',  ( -0.000000000000000000, 1.000000000000000000, -0.000000000000000000 ) ) ;
#9733=CARTESIAN_POINT ( 'NONE',  ( 11.18376618407356915, 4.150000000000000355, -27.00000000000000355 ) ) ;
#9735=LINE ( 'NONE', #3452, #5262 ) ;
#9737=CARTESIAN_POINT ( 'NONE',  ( -19.75840245672548789, 99.50000000000000000, -8.735905494466331689 ) ) ;
#9738=CARTESIAN_POINT ( 'NONE',  ( -21.28703419482447146, 99.99999999999994316, -11.01737971290317297 ) ) ;
#9739=CARTESIAN_POINT ( 'NONE',  ( 1.653273178848927064E-15, 0.2000000000000000111, -27.00000000000000355 ) ) ;
#9741=DIRECTION ( 'NONE',  ( -0.3368610894541371747, 0.000000000000000000, 0.9415543565890243105 ) ) ;
#9743=CARTESIAN_POINT ( 'NONE',  ( -19.39806930854668465, 0.7499999989075251117, 19.39806930854667755 ) ) ;
#9744=DIRECTION ( 'NONE',  ( 1.000000000000000000, 0.000000000000000000, 0.000000000000000000 ) ) ;
#9746=CARTESIAN_POINT ( 'NONE',  ( -22.69331084068295112, 99.49999999999998579, -10.43328931840349050 ) ) ;
#9747=CARTESIAN_POINT ( 'NONE',  ( -22.67341330918043951, 100.0000000000000000, -10.57563951594260665 ) ) ;
#9748=CARTESIAN_POINT ( 'NONE',  ( 26.99999999999999645, 5.349999997815049646, 11.18376618407358691 ) ) ;
#9753=CARTESIAN_POINT ( 'NONE',  ( -22.34945848979098670, 99.50000000000002842, -10.27225542379191481 ) ) ;
#9754=CARTESIAN_POINT ( 'NONE',  ( 3.717146347979291665, 99.99999999999997158, -21.42716062222556417 ) ) ;
#9755=DIRECTION ( 'NONE',  ( 0.8579654788304353907, 0.000000000000000000, -0.5137073458062109133 ) ) ;
#9757=ADVANCED_FACE ( 'NONE', ( #7427 ), #9111, .T. ) ;
#9760=CARTESIAN_POINT ( 'NONE',  ( -4.959819536546781389E-15, 2.799999997815050268, 27.00000000000000355 ) ) ;
#9761=CARTESIAN_POINT ( 'NONE',  ( 3.124251205490514494, 99.50000000000000000, -23.02140944421609703 ) ) ;
#9763=FACE_OUTER_BOUND ( 'NONE', #7342, .T. ) ;
#9766=ORIENTED_EDGE ( 'NONE', *, *, #1596, .T. ) ;
#9767=CARTESIAN_POINT ( 'NONE',  ( 9.820792995160308791, 99.50000000000000000, 20.21220011423140761 ) ) ;
#9768=CARTESIAN_POINT ( 'NONE',  ( -27.00000000000001421, 2.649999997815050357, 11.18376618407356382 ) ) ;
#9770=CARTESIAN_POINT ( 'NONE',  ( -21.31369174262763622, 99.99999999999997158, -9.710155485040722567 ) ) ;
#9772=CARTESIAN_POINT ( 'NONE',  ( -21.37606745505193473, 100.0000000000000284, -11.05925878703054011 ) ) ;
#9775=ORIENTED_EDGE ( 'NONE', *, *, #10245, .F. ) ;
#9779=CARTESIAN_POINT ( 'NONE',  ( 2.924645347134957163, 99.50000000000001421, -23.60918035669702064 ) ) ;
#9780=CARTESIAN_POINT ( 'NONE',  ( 1.679787559701184688E-15, 2.849999998907525534, -27.43301270000000258 ) ) ;
#9781=CARTESIAN_POINT ( 'NONE',  ( 27.43301270000000258, 0.3999999989075252449, -11.36312591709336139 ) ) ;
#9782=DIRECTION ( 'NONE',  ( 0.000000000000000000, 0.000000000000000000, -1.000000000000000000 ) ) ;
#9783=CARTESIAN_POINT ( 'NONE',  ( 0.000000000000000000, 85.00000000000000000, 0.000000000000000000 ) ) ;
#9784=CARTESIAN_POINT ( 'NONE',  ( -21.03403678956047074, 99.99999999999998579, -10.80451401317004922 ) ) ;
#9785=EDGE_CURVE ( 'NONE', #1485, #7672, #7641, .T. ) ;
#9786=EDGE_LOOP ( 'NONE', ( #2499, #4269, #1449, #5215 ) ) ;
#9787=CARTESIAN_POINT ( 'NONE',  ( -22.05573893622344173, 99.50000000000000000, -9.391591294897233766 ) ) ;
#9788=CARTESIAN_POINT ( 'NONE',  ( 3.238942592553923472, 100.0000000000000142, -24.36085717291697250 ) ) ;
#9789=CARTESIAN_POINT ( 'NONE',  ( 9.431378708427812896, 99.49999999999998579, 21.34379071326255684 ) ) ;
#9790=CARTESIAN_POINT ( 'NONE',  ( -21.29537297865864431, 100.0000000000000000, -11.39144590536739976 ) ) ;
#9791=CARTESIAN_POINT ( 'NONE',  ( 19.09188309203678102, 4.700000000000000178, 19.09188309203678813 ) ) ;
#9792=FACE_OUTER_BOUND ( 'NONE', #9635, .T. ) ;
#9793=CARTESIAN_POINT ( 'NONE',  ( -22.08823018108446234, 99.50000000000000000, -9.406177930363766038 ) ) ;
#9795=CARTESIAN_POINT ( 'NONE',  ( 8.187169943530866689, 99.99999999999998579, 20.27434297626003712 ) ) ;
#9797=VERTEX_POINT ( 'NONE', #8488 ) ;
#9803=DIRECTION ( 'NONE',  ( 0.9789429660840185399, 0.000000000000000000, -0.2041339490496966447 ) ) ;
#9804=CARTESIAN_POINT ( 'NONE',  ( 21.79306891025641235, 100.0000000000000000, -1.065004006410256387 ) ) ;
#9805=CARTESIAN_POINT ( 'NONE',  ( 9.248677610544923766, 99.50000000000000000, 22.83089001807756446 ) ) ;
#9807=LINE ( 'NONE', #930, #6621 ) ;
#9812=CARTESIAN_POINT ( 'NONE',  ( 4.446585460023182890, 99.50000000000002842, -21.79057454014859019 ) ) ;
#9813=CARTESIAN_POINT ( 'NONE',  ( 1.679787559701184688E-15, 5.249999998907525445, -27.43301270000000258 ) ) ;
#9815=AXIS2_PLACEMENT_3D ( 'NONE', #4762, #52, #7266 ) ;
#9816=CARTESIAN_POINT ( 'NONE',  ( 8.685676809262872666, 100.0000000000000000, 23.43455588346217766 ) ) ;
#9817=CARTESIAN_POINT ( 'NONE',  ( 3.739209042966564311, 99.99999999999998579, -21.42288334414699591 ) ) ;
#9818=CARTESIAN_POINT ( 'NONE',  ( 3.105863891863242632, 99.50000000000001421, -22.59672720503480292 ) ) ;
#9819=CARTESIAN_POINT ( 'NONE',  ( -27.00000000000000355, 4.949999997815051067, -11.18376618407357093 ) ) ;
#9821=CARTESIAN_POINT ( 'NONE',  ( -21.73488407773357167, 100.0000000000000000, -9.647150398373231184 ) ) ;
#9823=LINE ( 'NONE', #1862, #8952 ) ;
#9825=CARTESIAN_POINT ( 'NONE',  ( 4.803433990161294354, 99.50000000000001421, -23.96838578116891583 ) ) ;
#9827=EDGE_LOOP ( 'NONE', ( #2907, #1666, #2376, #3595 ) ) ;
#9828=ADVANCED_FACE ( 'NONE', ( #5179, #9381 ), #3675, .F. ) ;
#9831=CARTESIAN_POINT ( 'NONE',  ( -14.76042637754942177, 99.50000000000000000, 16.05242888258284140 ) ) ;
#9832=CARTESIAN_POINT ( 'NONE',  ( 3.016803124593948393, 99.50000000000001421, -23.20507807535735978 ) ) ;
#9833=CARTESIAN_POINT ( 'NONE',  ( 19.39806930854667399, 2.549999998907525267, 19.39806930854668465 ) ) ;
#9835=CARTESIAN_POINT ( 'NONE',  ( -20.71654887124055122, 100.0000000000000142, -9.874326132881018125 ) ) ;
#9836=DIRECTION ( 'NONE',  ( -0.000000000000000000, -1.000000000000000000, -0.000000000000000000 ) ) ;
#9837=LINE ( 'NONE', #2884, #8580 ) ;
#9838=VERTEX_POINT ( 'NONE', #7587 ) ;
#9839=CARTESIAN_POINT ( 'NONE',  ( -21.79396932678589849, 99.50000000000000000, -9.306975108219608828 ) ) ;
#9840=CARTESIAN_POINT ( 'NONE',  ( -27.43301270000000258, 4.649999998907525800, -3.359575119402369376E-15 ) ) ;
#9841=CARTESIAN_POINT ( 'NONE',  ( -15.84348323231452049, 99.50000000000000000, 15.18005498687102772 ) ) ;
#9842=CARTESIAN_POINT ( 'NONE',  ( 0.000000000000000000, 0.000000000000000000, 0.000000000000000000 ) ) ;
#9843=CARTESIAN_POINT ( 'NONE',  ( 4.320351800798612807, 99.99999999999995737, -21.62386382141117736 ) ) ;
#9844=CARTESIAN_POINT ( 'NONE',  ( -22.13144646319157260, 99.50000000000001421, -9.428651666388001118 ) ) ;
#9845=CARTESIAN_POINT ( 'NONE',  ( 3.659868213429061878, 99.50000000000000000, -22.50687739797974274 ) ) ;
#9846=CARTESIAN_POINT ( 'NONE',  ( -21.18972881998075763, 99.99999999999998579, -9.781869222470191971 ) ) ;
#9849=ORIENTED_EDGE ( 'NONE', *, *, #2683, .T. ) ;
#9851=EDGE_CURVE ( 'NONE', #1699, #10071, #3556, .T. ) ;
#9853=CARTESIAN_POINT ( 'NONE',  ( 3.204253864046738176, 99.50000000000000000, -22.06071064728738662 ) ) ;
#9854=CARTESIAN_POINT ( 'NONE',  ( 3.504547665631520648, 99.49999999999997158, -23.10026541809159184 ) ) ;
#9856=CARTESIAN_POINT ( 'NONE',  ( 4.331079892889020400, 99.50000000000000000, -24.67336562508343079 ) ) ;
#9857=CARTESIAN_POINT ( 'NONE',  ( 8.399337394135656609, 99.49999999999998579, 20.06291166101774692 ) ) ;
#9859=CARTESIAN_POINT ( 'NONE',  ( 5.725936192474917696, 99.50000000000000000, 21.08018326417248645 ) ) ;
#9860=CARTESIAN_POINT ( 'NONE',  ( 4.486604876299897349, 99.50000000000000000, -21.85617661337775885 ) ) ;
#9861=CARTESIAN_POINT ( 'NONE',  ( 9.431378708427812896, 99.99999999999998579, 21.34379071326255684 ) ) ;
#9864=CARTESIAN_POINT ( 'NONE',  ( 11.36312591709336850, 3.399999998907525356, 27.43301269999999903 ) ) ;
#9866=CARTESIAN_POINT ( 'NONE',  ( 3.973150561375555334, 99.99999999999997158, -22.87236500961342855 ) ) ;
#9867=CARTESIAN_POINT ( 'NONE',  ( 7.729958523985794194, 99.99999999999995737, 20.63140804260154937 ) ) ;
#9869=CARTESIAN_POINT ( 'NONE',  ( 9.861577898019769250, 99.49999999999995737, 21.03794551367759169 ) ) ;
#9870=CARTESIAN_POINT ( 'NONE',  ( -27.00000000000001421, 4.249999997815050001, 11.18376618407356382 ) ) ;
#9874=CARTESIAN_POINT ( 'NONE',  ( 2.901827748664965068, 99.99999999999998579, -21.68759887446373469 ) ) ;
#9875=DIRECTION ( 'NONE',  ( -0.1966827481675937905, 0.000000000000000000, -0.9804671828129909450 ) ) ;
#9877=FACE_BOUND ( 'NONE', #2942, .T. ) ;
#9879=CARTESIAN_POINT ( 'NONE',  ( 11.36312591709336850, 3.299999998907525711, 27.43301269999999903 ) ) ;
#9880=CARTESIAN_POINT ( 'NONE',  ( -11.36312591709335962, 0.5999999989075250895, -27.43301270000000258 ) ) ;
#9882=AXIS2_PLACEMENT_3D ( 'NONE', #6103, #6831, #8463 ) ;
#9884=CARTESIAN_POINT ( 'NONE',  ( -20.63666786535793207, 99.99999999999998579, -10.16306733409737717 ) ) ;
#9885=PLANE ( 'NONE',  #5662 ) ;
#9886=DIRECTION ( 'NONE',  ( 0.000000000000000000, 1.000000000000000000, 0.000000000000000000 ) ) ;
#9887=ORIENTED_EDGE ( 'NONE', *, *, #10251, .F. ) ;
#9888=CARTESIAN_POINT ( 'NONE',  ( -21.99154324187120579, 99.99999999999994316, -9.362771248264911250 ) ) ;
#9890=CARTESIAN_POINT ( 'NONE',  ( 3.097283534322414766, 100.0000000000000284, -24.18405864774921454 ) ) ;
#9891=CARTESIAN_POINT ( 'NONE',  ( -15.49723655759404295, 99.49999999999997158, 15.26389171799780264 ) ) ;
#9892=VECTOR ( 'NONE', #5301, 1000.000000000000000 ) ;
#9894=CARTESIAN_POINT ( 'NONE',  ( 4.187832255138415505, 100.0000000000000142, -21.50835573230103037 ) ) ;
#9895=CARTESIAN_POINT ( 'NONE',  ( 9.513000527211589841, 99.50000000000000000, 20.35102222961602436 ) ) ;
#9896=CARTESIAN_POINT ( 'NONE',  ( 9.358681735871565266, 99.99999999999992895, 21.55373624431538815 ) ) ;
#9897=CARTESIAN_POINT ( 'NONE',  ( -21.00001322343447541, 100.0000000000000142, -9.990026185521596602 ) ) ;
#9898=ORIENTED_EDGE ( 'NONE', *, *, #6559, .T. ) ;
#9899=EDGE_CURVE ( 'NONE', #7937, #6736, #2889, .T. ) ;
#9901=VECTOR ( 'NONE', #10103, 1000.000000000000000 ) ;
#9904=CARTESIAN_POINT ( 'NONE',  ( -4.959819536546781389E-15, 4.599999999999999645, 27.00000000000000355 ) ) ;
#9905=CARTESIAN_POINT ( 'NONE',  ( 3.202955020264580899, 99.50000000000000000, -21.91595956354277064 ) ) ;
#9906=CARTESIAN_POINT ( 'NONE',  ( -19.09188309203678457, 4.899999997815050357, -19.09188309203678813 ) ) ;
#9911=EDGE_LOOP ( 'NONE', ( #2166, #4671, #9284, #4401 ) ) ;
#9912=CARTESIAN_POINT ( 'NONE',  ( -27.00000000000000355, 2.750000000000000888, -11.18376618407357270 ) ) ;
#9913=DIRECTION ( 'NONE',  ( -0.000000000000000000, 1.000000000000000000, -0.000000000000000000 ) ) ;
#9914=CARTESIAN_POINT ( 'NONE',  ( -22.20893716642541804, 100.0000000000000284, -10.81429252070940272 ) ) ;
#9915=CARTESIAN_POINT ( 'NONE',  ( 3.282077632710153292, 99.50000000000000000, -23.74569985055724786 ) ) ;
#9916=( BOUNDED_CURVE ( )  B_SPLINE_CURVE ( 2, ( #3275, #9117, #9015, #10006, #430, #1988, #485, #3569, #8437 ),
 .UNSPECIFIED., .F., .T. ) 
 B_SPLINE_CURVE_WITH_KNOTS ( ( 3, 2, 2, 2, 3 ),
 ( 0.3928571428571428492, 0.4107142857142856984, 0.4285714285714285476, 0.4464285714285714524, 0.4642857142857143016 ),
 .UNSPECIFIED. ) 
 CURVE ( )  GEOMETRIC_REPRESENTATION_ITEM ( )  RATIONAL_B_SPLINE_CURVE ( ( 1.000000000000000000, 0.9238795325112867385, 1.000000000000000000, 0.9238795325112867385, 1.000000000000000000, 0.9238795325112867385, 1.000000000000000000, 0.9238795325112867385, 1.000000000000000000 ) ) 
 REPRESENTATION_ITEM ( '' )  );
#9917=ORIENTED_EDGE ( 'NONE', *, *, #1615, .F. ) ;
#9918=CARTESIAN_POINT ( 'NONE',  ( -20.72805389903318130, 99.50000000000000000, -9.848585782927868237 ) ) ;
#9919=CARTESIAN_POINT ( 'NONE',  ( -11.36312591709337383, 4.899999998907526688, 27.43301269999999548 ) ) ;
#9921=CARTESIAN_POINT ( 'NONE',  ( 2.940631318607589417, 99.50000000000000000, -23.77584808773673331 ) ) ;
#9922=CARTESIAN_POINT ( 'NONE',  ( 8.133363296361027395, 99.99999999999998579, 19.85287606700953233 ) ) ;
#9923=ORIENTED_EDGE ( 'NONE', *, *, #2961, .F. ) ;
#9925=CARTESIAN_POINT ( 'NONE',  ( -27.00000000000000355, 4.999999997815050889, -3.306546357697854128E-15 ) ) ;
#9931=B_SPLINE_CURVE_WITH_KNOTS ( 'NONE', 3,
 ( #2729, #5866, #1985, #9789, #6649, #1879, #5073, #6552, #3566, #1004, #2782, #2626, #9112, #3405, #1932 ),
 .UNSPECIFIED., .F., .F.,
 ( 4, 1, 1, 1, 1, 1, 1, 1, 1, 1, 1, 1, 4 ),
 ( 0.000000000000000000, 0.1101401978779246588, 0.2116695470404897084, 0.3047824012491699430, 0.3893374185178356539, 0.4648567744508144695, 0.5325800579573772842, 0.5913915682020929321, 0.6424829260185016544, 0.7344861914544180692, 0.8232371011010507500, 0.9113455750355911045, 1.000000000000000000 ),
 .UNSPECIFIED. ) ;
#9934=ORIENTED_EDGE ( 'NONE', *, *, #6148, .F. ) ;
#9937=FACE_OUTER_BOUND ( 'NONE', #563, .T. ) ;
#9938=CARTESIAN_POINT ( 'NONE',  ( 2.927917759182871560, 99.49999999999997158, -23.69257214368879261 ) ) ;
#9939=CARTESIAN_POINT ( 'NONE',  ( 27.43301270000000258, 1.899999998907525134, -11.36312591709336139 ) ) ;
#9942=CYLINDRICAL_SURFACE ( 'NONE', #4610, 25.15000000000000213 ) ;
#9944=CARTESIAN_POINT ( 'NONE',  ( -27.00000000000000355, 4.149999997815050357, -11.18376618407357270 ) ) ;
#9946=CARTESIAN_POINT ( 'NONE',  ( 7.746148141271532950, 99.50000000000002842, 20.51930889200067298 ) ) ;
#9947=FACE_OUTER_BOUND ( 'NONE', #6809, .T. ) ;
#9950=CARTESIAN_POINT ( 'NONE',  ( -19.39806930854667755, 0.5499999989075252671, -19.39806930854668110 ) ) ;
#9951=ADVANCED_FACE ( 'NONE', ( #886 ), #1805, .T. ) ;
#9953=CARTESIAN_POINT ( 'NONE',  ( 9.358681735871565266, 99.49999999999998579, 21.55373624431538815 ) ) ;
#9956=CARTESIAN_POINT ( 'NONE',  ( -15.98323291606820362, 99.49999999999998579, 16.64087298452848884 ) ) ;
#9959=CARTESIAN_POINT ( 'NONE',  ( -21.96365545856212265, 99.99999999999998579, -9.726658277667754149 ) ) ;
#9960=CARTESIAN_POINT ( 'NONE',  ( -16.63177974700816009, 99.50000000000000000, 16.59747536361813403 ) ) ;
#9962=CARTESIAN_POINT ( 'NONE',  ( 3.973150561375555334, 99.50000000000000000, -22.87236500961342855 ) ) ;
#9964=VERTEX_POINT ( 'NONE', #2510 ) ;
#9965=CARTESIAN_POINT ( 'NONE',  ( -16.37951318544778445, 99.49999999999997158, 15.41600550949200077 ) ) ;
#9966=CIRCLE ( 'NONE', #9477, 7.500000000000000000 ) ;
#9967=CARTESIAN_POINT ( 'NONE',  ( 3.207057600658871355, 99.50000000000000000, -22.07913334414698880 ) ) ;
#9968=EDGE_CURVE ( 'NONE', #969, #10097, #255, .T. ) ;
#9969=CARTESIAN_POINT ( 'NONE',  ( -16.91946509138130139, 100.0000000000000142, 15.98858002463268413 ) ) ;
#9970=CARTESIAN_POINT ( 'NONE',  ( 3.478562133589548910, 99.49999999999997158, -24.13114810667639532 ) ) ;
#9971=ORIENTED_EDGE ( 'NONE', *, *, #2318, .F. ) ;
#9973=CARTESIAN_POINT ( 'NONE',  ( -19.39806930854667755, 3.849999998907525089, -19.39806930854668110 ) ) ;
#9974=DIRECTION ( 'NONE',  ( -0.000000000000000000, 1.000000000000000000, -0.000000000000000000 ) ) ;
#9975=CARTESIAN_POINT ( 'NONE',  ( 9.910564025336874749, 100.0000000000000000, 20.75459158945058036 ) ) ;
#9978=CARTESIAN_POINT ( 'NONE',  ( 9.834295043520187463, 99.50000000000002842, 21.14079655679390513 ) ) ;
#9979=CARTESIAN_POINT ( 'NONE',  ( 11.18376618407357626, 4.449999997815051067, 27.00000000000000000 ) ) ;
#9980=CARTESIAN_POINT ( 'NONE',  ( 27.00000000000000355, 3.250000000000000444, -11.18376618407356915 ) ) ;
#9985=CARTESIAN_POINT ( 'NONE',  ( 4.829054701479813083, 100.0000000000000000, -23.91032069601275367 ) ) ;
#9986=CARTESIAN_POINT ( 'NONE',  ( -19.39806930854667755, 1.449999998907525178, -19.39806930854668110 ) ) ;
#9988=ADVANCED_FACE ( 'NONE', ( #5701 ), #8516, .T. ) ;
#9992=CARTESIAN_POINT ( 'NONE',  ( -11.36312591709337383, 2.399999998907525356, 27.43301269999999548 ) ) ;
#9993=LINE ( 'NONE', #415, #4541 ) ;
#9995=CARTESIAN_POINT ( 'NONE',  ( -16.60513711880302878, 100.0000000000000000, 15.15667007515659570 ) ) ;
#9996=VECTOR ( 'NONE', #6746, 1000.000000000000000 ) ;
#9998=CARTESIAN_POINT ( 'NONE',  ( 7.753999887479250397, 100.0000000000000000, 20.97676509141502166 ) ) ;
#9999=CARTESIAN_POINT ( 'NONE',  ( 3.597125852879613728, 99.99999999999998579, -24.22990373345680126 ) ) ;
#10000=DIRECTION ( 'NONE',  ( 0.2499845035238856816, 0.000000000000000000, -0.9682498375925071565 ) ) ;
#10001=EDGE_LOOP ( 'NONE', ( #8705, #1215, #9421, #4317 ) ) ;
#10003=CARTESIAN_POINT ( 'NONE',  ( -11.36312591709337383, 2.399999998907525356, 27.43301269999999548 ) ) ;
#10004=CARTESIAN_POINT ( 'NONE',  ( -16.56926954694585774, 99.50000000000001421, 15.12296757606276643 ) ) ;
#10005=CARTESIAN_POINT ( 'NONE',  ( 3.212364564527730337, 99.50000000000000000, -22.10366694310577884 ) ) ;
#10006=CARTESIAN_POINT ( 'NONE',  ( 26.99999999999999645, 2.350000000000000533, 11.18376618407358691 ) ) ;
#10008=DIRECTION ( 'NONE',  ( -0.000000000000000000, -1.000000000000000000, -0.000000000000000000 ) ) ;
#10010=ORIENTED_EDGE ( 'NONE', *, *, #8691, .F. ) ;
#10012=DIRECTION ( 'NONE',  ( -0.000000000000000000, 1.000000000000000000, -0.000000000000000000 ) ) ;
#10014=CARTESIAN_POINT ( 'NONE',  ( 2.924645347134957163, 100.0000000000000142, -23.60918035669702064 ) ) ;
#10015=ORIENTED_EDGE ( 'NONE', *, *, #8659, .F. ) ;
#10016=EDGE_CURVE ( 'NONE', #1992, #5243, #5838, .T. ) ;
#10017=CARTESIAN_POINT ( 'NONE',  ( 4.200543313440712190, 99.50000000000000000, -21.13206004899810608 ) ) ;
#10019=DIRECTION ( 'NONE',  ( 0.05468478504300072762, 0.000000000000000000, 0.9985036676371302766 ) ) ;
#10022=CARTESIAN_POINT ( 'NONE',  ( 19.39806930854668110, 3.649999998907525356, -19.39806930854668110 ) ) ;
#10024=CARTESIAN_POINT ( 'NONE',  ( 9.902568905804752575, 99.49999999999998579, 20.48863403721516363 ) ) ;
#10026=CARTESIAN_POINT ( 'NONE',  ( 1.670949432750432147E-15, 5.433333331876700534, -27.28867513333333505 ) ) ;
#10027=VECTOR ( 'NONE', #6888, 1000.000000000000000 ) ;
#10028=CARTESIAN_POINT ( 'NONE',  ( 4.988497440555089923, 99.50000000000000000, -24.29977663856455194 ) ) ;
#10030=CYLINDRICAL_SURFACE ( 'NONE', #8003, 7.500000000000000000 ) ;
#10033=CARTESIAN_POINT ( 'NONE',  ( 1.679787559701184688E-15, 2.149999998907525356, -27.43301270000000258 ) ) ;
#10035=B_SPLINE_CURVE_WITH_KNOTS ( 'NONE', 3,
 ( #4309, #7494, #5929, #4260, #1224, #4415, #1945, #7600, #9854, #1169, #333, #1841, #9176, #3689, #5832, #9962, #4467, #8236, #9024 ),
 .UNSPECIFIED., .F., .F.,
 ( 4, 1, 1, 1, 1, 1, 1, 1, 1, 1, 1, 1, 1, 1, 1, 1, 4 ),
 ( 0.000000000000000000, 0.07039602572822099835, 0.1400447079551435658, 0.2099027554305550880, 0.2826152692239142783, 0.3556467613428230812, 0.4271065942619623468, 0.4986634349892335449, 0.5720141774457471184, 0.6112909118483191850, 0.6543288624652392471, 0.7009162800881839628, 0.7518538071550001645, 0.8072437197097745987, 0.8671654997918389896, 0.9315515937071113806, 1.000000000000000000 ),
 .UNSPECIFIED. ) ;
#10038=CARTESIAN_POINT ( 'NONE',  ( 3.551917533706515417, 99.99999999999998579, -21.11785906961830150 ) ) ;
#10040=ADVANCED_FACE ( 'NONE', ( #9032 ), #1849, .F. ) ;
#10041=CARTESIAN_POINT ( 'NONE',  ( 27.43301270000000258, 5.049999998907525267, 0.000000000000000000 ) ) ;
#10042=CARTESIAN_POINT ( 'NONE',  ( 11.36312591709336850, 0.9999999989075254447, 27.43301269999999903 ) ) ;
#10044=CARTESIAN_POINT ( 'NONE',  ( -16.18394139941567644, 100.0000000000000000, 16.57042731130403723 ) ) ;
#10046=CARTESIAN_POINT ( 'NONE',  ( 1.653273178848927064E-15, 3.999999997815050889, -27.00000000000000355 ) ) ;
#10047=CARTESIAN_POINT ( 'NONE',  ( -16.34436021381890924, 100.0000000000000000, 15.38072013554846151 ) ) ;
#10050=DIRECTION ( 'NONE',  ( -0.000000000000000000, 1.000000000000000000, -0.000000000000000000 ) ) ;
#10052=CARTESIAN_POINT ( 'NONE',  ( 0.000000000000000000, 97.50000000000000000, 0.000000000000000000 ) ) ;
#10053=CARTESIAN_POINT ( 'NONE',  ( -19.39806930854668465, 1.549999998907525267, 19.39806930854667755 ) ) ;
#10058=CARTESIAN_POINT ( 'NONE',  ( 9.526713201929464248, 99.50000000000000000, 20.38668308130821671 ) ) ;
#10059=FACE_OUTER_BOUND ( 'NONE', #10328, .T. ) ;
#10064=EDGE_LOOP ( 'NONE', ( #2078, #2842, #7645, #3842, #5796, #2046, #8415, #8103 ) ) ;
#10065=CARTESIAN_POINT ( 'NONE',  ( -21.94169572595625795, 99.99999999999997158, -9.715372641902229489 ) ) ;
#10071=VERTEX_POINT ( 'NONE', #395 ) ;
#10074=DIRECTION ( 'NONE',  ( 0.000000000000000000, 0.000000000000000000, -1.000000000000000000 ) ) ;
#10077=VECTOR ( 'NONE', #8247, 1000.000000000000000 ) ;
#10078=CARTESIAN_POINT ( 'NONE',  ( 1.679787559701184688E-15, 2.949999998907525178, -27.43301270000000258 ) ) ;
#10083=CARTESIAN_POINT ( 'NONE',  ( -21.30033281797529909, 100.0000000000000284, -9.345151174687854834 ) ) ;
#10087=ORIENTED_EDGE ( 'NONE', *, *, #5646, .F. ) ;
#10088=CARTESIAN_POINT ( 'NONE',  ( -15.69732130854469432, 99.50000000000001421, 15.19348709373450035 ) ) ;
#10089=CARTESIAN_POINT ( 'NONE',  ( -27.43301270000000258, 2.299999998907525267, -11.36312591709336317 ) ) ;
#10090=VERTEX_POINT ( 'NONE', #5201 ) ;
#10092=CARTESIAN_POINT ( 'NONE',  ( -16.56928979259283352, 100.0000000000000284, 16.65656195153832897 ) ) ;
#10095=CARTESIAN_POINT ( 'NONE',  ( 3.306546357697854128E-15, 100.0000000000000000, 27.00000000000000355 ) ) ;
#10096=CARTESIAN_POINT ( 'NONE',  ( 27.43301269999999548, 1.899999998907525356, 11.36312591709337738 ) ) ;
#10097=VERTEX_POINT ( 'NONE', #7610 ) ;
#10098=UNCERTAINTY_MEASURE_WITH_UNIT (LENGTH_MEASURE( 1.000000000000000082E-05 ), #1933, 'distance_accuracy_value', 'NONE');
#10100=EDGE_CURVE ( 'NONE', #7488, #3916, #5096, .T. ) ;
#10101=VECTOR ( 'NONE', #4675, 1000.000000000000000 ) ;
#10102=CARTESIAN_POINT ( 'NONE',  ( 4.143207896384923039, 99.99999999999998579, -24.36264353342416911 ) ) ;
#10103=DIRECTION ( 'NONE',  ( -0.8547548816071318667, 0.000000000000000000, 0.5190318799156541374 ) ) ;
#10109=ORIENTED_EDGE ( 'NONE', *, *, #4349, .F. ) ;
#10110=ADVANCED_FACE ( 'NONE', ( #5150 ), #3589, .T. ) ;
#10112=CARTESIAN_POINT ( 'NONE',  ( -11.36312591709335962, 3.699999998907525622, -27.43301270000000258 ) ) ;
#10115=CARTESIAN_POINT ( 'NONE',  ( -11.18376618407356560, 1.849999999999999867, -27.00000000000000355 ) ) ;
#10116=DIRECTION ( 'NONE',  ( -0.000000000000000000, -1.000000000000000000, -0.000000000000000000 ) ) ;
#10120=CARTESIAN_POINT ( 'NONE',  ( 8.064245308217579122, 99.49999999999998579, 20.64099956338070641 ) ) ;
#10122=VERTEX_POINT ( 'NONE', #6774 ) ;
#10123=CARTESIAN_POINT ( 'NONE',  ( 4.386516977709190357, 99.50000000000004263, -24.31220192127581825 ) ) ;
#10124=CARTESIAN_POINT ( 'NONE',  ( -19.39806930854667755, 0.5499999989075252671, -19.39806930854668110 ) ) ;
#10125=CARTESIAN_POINT ( 'NONE',  ( -21.80427673524616239, 99.50000000000000000, -9.663674634844889866 ) ) ;
#10127=EDGE_CURVE ( 'NONE', #3209, #6813, #9419, .T. ) ;
#10133=DIRECTION ( 'NONE',  ( -0.000000000000000000, 1.000000000000000000, -0.000000000000000000 ) ) ;
#10135=DIRECTION ( 'NONE',  ( -0.000000000000000000, -1.000000000000000000, -0.000000000000000000 ) ) ;
#10136=ORIENTED_EDGE ( 'NONE', *, *, #5142, .T. ) ;
#10137=CARTESIAN_POINT ( 'NONE',  ( -21.98271324694694329, 100.0000000000000000, -11.39207625356720222 ) ) ;
#10140=CARTESIAN_POINT ( 'NONE',  ( 9.723125805078051798, 99.99999999999998579, 21.50134635983626907 ) ) ;
#10141=ORIENTED_EDGE ( 'NONE', *, *, #4254, .T. ) ;
#10144=CARTESIAN_POINT ( 'NONE',  ( 8.644881627383616873, 99.99999999999995737, 19.60534525227960145 ) ) ;
#10147=CARTESIAN_POINT ( 'NONE',  ( -21.30928386698190025, 100.0000000000000000, -11.02857376369709996 ) ) ;
#10154=VECTOR ( 'NONE', #8980, 1000.000000000000000 ) ;
#10157=LINE ( 'NONE', #7849, #1433 ) ;
#10159=CARTESIAN_POINT ( 'NONE',  ( -16.76168403648438243, 99.50000000000002842, 16.44483764528499847 ) ) ;
#10160=CARTESIAN_POINT ( 'NONE',  ( 27.43301269999999548, 2.699999998907525178, 11.36312591709337738 ) ) ;
#10161=CARTESIAN_POINT ( 'NONE',  ( 8.465276868207817884, 100.0000000000000142, 19.66343818277063704 ) ) ;
#10163=DIRECTION ( 'NONE',  ( -0.9851965920526258857, 0.000000000000000000, -0.1714283378204774222 ) ) ;
#10164=CARTESIAN_POINT ( 'NONE',  ( 3.681717055787076642, 99.50000000000000000, -21.09125273517263111 ) ) ;
#10166=CARTESIAN_POINT ( 'NONE',  ( -15.69732130854469432, 100.0000000000000142, 15.19348709373450035 ) ) ;
#10171=CARTESIAN_POINT ( 'NONE',  ( 11.36312591709336139, 1.199999998907525178, -27.43301270000000258 ) ) ;
#10173=ORIENTED_EDGE ( 'NONE', *, *, #2174, .T. ) ;
#10174=LINE ( 'NONE', #2892, #3932 ) ;
#10175=CARTESIAN_POINT ( 'NONE',  ( 19.09188309203678102, 2.299999999999999822, 19.09188309203678813 ) ) ;
#10176=CARTESIAN_POINT ( 'NONE',  ( 0.000000000000000000, 100.0000000000000000, 0.000000000000000000 ) ) ;
#10178=CARTESIAN_POINT ( 'NONE',  ( -16.54512803120131181, 99.99999999999995737, 16.13427955854364626 ) ) ;
#10184=VECTOR ( 'NONE', #7843, 999.9999999999998863 ) ;
#10188=CARTESIAN_POINT ( 'NONE',  ( 2.927917759182871560, 99.99999999999997158, -23.69257214368879261 ) ) ;
#10190=EDGE_CURVE ( 'NONE', #8208, #7672, #7721, .T. ) ;
#10191=B_SPLINE_CURVE_WITH_KNOTS ( 'NONE', 3,
 ( #3300, #4763, #9680, #1241, #9042, #5899, #1136, #4329, #6835, #2817, #250, #2012, #1860, #8358, #2657, #1189, #5847, #9095, #6000 ),
 .UNSPECIFIED., .F., .F.,
 ( 4, 1, 1, 1, 1, 1, 1, 1, 1, 1, 1, 1, 1, 1, 1, 1, 4 ),
 ( 0.000000000000000000, 0.07039602572822099835, 0.1400447079551435658, 0.2099027554305550880, 0.2826152692239142783, 0.3556467613428230812, 0.4271065942619623468, 0.4986634349892335449, 0.5720141774457471184, 0.6112909118483191850, 0.6543288624652392471, 0.7009162800881839628, 0.7518538071550001645, 0.8072437197097745987, 0.8671654997918389896, 0.9315515937071113806, 1.000000000000000000 ),
 .UNSPECIFIED. ) ;
#10192=EDGE_CURVE ( 'NONE', #9616, #717, #7667, .T. ) ;
#10194=EDGE_LOOP ( 'NONE', ( #3304, #6890, #5332, #3806 ) ) ;
#10196=CARTESIAN_POINT ( 'NONE',  ( 27.00000000000000355, 0.8500000000000001998, -11.18376618407356915 ) ) ;
#10200=B_SPLINE_SURFACE_WITH_KNOTS ( 'NONE', 3, 1, ( 
 ( #9071, #1990 ),
 ( #9120, #1886 ),
 ( #5135, #6758 ),
 ( #7651, #5080 ),
 ( #378, #488 ),
 ( #6865, #2736 ),
 ( #6083, #1216 ),
 ( #9956, #2789 ),
 ( #9273, #1111 ),
 ( #4303, #8387 ),
 ( #6355, #3065 ),
 ( #2219, #3015 ),
 ( #9548, #3895 ),
 ( #2326, #9447 ),
 ( #5572, #6192 ),
 ( #2956, #8715 ),
 ( #9390, #7870 ),
 ( #1379, #2374 ),
 ( #7767, #5523 ) ),
 .UNSPECIFIED., .F., .F., .F.,
 ( 4, 1, 1, 1, 1, 1, 1, 1, 1, 1, 1, 1, 1, 1, 1, 1, 4 ),
 ( 2, 2 ),
 ( 0.000000000000000000, 0.06473117683888822416, 0.1283191082976379849, 0.1900130092022370987, 0.2509653124206144836, 0.3118694605430146760, 0.3735603890354366463, 0.4359106579620777855, 0.5007804971236301528, 0.5656503362851855732, 0.6280858374182423098, 0.6899222460797727052, 0.7510277903999277305, 0.8114330998898260372, 0.8726106248506092511, 0.9357151229638154266, 1.000000000000000000 ),
 ( 0.000000000000000000, 1.000000000000000000 ),
 .UNSPECIFIED. ) ;
#10202=CARTESIAN_POINT ( 'NONE',  ( 9.445361748092775400, 99.50000000000001421, 19.75398588445988324 ) ) ;
#10203=FACE_BOUND ( 'NONE', #745, .T. ) ;
#10204=EDGE_LOOP ( 'NONE', ( #6795, #585, #10230, #5353 ) ) ;
#10205=CARTESIAN_POINT ( 'NONE',  ( -15.84348323231452049, 99.50000000000000000, 15.18005498687102772 ) ) ;
#10206=CARTESIAN_POINT ( 'NONE',  ( 19.39806930854668110, 1.249999998907525223, -19.39806930854668110 ) ) ;
#10209=DIRECTION ( 'NONE',  ( 0.000000000000000000, 0.000000000000000000, -1.000000000000000000 ) ) ;
#10210=( BOUNDED_CURVE ( )  B_SPLINE_CURVE ( 2, ( #6762, #8502, #3742, #2963, #6924, #6817, #10124, #6142, #601, #2795, #9340, #2170, #5982, #3798, #5193, #8392, #4414, #6408, #3174, #4782, #9648, #2380, #2330, #4053, #7035, #5577, #1537, #7189, #7236, #9552, #9452, #5677, #1491, #9598, #4687, #8720, #6254, #6460, #2429, #2484, #7137, #8765, #4733, #7086, #7873, #706, #3899, #5625, #8865, #1590, #1691, #9505, #7927, #18, #3953, #10291, #3124, #6309, #1644, #4887, #8815, #7978, #759, #8082, #10342, #5527, #3848, #811, #6358, #5477, #10237, #2281, #4836, #8669, #8030, #863, #4005, #3219, #3070, #75, #3267, #4152, #7381, #2534, #6648, #2673, #3404, #9061, #9840, #5772, #8274, #3315, #4296, #3508, #128, #1054, #6694, #6504, #9694, #219, #5819 ),
 .UNSPECIFIED., .F., .T. ) 
 B_SPLINE_CURVE_WITH_KNOTS ( ( 3, 2, 2, 2, 2, 2, 2, 2, 2, 2, 2, 2, 2, 2, 2, 2, 2, 2, 2, 2, 2, 2, 2, 2, 2, 2, 2, 2, 2, 2, 2, 2, 2, 2, 2, 2, 2, 2, 2, 2, 2, 2, 2, 2, 2, 2, 2, 2, 2, 2, 3 ),
 ( 0.000000000000000000, 0.01785714285714285615, 0.03571428571428571230, 0.05357142857142856845, 0.07142857142857142461, 0.08928571428571428770, 0.1071428571428571369, 0.1250000000000000000, 0.1428571428571428492, 0.1607142857142857262, 0.1785714285714285754, 0.1964285714285714246, 0.2142857142857142738, 0.2321428571428571508, 0.2500000000000000000, 0.2678571428571428492, 0.2857142857142856984, 0.3035714285714285476, 0.3214285714285714524, 0.3392857142857143016, 0.3571428571428571508, 0.3750000000000000000, 0.3928571428571428492, 0.4107142857142856984, 0.4285714285714285476, 0.4464285714285714524, 0.4642857142857143016, 0.4821428571428571508, 0.5000000000000000000, 0.5178571428571429047, 0.5357142857142856984, 0.5535714285714286031, 0.5714285714285713969, 0.5892857142857143016, 0.6071428571428570953, 0.6250000000000000000, 0.6428571428571429047, 0.6607142857142856984, 0.6785714285714286031, 0.6964285714285715079, 0.7142857142857143016, 0.7321428571428570953, 0.7500000000000000000, 0.7678571428571429047, 0.7857142857142856984, 0.8035714285714286031, 0.8214285714285713969, 0.8392857142857143016, 0.8571428571428570953, 0.8750000000000000000, 0.8928571428571429047 ),
 .UNSPECIFIED. ) 
 CURVE ( )  GEOMETRIC_REPRESENTATION_ITEM ( )  RATIONAL_B_SPLINE_CURVE ( ( 1.000000000000000000, 0.9238795325112867385, 1.000000000000000000, 0.9238795325112867385, 1.000000000000000000, 0.9238795325112867385, 1.000000000000000000, 0.9238795325112867385, 1.000000000000000000, 0.9238795325112867385, 1.000000000000000000, 0.9238795325112867385, 1.000000000000000000, 0.9238795325112867385, 1.000000000000000000, 0.9238795325112867385, 1.000000000000000000, 0.9238795325112867385, 1.000000000000000000, 0.9238795325112867385, 1.000000000000000000, 0.9238795325112867385, 1.000000000000000000, 0.9238795325112867385, 1.000000000000000000, 0.9238795325112867385, 1.000000000000000000, 0.9238795325112867385, 1.000000000000000000, 0.9238795325112867385, 1.000000000000000000, 0.9238795325112867385, 1.000000000000000000, 0.9238795325112867385, 1.000000000000000000, 0.9238795325112867385, 1.000000000000000000, 0.9238795325112867385, 1.000000000000000000, 0.9238795325112867385, 1.000000000000000000, 0.9238795325112867385, 1.000000000000000000, 0.9238795325112867385, 1.000000000000000000, 0.9238795325112867385, 1.000000000000000000, 0.9238795325112867385, 1.000000000000000000, 0.9238795325112867385, 1.000000000000000000, 0.9238795325112867385, 1.000000000000000000, 0.9238795325112867385, 1.000000000000000000, 0.9238795325112867385, 1.000000000000000000, 0.9238795325112867385, 1.000000000000000000, 0.9238795325112867385, 1.000000000000000000, 0.9238795325112867385, 1.000000000000000000, 0.9238795325112867385, 1.000000000000000000, 0.9238795325112867385, 1.000000000000000000, 0.9238795325112867385, 1.000000000000000000, 0.9238795325112867385, 1.000000000000000000, 0.9238795325112867385, 1.000000000000000000, 0.9238795325112867385, 1.000000000000000000, 0.9238795325112867385, 1.000000000000000000, 0.9238795325112867385, 1.000000000000000000, 0.9238795325112867385, 1.000000000000000000, 0.9238795325112867385, 1.000000000000000000, 0.9238795325112867385, 1.000000000000000000, 0.9238795325112867385, 1.000000000000000000, 0.9238795325112867385, 1.000000000000000000, 0.9238795325112867385, 1.000000000000000000, 0.9238795325112867385, 1.000000000000000000, 0.9238795325112867385, 1.000000000000000000, 0.9238795325112867385, 1.000000000000000000, 0.9238795325112867385, 1.000000000000000000, 0.9238795325112867385, 1.000000000000000000 ) ) 
 REPRESENTATION_ITEM ( '' )  );
#10212=CARTESIAN_POINT ( 'NONE',  ( -11.36312591709337383, 4.799999998907525267, 27.43301269999999548 ) ) ;
#10213=CARTESIAN_POINT ( 'NONE',  ( -27.43301270000000258, 2.299999998907525267, -11.36312591709336317 ) ) ;
#10216=CARTESIAN_POINT ( 'NONE',  ( -16.56926954694585774, 100.0000000000000142, 15.12296757606276643 ) ) ;
#10219=CARTESIAN_POINT ( 'NONE',  ( -15.34161522349497808, 99.99999999999998579, 15.37783959465231121 ) ) ;
#10222=CARTESIAN_POINT ( 'NONE',  ( 4.504418077186241653, 100.0000000000000426, -21.31258943653750393 ) ) ;
#10223=ORIENTED_EDGE ( 'NONE', *, *, #1907, .F. ) ;
#10225=CARTESIAN_POINT ( 'NONE',  ( -19.39806930854668465, 3.949999998907525178, 19.39806930854667755 ) ) ;
#10226=DIRECTION ( 'NONE',  ( 0.9853569121566161382, 0.000000000000000000, 0.1705044153832351028 ) ) ;
#10227=EDGE_CURVE ( 'NONE', #5876, #2327, #5321, .T. ) ;
#10228=CARTESIAN_POINT ( 'NONE',  ( -11.18376618407356560, 2.649999999999999911, -27.00000000000000355 ) ) ;
#10229=CARTESIAN_POINT ( 'NONE',  ( 8.901217755223779449, 99.50000000000004263, 19.92336871027421097 ) ) ;
#10230=ORIENTED_EDGE ( 'NONE', *, *, #10190, .T. ) ;
#10231=CARTESIAN_POINT ( 'NONE',  ( -27.00000000000001421, 2.850000000000000089, 11.18376618407356560 ) ) ;
#10232=CARTESIAN_POINT ( 'NONE',  ( -20.96643530928959365, 99.50000000000000000, -10.05541671241504886 ) ) ;
#10233=ORIENTED_EDGE ( 'NONE', *, *, #6559, .F. ) ;
#10236=ORIENTED_EDGE ( 'NONE', *, *, #1731, .T. ) ;
#10237=CARTESIAN_POINT ( 'NONE',  ( -19.39806930854667755, 3.749999998907525445, -19.39806930854668110 ) ) ;
#10238=VECTOR ( 'NONE', #6518, 1000.000000000000000 ) ;
#10241=CARTESIAN_POINT ( 'NONE',  ( 4.988497440555089923, 99.50000000000000000, -24.29977663856455194 ) ) ;
#10242=ADVANCED_FACE ( 'NONE', ( #2002 ), #3645, .T. ) ;
#10245=EDGE_CURVE ( 'NONE', #7989, #4244, #8818, .T. ) ;
#10248=CARTESIAN_POINT ( 'NONE',  ( 4.034460619503033030, 99.99999999999995737, -21.08676866017170681 ) ) ;
#10249=CARTESIAN_POINT ( 'NONE',  ( -22.08823018108446234, 99.50000000000000000, -9.406177930363766038 ) ) ;
#10250=EDGE_LOOP ( 'NONE', ( #4860, #9917, #4382, #8593 ) ) ;
#10251=EDGE_CURVE ( 'NONE', #358, #8208, #4387, .T. ) ;
#10252=CARTESIAN_POINT ( 'NONE',  ( 8.751508028230254865, 99.49999999999998579, 19.58480916780017722 ) ) ;
#10256=ORIENTED_EDGE ( 'NONE', *, *, #1716, .T. ) ;
#10258=CARTESIAN_POINT ( 'NONE',  ( 9.600410285814406919, 99.49999999999998579, 19.87914582625927196 ) ) ;
#10259=CARTESIAN_POINT ( 'NONE',  ( 24.93339342948717885, 100.0000000000000000, -1.235376602564102644 ) ) ;
#10261=CARTESIAN_POINT ( 'NONE',  ( -15.69732130854469432, 100.0000000000000142, 15.19348709373450035 ) ) ;
#10262=AXIS2_PLACEMENT_3D ( 'NONE', #7450, #2432, #4890 ) ;
#10263=CARTESIAN_POINT ( 'NONE',  ( -19.39806930854668465, 4.049999998907525267, 19.39806930854667755 ) ) ;
#10264=ORIENTED_EDGE ( 'NONE', *, *, #2448, .F. ) ;
#10266=CARTESIAN_POINT ( 'NONE',  ( 3.764204346677844093, 100.0000000000000142, -22.52576385118515745 ) ) ;
#10268=CARTESIAN_POINT ( 'NONE',  ( 4.829054701479813083, 99.50000000000000000, -23.91032069601275367 ) ) ;
#10269=CARTESIAN_POINT ( 'NONE',  ( 1.679787559701184688E-15, 3.749999998907525445, -27.43301270000000258 ) ) ;
#10271=CARTESIAN_POINT ( 'NONE',  ( -15.30604604128650692, 99.99999999999997158, 15.41317891555018349 ) ) ;
#10273=CARTESIAN_POINT ( 'NONE',  ( -16.56928979259283352, 99.50000000000002842, 16.65656195153832897 ) ) ;
#10274=CARTESIAN_POINT ( 'NONE',  ( 11.18376618407357626, 3.850000000000000089, 27.00000000000000000 ) ) ;
#10276=CARTESIAN_POINT ( 'NONE',  ( 3.712044765110731337, 99.49999999999998579, -21.08683700305641651 ) ) ;
#10277=ORIENTED_EDGE ( 'NONE', *, *, #7602, .F. ) ;
#10278=VERTEX_POINT ( 'NONE', #2180 ) ;
#10281=CARTESIAN_POINT ( 'NONE',  ( -27.43301270000000258, 1.549999998907525267, -3.359575119402369376E-15 ) ) ;
#10282=CARTESIAN_POINT ( 'NONE',  ( 3.681717055787076642, 99.50000000000000000, -21.09125273517263111 ) ) ;
#10283=FACE_OUTER_BOUND ( 'NONE', #2315, .T. ) ;
#10284=CARTESIAN_POINT ( 'NONE',  ( 9.245739950628269810, 99.50000000000002842, 20.03726560014620617 ) ) ;
#10285=ORIENTED_EDGE ( 'NONE', *, *, #3357, .F. ) ;
#10286=CARTESIAN_POINT ( 'NONE',  ( -16.56313167360273297, 99.99999999999998579, 16.06491815633068398 ) ) ;
#10287=CARTESIAN_POINT ( 'NONE',  ( 8.337740814200648387, 100.0000000000000284, 20.10843643765939248 ) ) ;
#10289=EDGE_LOOP ( 'NONE', ( #6164, #2635, #6864, #8774 ) ) ;
#10291=CARTESIAN_POINT ( 'NONE',  ( -27.43301270000000258, 2.999999998907525445, -11.36312591709336317 ) ) ;
#10293=B_SPLINE_SURFACE_WITH_KNOTS ( 'NONE', 3, 1, ( 
 ( #7670, #561 ),
 ( #6045, #398 ),
 ( #2125, #7143 ),
 ( #10024, #3701 ),
 ( #1182, #6883 ),
 ( #5325, #9975 ),
 ( #2916, #8515 ),
 ( #1343, #2859 ),
 ( #7559, #4530 ),
 ( #7727, #1544 ),
 ( #5995, #3179 ),
 ( #3754, #9234 ),
 ( #9186, #10140 ),
 ( #2066, #2977 ),
 ( #6158, #9354 ) ),
 .UNSPECIFIED., .F., .F., .F.,
 ( 4, 1, 1, 1, 1, 1, 1, 1, 1, 1, 1, 1, 4 ),
 ( 2, 2 ),
 ( 0.000000000000000000, 0.09895296010982183865, 0.1966578232739713550, 0.2939931048315790330, 0.3929322324600736938, 0.4463669803336778319, 0.5055752425223922764, 0.5715235163887821823, 0.6440401046887170855, 0.7229629404452876384, 0.8087840669208056221, 0.9009145765370688563, 1.000000000000000000 ),
 ( 0.000000000000000000, 1.000000000000000000 ),
 .UNSPECIFIED. ) ;
#10295=CARTESIAN_POINT ( 'NONE',  ( -16.52319226728147328, 99.99999999999998579, 15.63609008536095324 ) ) ;
#10298=EDGE_LOOP ( 'NONE', ( #9451, #5155, #3515, #5700 ) ) ;
#10300=ADVANCED_FACE ( 'NONE', ( #763 ), #7723, .T. ) ;
#10301=CARTESIAN_POINT ( 'NONE',  ( 4.835062408351179286, 100.0000000000000000, -21.79588013901878440 ) ) ;
#10302=CARTESIAN_POINT ( 'NONE',  ( -15.24337324910153946, 99.99999999999997158, 16.81353386054630761 ) ) ;
#10306=LINE ( 'NONE', #2299, #7198 ) ;
#10308=CARTESIAN_POINT ( 'NONE',  ( -17.94007301623892658, 99.50000000000000000, 17.49000340848992607 ) ) ;
#10309=CARTESIAN_POINT ( 'NONE',  ( -19.39806930854667755, 4.649999998907525800, -19.39806930854668110 ) ) ;
#10310=EDGE_LOOP ( 'NONE', ( #7436, #2855, #5362, #10109, #9437, #1643, #9608, #73, #7696, #3118, #2550, #4333, #2912, #1589, #623, #4754, #3516 ) ) ;
#10314=CARTESIAN_POINT ( 'NONE',  ( -20.93575003794465061, 100.0000000000000142, -10.12220034237898503 ) ) ;
#10316=CARTESIAN_POINT ( 'NONE',  ( -21.12798922145720582, 99.50000000000001421, -10.90888695829967325 ) ) ;
#10317=CARTESIAN_POINT ( 'NONE',  ( 11.36312591709336850, 4.999999998907526333, 27.43301269999999903 ) ) ;
#10318=CARTESIAN_POINT ( 'NONE',  ( 6.246869686064662197, 99.50000000000000000, 20.92172973853146090 ) ) ;
#10319=B_SPLINE_CURVE_WITH_KNOTS ( 'NONE', 3,
 ( #530, #2939, #9317, #6906, #10273, #2204, #7752 ),
 .UNSPECIFIED., .F., .F.,
 ( 4, 1, 1, 1, 4 ),
 ( 0.000000000000000000, 0.2687002788711734813, 0.5225003893189538173, 0.7676814173175746658, 1.000000000000000000 ),
 .UNSPECIFIED. ) ;
#10320=CARTESIAN_POINT ( 'NONE',  ( 3.664124300404482337, 100.0000000000000284, -24.27219056640880623 ) ) ;
#10322=ADVANCED_FACE ( 'NONE', ( #1646 ), #9649, .T. ) ;
#10326=CARTESIAN_POINT ( 'NONE',  ( -21.39817337045129619, 99.50000000000001421, -9.317726141196148504 ) ) ;
#10328=EDGE_LOOP ( 'NONE', ( #424, #6968, #3684, #9188 ) ) ;
#10330=CARTESIAN_POINT ( 'NONE',  ( -27.43301270000000258, 4.599999998907525978, -11.36312591709336317 ) ) ;
#10333=CARTESIAN_POINT ( 'NONE',  ( 19.39806930854668110, 1.149999998907525356, -19.39806930854668110 ) ) ;
#10337=DIRECTION ( 'NONE',  ( -0.000000000000000000, 1.000000000000000000, -0.000000000000000000 ) ) ;
#10338=CARTESIAN_POINT ( 'NONE',  ( 8.149445629999579666, 100.0000000000000284, 20.33980848884064230 ) ) ;
#10339=( BOUNDED_CURVE ( )  B_SPLINE_CURVE ( 2, ( #6290, #10274, #6342, #2413, #9537, #7859, #5558, #1626, #1574 ),
 .UNSPECIFIED., .F., .T. ) 
 B_SPLINE_CURVE_WITH_KNOTS ( ( 3, 2, 2, 2, 3 ),
 ( 0.6785714285714286031, 0.6964285714285713969, 0.7142857142857143016, 0.7321428571428570953, 0.7500000000000000000 ),
 .UNSPECIFIED. ) 
 CURVE ( )  GEOMETRIC_REPRESENTATION_ITEM ( )  RATIONAL_B_SPLINE_CURVE ( ( 1.000000000000000000, 0.9238795325112867385, 1.000000000000000000, 0.9238795325112867385, 1.000000000000000000, 0.9238795325112867385, 1.000000000000000000, 0.9238795325112867385, 1.000000000000000000 ) ) 
 REPRESENTATION_ITEM ( '' )  );
#10342=CARTESIAN_POINT ( 'NONE',  ( 27.43301270000000258, 3.449999998907525178, 0.000000000000000000 ) ) ;
#10343=CARTESIAN_POINT ( 'NONE',  ( 4.135809822336132591, 99.99999999999998579, -24.70305975188825443 ) ) ;
#10347=CARTESIAN_POINT ( 'NONE',  ( 3.079986699855593473E-15, 100.0000000000000000, 25.15000000000000213 ) ) ;
#10348=CARTESIAN_POINT ( 'NONE',  ( -16.70213339477928471, 99.49999999999998579, 16.52464093453885852 ) ) ;
#10356=ADVANCED_FACE ( 'NONE', ( #7929 ), #762, .T. ) ;
#10357=ORIENTED_EDGE ( 'NONE', *, *, #531, .F. ) ;
#10358=CARTESIAN_POINT ( 'NONE',  ( 2.928963527206765338, 99.49999999999997158, -23.52685633767685758 ) ) ;
#10359=ORIENTED_EDGE ( 'NONE', *, *, #4869, .T. ) ;
#10360=CYLINDRICAL_SURFACE ( 'NONE', #1116, 18.00000000000000000 ) ;
#10362=B_SPLINE_CURVE_WITH_KNOTS ( 'NONE', 3,
 ( #9711, #7396, #7253, #94, #5696, #1950, #7550, #700, #9446, #9129, #2218, #4680, #3583, #7820, #8610, #2955, #7496, #6304, #9389 ),
 .UNSPECIFIED., .F., .F.,
 ( 4, 1, 1, 1, 1, 1, 1, 1, 1, 1, 1, 1, 1, 1, 1, 1, 4 ),
 ( 0.000000000000000000, 0.06473908249738200005, 0.1274869542813800993, 0.1888754624962200035, 0.2498352098569301405, 0.3101749858420705941, 0.3718734486855839183, 0.4342313324889700565, 0.4990836447755341299, 0.5639614065304963120, 0.6264045329497629488, 0.6882484937299673255, 0.7493615009078817835, 0.8100377551054726011, 0.8717391907241844873, 0.9348513958286107650, 1.000000000000000000 ),
 .UNSPECIFIED. ) ;
#10363=CARTESIAN_POINT ( 'NONE',  ( 7.826802610544922878, 99.50000000000000000, 21.21129867192371421 ) ) ;
#10364=CARTESIAN_POINT ( 'NONE',  ( -19.39806930854668465, 3.249999998907525001, 19.39806930854667755 ) ) ;
#10366=CARTESIAN_POINT ( 'NONE',  ( -15.76250887235353737, 99.49999999999998579, 16.65066592061022277 ) ) ;
#10381=COLOUR_RGB('Light Blue',0.38,0.62,0.78);
#10382=FILL_AREA_STYLE_COLOUR('',#10381);
#10383=FILL_AREA_STYLE('',(#10382));
#10384=SURFACE_STYLE_FILL_AREA(#10383);
#10385=SURFACE_SIDE_STYLE('',(#10384));
#10386=SURFACE_STYLE_USAGE(.BOTH.,#10385);
#10387=PRESENTATION_STYLE_ASSIGNMENT((#10386));
ENDSEC;
END-ISO-10303-21;
